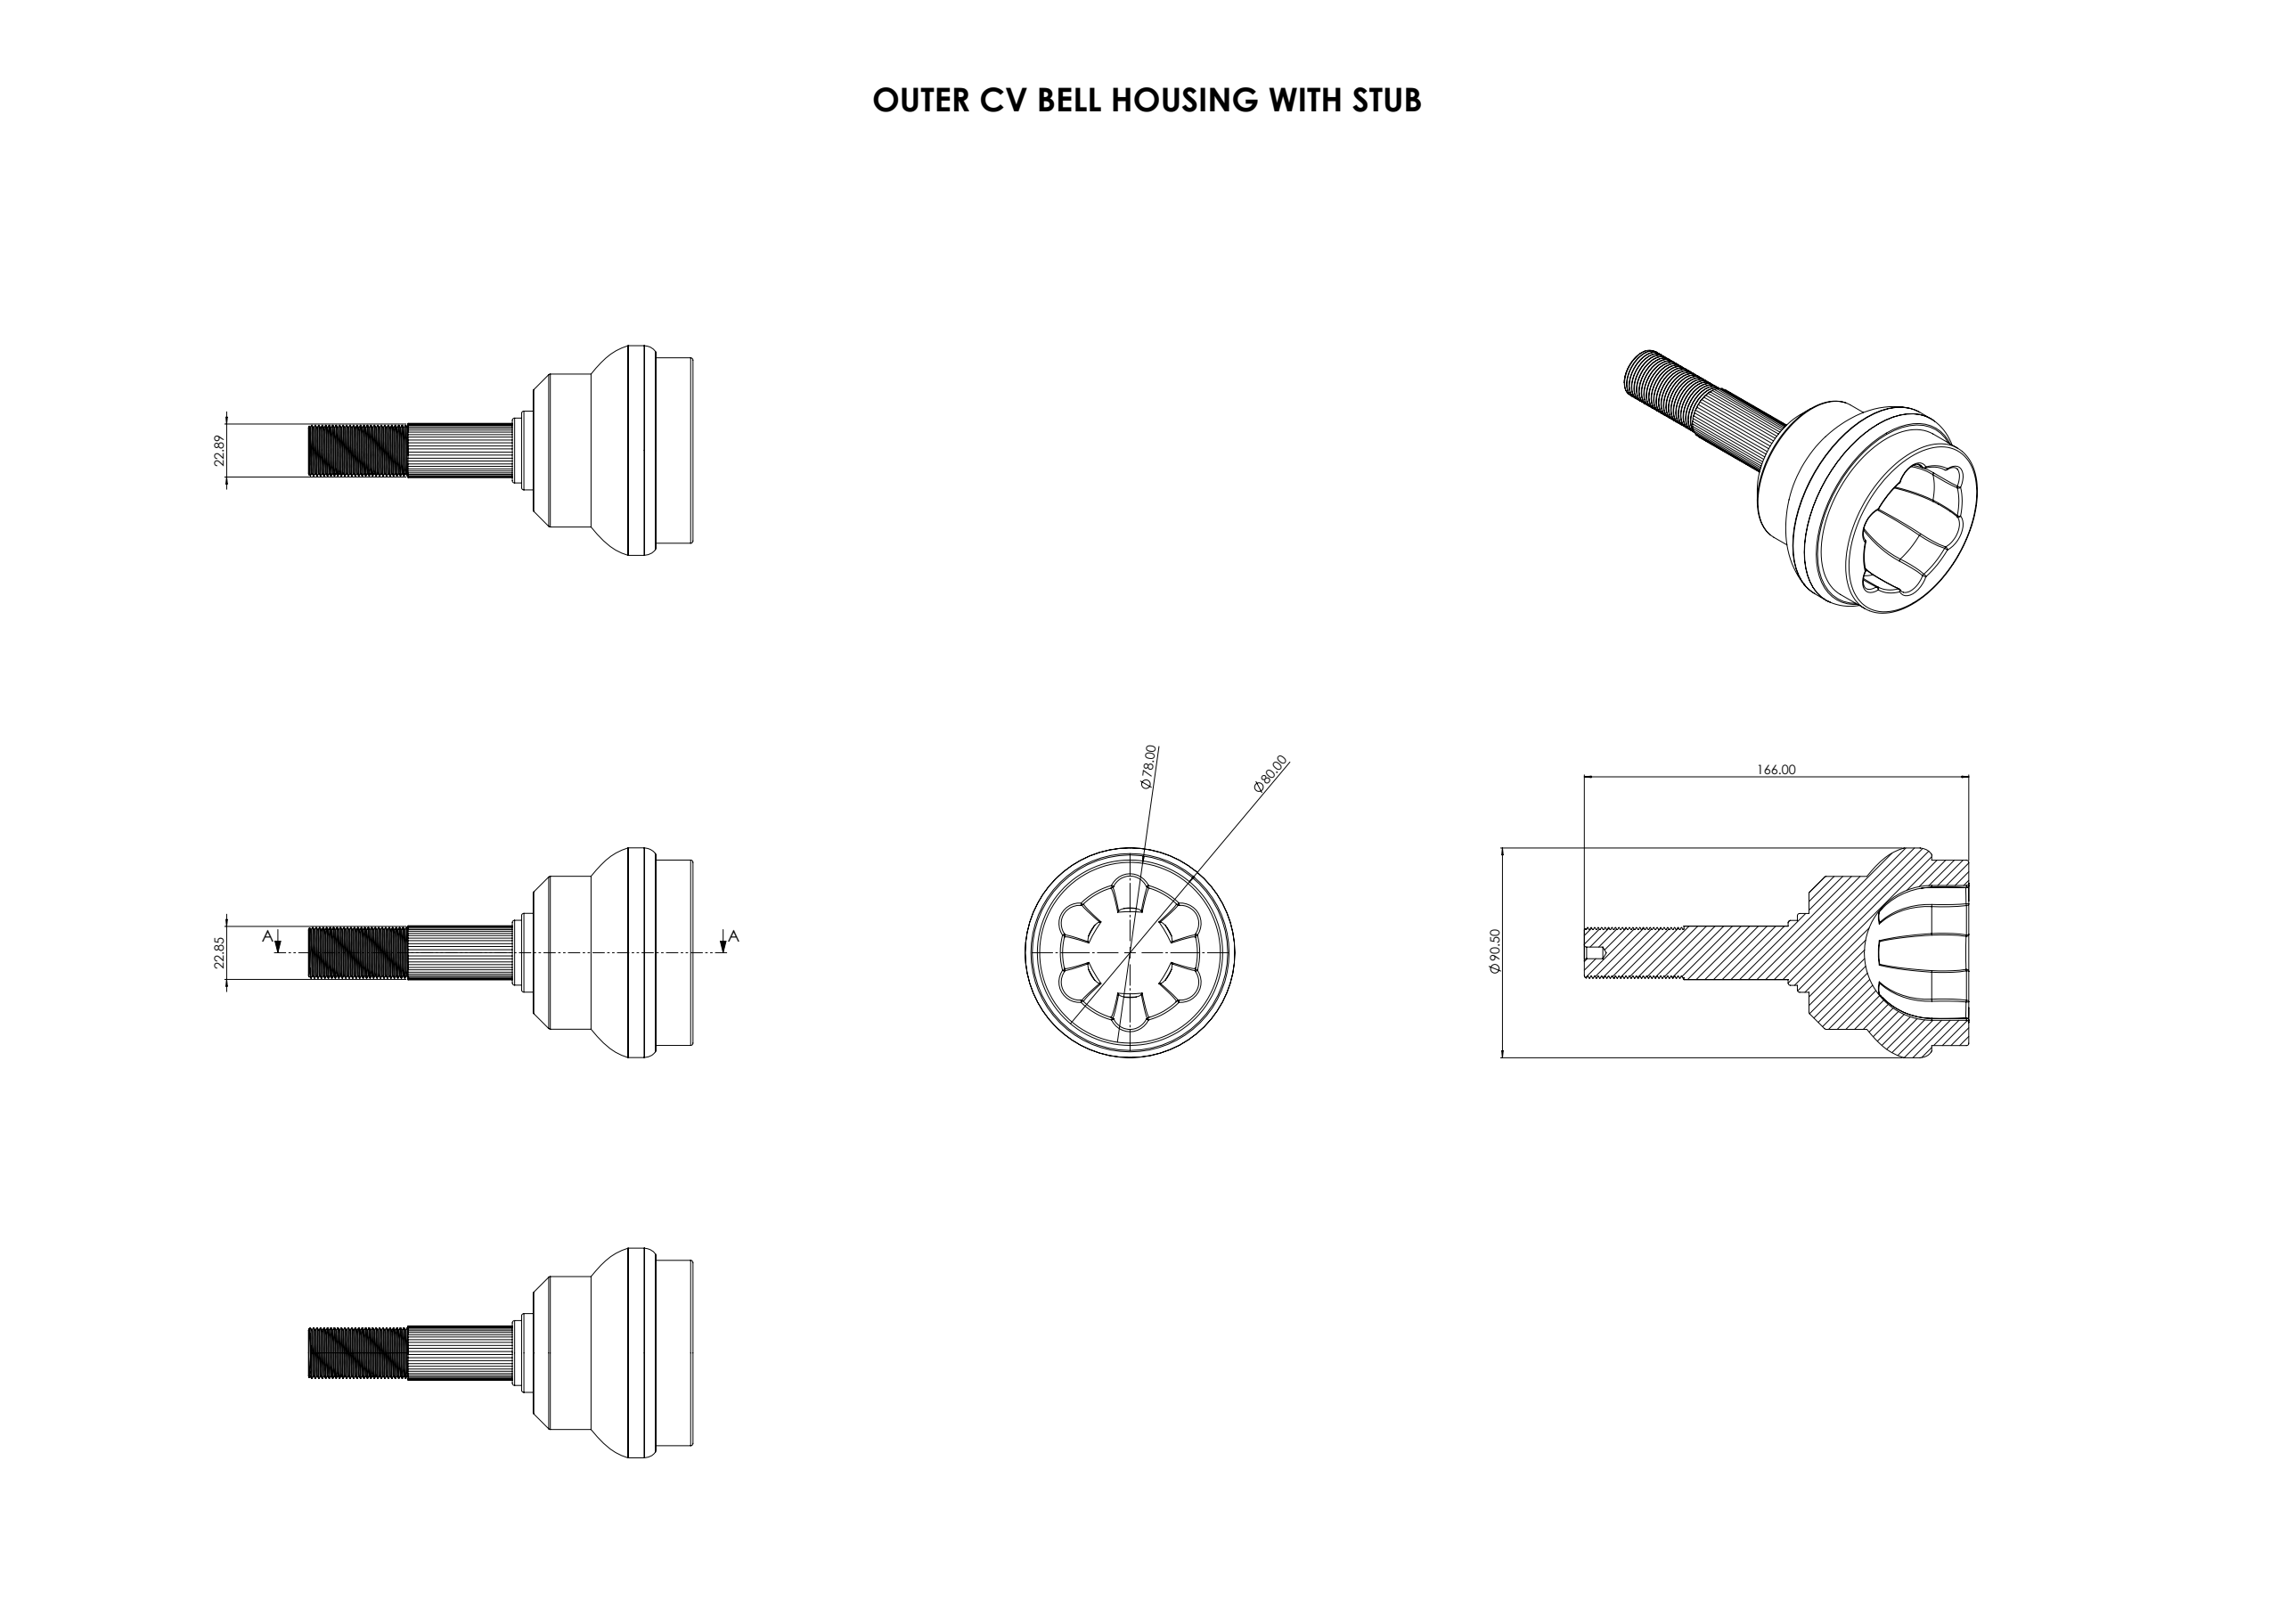
ISO-10303-21;
HEADER;
/* Generated by software containing ST-Developer
 * from STEP Tools, Inc. (www.steptools.com) 
 */

FILE_DESCRIPTION(
/* description */ (''),
/* implementation_level */ '2;1');

FILE_NAME(
/* name */ '01_Outer_CV_Bell_Housing_with_Stub.step',
/* time_stamp */ '2026-10-11T12:57:03-07:00',
/* author */ (''),
/* organization */ (''),
/* preprocessor_version */ 'ST-DEVELOPER v20.2',
/* originating_system */ 'Autodesk Translation Framework v15.15.0.0',
/* authorisation */ '');

FILE_SCHEMA (('AUTOMOTIVE_DESIGN { 1 0 10303 214 3 1 1 }'));
ENDSEC;

DATA;
#10=MECHANICAL_DESIGN_GEOMETRIC_PRESENTATION_REPRESENTATION('',(#256),#90374);
#222=SHAPE_REPRESENTATION_RELATIONSHIP('SRR','None',#90441,#239);
#239=ADVANCED_BREP_SHAPE_REPRESENTATION('',(#273),#90357);
#256=STYLED_ITEM('',(#90666),#273);
#273=MANIFOLD_SOLID_BREP('Body1',#40345);
#290=SPHERICAL_SURFACE('',#40682,1.);
#291=SPHERICAL_SURFACE('',#40693,1.);
#292=SPHERICAL_SURFACE('',#40696,1.);
#293=SPHERICAL_SURFACE('',#40706,1.);
#294=SPHERICAL_SURFACE('',#40722,1.);
#295=SPHERICAL_SURFACE('',#40737,1.);
#296=SPHERICAL_SURFACE('',#40746,1.);
#297=SPHERICAL_SURFACE('',#40754,1.);
#298=SPHERICAL_SURFACE('',#40760,1.);
#299=SPHERICAL_SURFACE('',#40771,1.);
#300=SPHERICAL_SURFACE('',#40778,1.);
#301=SPHERICAL_SURFACE('',#40783,1.);
#574=CONICAL_SURFACE('',#40627,29.5,0.785398163397447);
#575=CONICAL_SURFACE('',#40851,10.6,0.785398163397449);
#576=CONICAL_SURFACE('',#40869,2.5,1.03037682652431);
#781=TOROIDAL_SURFACE('',#40621,32.,1.);
#782=TOROIDAL_SURFACE('',#40631,25.5857864376269,1.);
#783=TOROIDAL_SURFACE('',#40636,16.,1.);
#784=TOROIDAL_SURFACE('',#40644,13.,1.);
#785=TOROIDAL_SURFACE('',#40685,26.4764045897475,8.05);
#786=TOROIDAL_SURFACE('',#40688,30.1,1.);
#787=TOROIDAL_SURFACE('',#40727,30.1,1.);
#788=TOROIDAL_SURFACE('',#40735,26.4764045897475,8.05);
#789=TOROIDAL_SURFACE('',#40740,30.1,1.);
#790=TOROIDAL_SURFACE('',#40748,26.4764045897475,8.05);
#791=TOROIDAL_SURFACE('',#40765,26.4764045897475,8.05);
#792=TOROIDAL_SURFACE('',#40766,30.1,1.);
#793=TOROIDAL_SURFACE('',#40773,26.4764045897475,8.05);
#794=TOROIDAL_SURFACE('',#40781,30.1,1.);
#795=TOROIDAL_SURFACE('',#40788,30.1,1.);
#796=TOROIDAL_SURFACE('',#40792,39.,1.);
#797=TOROIDAL_SURFACE('',#40849,9.925,1.);
#798=TOROIDAL_SURFACE('',#40857,9.78578643762691,1.);
#799=TOROIDAL_SURFACE('',#40863,3.5,1.);
#800=TOROIDAL_SURFACE('',#40899,26.4764045897475,8.05);
#1040=FACE_BOUND('',#4602,.T.);
#1041=FACE_BOUND('',#4612,.T.);
#1042=FACE_BOUND('',#4615,.T.);
#1043=FACE_BOUND('',#4619,.T.);
#1044=FACE_BOUND('',#4649,.T.);
#1045=FACE_BOUND('',#4695,.T.);
#1046=FACE_BOUND('',#4727,.T.);
#1116=PLANE('',#40614);
#1117=PLANE('',#40634);
#1118=PLANE('',#40641);
#1119=PLANE('',#40649);
#1120=PLANE('',#40678);
#1121=PLANE('',#40687);
#1122=PLANE('',#40729);
#1123=PLANE('',#40775);
#1124=PLANE('',#40799);
#1125=PLANE('',#40860);
#1126=PLANE('',#40870);
#1127=PLANE('',#40871);
#1128=PLANE('',#40872);
#1129=PLANE('',#40873);
#1130=PLANE('',#40874);
#1131=PLANE('',#40875);
#1132=PLANE('',#40876);
#1133=PLANE('',#40877);
#1134=PLANE('',#40878);
#1135=PLANE('',#40879);
#1136=PLANE('',#40880);
#1137=PLANE('',#40881);
#1138=PLANE('',#40882);
#1139=PLANE('',#40883);
#1140=PLANE('',#40884);
#1141=PLANE('',#40885);
#1142=PLANE('',#40886);
#1143=PLANE('',#40887);
#1144=PLANE('',#40888);
#1145=PLANE('',#40889);
#1146=PLANE('',#40890);
#1147=PLANE('',#40891);
#1148=PLANE('',#40892);
#1149=PLANE('',#40893);
#1150=PLANE('',#40894);
#1151=PLANE('',#40895);
#1152=PLANE('',#40896);
#1153=PLANE('',#40897);
#1154=PLANE('',#40901);
#1155=PLANE('',#40902);
#1828=(
BOUNDED_CURVE()
B_SPLINE_CURVE(5,(#61045,#61046,#61047,#61048,#61049,#61050,#61051,#61052,
#61053,#61054,#61055,#61056,#61057,#61058,#61059),.UNSPECIFIED.,.F.,.F.)
B_SPLINE_CURVE_WITH_KNOTS((6,1,1,1,1,1,1,1,1,1,6),(0.00785753170805376,
0.1,0.2,0.3,0.4,0.5,0.6,0.7,0.8,0.9,0.941278588050272),.UNSPECIFIED.)
CURVE()
GEOMETRIC_REPRESENTATION_ITEM()
RATIONAL_B_SPLINE_CURVE((1.,1.,1.,1.,1.,1.,1.,1.,1.,1.,1.,1.,1.,1.,1.))
REPRESENTATION_ITEM('')
);
#1829=(
BOUNDED_CURVE()
B_SPLINE_CURVE(5,(#61575,#61576,#61577,#61578,#61579,#61580,#61581,#61582,
#61583,#61584,#61585,#61586,#61587,#61588,#61589,#61590,#61591,#61592,#61593,
#61594),.UNSPECIFIED.,.F.,.F.)
B_SPLINE_CURVE_WITH_KNOTS((6,1,1,1,1,1,1,1,1,1,1,1,1,1,1,6),(0.,0.0666666666666667,
0.133333333333333,0.2,0.266666666666667,0.333333333333333,0.4,0.466666666666667,
0.533333333333333,0.6,0.666666666666667,0.733333333333333,0.8,0.866666666666667,
0.933333333333333,0.992729019266749),.UNSPECIFIED.)
CURVE()
GEOMETRIC_REPRESENTATION_ITEM()
RATIONAL_B_SPLINE_CURVE((1.,1.,1.,1.,1.,1.,1.,1.,1.,1.,1.,1.,1.,1.,1.,1.,
1.,1.,1.,1.))
REPRESENTATION_ITEM('')
);
#1931=(
BOUNDED_SURFACE()
B_SPLINE_SURFACE(5,2,((#60909,#60910,#60911,#60912,#60913,#60914,#60915,
#60916,#60917),(#60918,#60919,#60920,#60921,#60922,#60923,#60924,#60925,
#60926),(#60927,#60928,#60929,#60930,#60931,#60932,#60933,#60934,#60935),
(#60936,#60937,#60938,#60939,#60940,#60941,#60942,#60943,#60944),(#60945,
#60946,#60947,#60948,#60949,#60950,#60951,#60952,#60953),(#60954,#60955,
#60956,#60957,#60958,#60959,#60960,#60961,#60962),(#60963,#60964,#60965,
#60966,#60967,#60968,#60969,#60970,#60971),(#60972,#60973,#60974,#60975,
#60976,#60977,#60978,#60979,#60980),(#60981,#60982,#60983,#60984,#60985,
#60986,#60987,#60988,#60989),(#60990,#60991,#60992,#60993,#60994,#60995,
#60996,#60997,#60998),(#60999,#61000,#61001,#61002,#61003,#61004,#61005,
#61006,#61007),(#61008,#61009,#61010,#61011,#61012,#61013,#61014,#61015,
#61016),(#61017,#61018,#61019,#61020,#61021,#61022,#61023,#61024,#61025),
(#61026,#61027,#61028,#61029,#61030,#61031,#61032,#61033,#61034),(#61035,
#61036,#61037,#61038,#61039,#61040,#61041,#61042,#61043)),.UNSPECIFIED.,
 .F.,.T.,.F.)
B_SPLINE_SURFACE_WITH_KNOTS((6,1,1,1,1,1,1,1,1,1,6),(3,2,2,2,3),(-1.,-0.9,
-0.8,-0.7,-0.6,-0.5,-0.4,-0.3,-0.2,-0.1,0.),(0.,1.5707963267949,3.14159265358979,
4.71238898038469,6.28318530717959),.UNSPECIFIED.)
GEOMETRIC_REPRESENTATION_ITEM()
RATIONAL_B_SPLINE_SURFACE(((1.,0.707106781186548,1.,0.707106781186548,1.,
0.707106781186548,1.,0.707106781186548,1.),(1.,0.707106781186548,1.,0.707106781186548,
1.,0.707106781186548,1.,0.707106781186548,1.),(1.,0.707106781186548,1.,
0.707106781186548,1.,0.707106781186548,1.,0.707106781186548,1.),(1.,0.707106781186548,
1.,0.707106781186548,1.,0.707106781186548,1.,0.707106781186548,1.),(1.,
0.707106781186548,1.,0.707106781186548,1.,0.707106781186548,1.,0.707106781186548,
1.),(1.,0.707106781186548,1.,0.707106781186548,1.,0.707106781186548,1.,
0.707106781186548,1.),(1.,0.707106781186548,1.,0.707106781186548,1.,0.707106781186548,
1.,0.707106781186548,1.),(1.,0.707106781186548,1.,0.707106781186548,1.,
0.707106781186548,1.,0.707106781186548,1.),(1.,0.707106781186548,1.,0.707106781186548,
1.,0.707106781186548,1.,0.707106781186548,1.),(1.,0.707106781186548,1.,
0.707106781186548,1.,0.707106781186548,1.,0.707106781186548,1.),(1.,0.707106781186548,
1.,0.707106781186548,1.,0.707106781186548,1.,0.707106781186548,1.),(1.,
0.707106781186548,1.,0.707106781186548,1.,0.707106781186548,1.,0.707106781186548,
1.),(1.,0.707106781186548,1.,0.707106781186548,1.,0.707106781186548,1.,
0.707106781186548,1.),(1.,0.707106781186548,1.,0.707106781186548,1.,0.707106781186548,
1.,0.707106781186548,1.),(1.,0.707106781186548,1.,0.707106781186548,1.,
0.707106781186548,1.,0.707106781186548,1.)))
REPRESENTATION_ITEM('')
SURFACE()
);
#1932=(
BOUNDED_SURFACE()
B_SPLINE_SURFACE(5,2,((#61394,#61395,#61396,#61397,#61398,#61399,#61400,
#61401,#61402),(#61403,#61404,#61405,#61406,#61407,#61408,#61409,#61410,
#61411),(#61412,#61413,#61414,#61415,#61416,#61417,#61418,#61419,#61420),
(#61421,#61422,#61423,#61424,#61425,#61426,#61427,#61428,#61429),(#61430,
#61431,#61432,#61433,#61434,#61435,#61436,#61437,#61438),(#61439,#61440,
#61441,#61442,#61443,#61444,#61445,#61446,#61447),(#61448,#61449,#61450,
#61451,#61452,#61453,#61454,#61455,#61456),(#61457,#61458,#61459,#61460,
#61461,#61462,#61463,#61464,#61465),(#61466,#61467,#61468,#61469,#61470,
#61471,#61472,#61473,#61474),(#61475,#61476,#61477,#61478,#61479,#61480,
#61481,#61482,#61483),(#61484,#61485,#61486,#61487,#61488,#61489,#61490,
#61491,#61492),(#61493,#61494,#61495,#61496,#61497,#61498,#61499,#61500,
#61501),(#61502,#61503,#61504,#61505,#61506,#61507,#61508,#61509,#61510),
(#61511,#61512,#61513,#61514,#61515,#61516,#61517,#61518,#61519),(#61520,
#61521,#61522,#61523,#61524,#61525,#61526,#61527,#61528),(#61529,#61530,
#61531,#61532,#61533,#61534,#61535,#61536,#61537),(#61538,#61539,#61540,
#61541,#61542,#61543,#61544,#61545,#61546),(#61547,#61548,#61549,#61550,
#61551,#61552,#61553,#61554,#61555),(#61556,#61557,#61558,#61559,#61560,
#61561,#61562,#61563,#61564),(#61565,#61566,#61567,#61568,#61569,#61570,
#61571,#61572,#61573)),.UNSPECIFIED.,.F.,.T.,.F.)
B_SPLINE_SURFACE_WITH_KNOTS((6,1,1,1,1,1,1,1,1,1,1,1,1,1,1,6),(3,2,2,2,
3),(-1.,-0.933333333333333,-0.866666666666667,-0.8,-0.733333333333333,-0.666666666666667,
-0.6,-0.533333333333333,-0.466666666666667,-0.4,-0.333333333333333,-0.266666666666667,
-0.2,-0.133333333333333,-0.0666666666666667,0.),(0.,1.5707963267949,3.14159265358979,
4.71238898038469,6.28318530717959),.UNSPECIFIED.)
GEOMETRIC_REPRESENTATION_ITEM()
RATIONAL_B_SPLINE_SURFACE(((1.,0.707106781186548,1.,0.707106781186548,1.,
0.707106781186548,1.,0.707106781186548,1.),(1.,0.707106781186548,1.,0.707106781186548,
1.,0.707106781186548,1.,0.707106781186548,1.),(1.,0.707106781186548,1.,
0.707106781186548,1.,0.707106781186548,1.,0.707106781186548,1.),(1.,0.707106781186548,
1.,0.707106781186548,1.,0.707106781186548,1.,0.707106781186548,1.),(1.,
0.707106781186548,1.,0.707106781186548,1.,0.707106781186548,1.,0.707106781186548,
1.),(1.,0.707106781186548,1.,0.707106781186548,1.,0.707106781186548,1.,
0.707106781186548,1.),(1.,0.707106781186548,1.,0.707106781186548,1.,0.707106781186548,
1.,0.707106781186548,1.),(1.,0.707106781186548,1.,0.707106781186548,1.,
0.707106781186548,1.,0.707106781186548,1.),(1.,0.707106781186548,1.,0.707106781186548,
1.,0.707106781186548,1.,0.707106781186548,1.),(1.,0.707106781186548,1.,
0.707106781186548,1.,0.707106781186548,1.,0.707106781186548,1.),(1.,0.707106781186548,
1.,0.707106781186548,1.,0.707106781186548,1.,0.707106781186548,1.),(1.,
0.707106781186548,1.,0.707106781186548,1.,0.707106781186548,1.,0.707106781186548,
1.),(1.,0.707106781186548,1.,0.707106781186548,1.,0.707106781186548,1.,
0.707106781186548,1.),(1.,0.707106781186548,1.,0.707106781186548,1.,0.707106781186548,
1.,0.707106781186548,1.),(1.,0.707106781186548,1.,0.707106781186548,1.,
0.707106781186548,1.,0.707106781186548,1.),(1.,0.707106781186548,1.,0.707106781186548,
1.,0.707106781186548,1.,0.707106781186548,1.),(1.,0.707106781186548,1.,
0.707106781186548,1.,0.707106781186548,1.,0.707106781186548,1.),(1.,0.707106781186548,
1.,0.707106781186548,1.,0.707106781186548,1.,0.707106781186548,1.),(1.,
0.707106781186548,1.,0.707106781186548,1.,0.707106781186548,1.,0.707106781186548,
1.),(1.,0.707106781186548,1.,0.707106781186548,1.,0.707106781186548,1.,
0.707106781186548,1.)))
REPRESENTATION_ITEM('')
SURFACE()
);
#1933=(
BOUNDED_SURFACE()
B_SPLINE_SURFACE(2,2,((#62249,#62250,#62251,#62252,#62253,#62254,#62255,
#62256,#62257),(#62258,#62259,#62260,#62261,#62262,#62263,#62264,#62265,
#62266),(#62267,#62268,#62269,#62270,#62271,#62272,#62273,#62274,#62275)),
 .UNSPECIFIED.,.F.,.T.,.F.)
B_SPLINE_SURFACE_WITH_KNOTS((3,3),(3,2,2,2,3),(-1.5707731742648,-2.31493893392376E-5),
(-3.14159265358979,-1.5707963267949,0.,1.5707963267949,3.14159265358979),
 .UNSPECIFIED.)
GEOMETRIC_REPRESENTATION_ITEM()
RATIONAL_B_SPLINE_SURFACE(((1.,0.707106781186548,1.,0.707106781186548,1.,
0.707106781186548,1.,0.707106781186548,1.),(0.707123151197659,0.500011575345865,
0.707123151197659,0.500011575345865,0.707123151197659,0.500011575345865,
0.707123151197659,0.500011575345865,0.707123151197659),(1.,0.707106781186548,
1.,0.707106781186548,1.,0.707106781186548,1.,0.707106781186548,1.)))
REPRESENTATION_ITEM('')
SURFACE()
);
#1938=B_SPLINE_SURFACE_WITH_KNOTS('',3,3,((#60774,#60775,#60776,#60777,
#60778,#60779,#60780,#60781,#60782,#60783,#60784,#60785,#60786,#60787,#60788,
#60789,#60790,#60791,#60792,#60793,#60794,#60795),(#60796,#60797,#60798,
#60799,#60800,#60801,#60802,#60803,#60804,#60805,#60806,#60807,#60808,#60809,
#60810,#60811,#60812,#60813,#60814,#60815,#60816,#60817),(#60818,#60819,
#60820,#60821,#60822,#60823,#60824,#60825,#60826,#60827,#60828,#60829,#60830,
#60831,#60832,#60833,#60834,#60835,#60836,#60837,#60838,#60839),(#60840,
#60841,#60842,#60843,#60844,#60845,#60846,#60847,#60848,#60849,#60850,#60851,
#60852,#60853,#60854,#60855,#60856,#60857,#60858,#60859,#60860,#60861)),
 .UNSPECIFIED.,.F.,.T.,.F.,(4,4),(4,1,1,1,1,1,1,1,1,1,1,1,1,1,1,1,1,1,1,
4),(0.,1.),(1.5707963267949,2.01959527730772,2.46839422782055,2.76759352816244,
3.06679282850432,3.36599212884621,3.66519142918809,3.96439072952998,4.26359002987186,
4.56278933021375,4.86198863055563,5.16118793089752,5.4603872312394,5.75958653158129,
6.05878583192317,6.20838548209412,6.35798513226506,6.95638373294883,7.40518268346166,
7.85398163397448),.UNSPECIFIED.);
#1939=B_SPLINE_SURFACE_WITH_KNOTS('',3,3,((#61124,#61125,#61126,#61127,
#61128,#61129,#61130,#61131,#61132,#61133,#61134,#61135,#61136,#61137,#61138,
#61139,#61140,#61141,#61142,#61143,#61144,#61145,#61146),(#61147,#61148,
#61149,#61150,#61151,#61152,#61153,#61154,#61155,#61156,#61157,#61158,#61159,
#61160,#61161,#61162,#61163,#61164,#61165,#61166,#61167,#61168,#61169),
(#61170,#61171,#61172,#61173,#61174,#61175,#61176,#61177,#61178,#61179,
#61180,#61181,#61182,#61183,#61184,#61185,#61186,#61187,#61188,#61189,#61190,
#61191,#61192),(#61193,#61194,#61195,#61196,#61197,#61198,#61199,#61200,
#61201,#61202,#61203,#61204,#61205,#61206,#61207,#61208,#61209,#61210,#61211,
#61212,#61213,#61214,#61215)),.UNSPECIFIED.,.F.,.T.,.F.,(4,4),(4,1,1,1,
1,1,1,1,1,1,1,1,1,1,1,1,1,1,1,1,4),(0.,1.),(1.5707963267949,2.01959527730772,
2.46839422782055,2.76759352816244,3.06679282850432,3.36599212884621,3.66519142918809,
3.96439072952998,4.26359002987186,4.56278933021375,4.86198863055563,5.16118793089752,
5.4603872312394,5.75958653158129,6.05878583192317,6.20838548209412,6.35798513226506,
6.65718443260694,6.95638373294883,7.40518268346166,7.85398163397448),
 .UNSPECIFIED.);
#1940=B_SPLINE_SURFACE_WITH_KNOTS('',3,3,((#61277,#61278,#61279,#61280,
#61281,#61282,#61283,#61284,#61285,#61286,#61287,#61288,#61289,#61290,#61291,
#61292,#61293,#61294,#61295,#61296,#61297,#61298,#61299),(#61300,#61301,
#61302,#61303,#61304,#61305,#61306,#61307,#61308,#61309,#61310,#61311,#61312,
#61313,#61314,#61315,#61316,#61317,#61318,#61319,#61320,#61321,#61322),
(#61323,#61324,#61325,#61326,#61327,#61328,#61329,#61330,#61331,#61332,
#61333,#61334,#61335,#61336,#61337,#61338,#61339,#61340,#61341,#61342,#61343,
#61344,#61345),(#61346,#61347,#61348,#61349,#61350,#61351,#61352,#61353,
#61354,#61355,#61356,#61357,#61358,#61359,#61360,#61361,#61362,#61363,#61364,
#61365,#61366,#61367,#61368)),.UNSPECIFIED.,.F.,.T.,.F.,(4,4),(4,1,1,1,
1,1,1,1,1,1,1,1,1,1,1,1,1,1,1,1,4),(0.,1.),(1.5707963267949,2.01959527730772,
2.46839422782055,2.76759352816244,3.06679282850432,3.36599212884621,3.66519142918809,
3.96439072952998,4.26359002987186,4.56278933021375,4.86198863055563,5.16118793089752,
5.4603872312394,5.75958653158129,6.05878583192317,6.20838548209412,6.35798513226506,
6.65718443260694,6.95638373294883,7.40518268346166,7.85398163397448),
 .UNSPECIFIED.);
#1941=B_SPLINE_SURFACE_WITH_KNOTS('',3,3,((#61755,#61756,#61757,#61758),
(#61759,#61760,#61761,#61762),(#61763,#61764,#61765,#61766),(#61767,#61768,
#61769,#61770),(#61771,#61772,#61773,#61774)),.UNSPECIFIED.,.F.,.F.,.F.,
(4,1,4),(4,4),(0.,0.571428571428571,1.),(4.17539678580906,5.27137424194997),
 .UNSPECIFIED.);
#1942=B_SPLINE_SURFACE_WITH_KNOTS('',3,3,((#61821,#61822,#61823,#61824),
(#61825,#61826,#61827,#61828),(#61829,#61830,#61831,#61832),(#61833,#61834,
#61835,#61836),(#61837,#61838,#61839,#61840)),.UNSPECIFIED.,.F.,.F.,.F.,
(4,1,4),(4,4),(0.,0.571428571428571,1.),(4.17538600473639,5.27136346380212),
 .UNSPECIFIED.);
#1943=B_SPLINE_SURFACE_WITH_KNOTS('',3,3,((#61885,#61886,#61887,#61888,
#61889),(#61890,#61891,#61892,#61893,#61894),(#61895,#61896,#61897,#61898,
#61899),(#61900,#61901,#61902,#61903,#61904)),.UNSPECIFIED.,.F.,.F.,.F.,
(4,4),(4,1,4),(0.,1.),(8.38443833695044,9.5374231246245,11.0747361748566),
 .UNSPECIFIED.);
#1944=B_SPLINE_SURFACE_WITH_KNOTS('',3,3,((#61923,#61924,#61925,#61926,
#61927,#61928),(#61929,#61930,#61931,#61932,#61933,#61934),(#61935,#61936,
#61937,#61938,#61939,#61940),(#61941,#61942,#61943,#61944,#61945,#61946)),
 .UNSPECIFIED.,.F.,.F.,.F.,(4,4),(4,1,1,4),(0.,1.),(-2.31999627410953E-6,
0.644940971614267,1.07490316602129,1.50486536042832),.UNSPECIFIED.);
#1945=B_SPLINE_SURFACE_WITH_KNOTS('',3,3,((#62010,#62011,#62012,#62013,
#62014,#62015,#62016),(#62017,#62018,#62019,#62020,#62021,#62022,#62023),
(#62024,#62025,#62026,#62027,#62028,#62029,#62030),(#62031,#62032,#62033,
#62034,#62035,#62036,#62037),(#62038,#62039,#62040,#62041,#62042,#62043,
#62044),(#62045,#62046,#62047,#62048,#62049,#62050,#62051)),
 .UNSPECIFIED.,.F.,.F.,.F.,(4,1,1,4),(4,1,1,1,4),(0.,0.285714285714286,
0.571428571428571,1.),(3.95106839817899,4.52186525716006,4.8072636866506,
5.37806054563167,5.94885740461274),.UNSPECIFIED.);
#1946=B_SPLINE_SURFACE_WITH_KNOTS('',3,3,((#62135,#62136,#62137,#62138,
#62139,#62140),(#62141,#62142,#62143,#62144,#62145,#62146),(#62147,#62148,
#62149,#62150,#62151,#62152),(#62153,#62154,#62155,#62156,#62157,#62158)),
 .UNSPECIFIED.,.F.,.F.,.F.,(4,4),(4,1,1,4),(0.,1.),(-2.31999627050912E-6,
0.430022123191898,0.860046566380066,1.50508323116232),.UNSPECIFIED.);
#1947=B_SPLINE_SURFACE_WITH_KNOTS('',3,3,((#62182,#62183,#62184,#62185,
#62186),(#62187,#62188,#62189,#62190,#62191),(#62192,#62193,#62194,#62195,
#62196),(#62197,#62198,#62199,#62200,#62201)),.UNSPECIFIED.,.F.,.F.,.F.,
(4,4),(4,1,4),(0.,1.),(0.,0.644978914561078,1.50495080064252),
 .UNSPECIFIED.);
#1948=B_SPLINE_SURFACE_WITH_KNOTS('',3,3,((#62213,#62214,#62215,#62216,
#62217),(#62218,#62219,#62220,#62221,#62222),(#62223,#62224,#62225,#62226,
#62227),(#62228,#62229,#62230,#62231,#62232)),.UNSPECIFIED.,.F.,.F.,.F.,
(4,4),(4,1,4),(0.,1.),(-2.31999443863861E-6,1.15298346196168,2.69029783790316),
 .UNSPECIFIED.);
#1949=B_SPLINE_SURFACE_WITH_KNOTS('',3,3,((#62392,#62393,#62394,#62395),
(#62396,#62397,#62398,#62399),(#62400,#62401,#62402,#62403),(#62404,#62405,
#62406,#62407),(#62408,#62409,#62410,#62411)),.UNSPECIFIED.,.F.,.F.,.F.,
(4,1,4),(4,4),(0.,0.571428571428571,1.),(4.17539678580906,5.27137424194994),
 .UNSPECIFIED.);
#1950=B_SPLINE_SURFACE_WITH_KNOTS('',3,3,((#62452,#62453,#62454,#62455,
#62456,#62457,#62458),(#62459,#62460,#62461,#62462,#62463,#62464,#62465),
(#62466,#62467,#62468,#62469,#62470,#62471,#62472),(#62473,#62474,#62475,
#62476,#62477,#62478,#62479),(#62480,#62481,#62482,#62483,#62484,#62485,
#62486),(#62487,#62488,#62489,#62490,#62491,#62492,#62493)),
 .UNSPECIFIED.,.F.,.F.,.F.,(4,1,1,4),(4,1,1,1,4),(0.,0.285714285714286,
0.571428571428571,1.),(5.94885740461274,6.5196542639437,6.80505269360918,
7.37584955294014,7.9466464122711),.UNSPECIFIED.);
#1951=B_SPLINE_SURFACE_WITH_KNOTS('',3,3,((#62577,#62578,#62579,#62580,
#62581),(#62582,#62583,#62584,#62585,#62586),(#62587,#62588,#62589,#62590,
#62591),(#62592,#62593,#62594,#62595,#62596)),.UNSPECIFIED.,.F.,.F.,.F.,
(4,4),(4,1,4),(0.,1.),(0.206729096402498,0.851718551084393,1.71170449066025),
 .UNSPECIFIED.);
#1952=B_SPLINE_SURFACE_WITH_KNOTS('',3,3,((#62604,#62605,#62606,#62607,
#62608),(#62609,#62610,#62611,#62612,#62613),(#62614,#62615,#62616,#62617,
#62618),(#62619,#62620,#62621,#62622,#62623)),.UNSPECIFIED.,.F.,.F.,.F.,
(4,4),(4,1,4),(0.,1.),(-2.31999444043195E-6,1.15298346125989,2.69029783626566),
 .UNSPECIFIED.);
#1953=B_SPLINE_SURFACE_WITH_KNOTS('',3,3,((#62634,#62635,#62636,#62637,
#62638),(#62639,#62640,#62641,#62642,#62643),(#62644,#62645,#62646,#62647,
#62648),(#62649,#62650,#62651,#62652,#62653)),.UNSPECIFIED.,.F.,.F.,.F.,
(4,4),(4,1,4),(0.,1.),(8.52932428183543,9.68230906880774,11.2196221181042),
 .UNSPECIFIED.);
#1954=B_SPLINE_SURFACE_WITH_KNOTS('',3,3,((#62666,#62667,#62668,#62669,
#62670),(#62671,#62672,#62673,#62674,#62675),(#62676,#62677,#62678,#62679,
#62680),(#62681,#62682,#62683,#62684,#62685)),.UNSPECIFIED.,.F.,.F.,.F.,
(4,4),(4,1,4),(0.,1.),(-2.31999627648449E-6,0.85992278978735,1.50486662212507),
 .UNSPECIFIED.);
#1955=B_SPLINE_SURFACE_WITH_KNOTS('',3,3,((#63057,#63058,#63059,#63060),
(#63061,#63062,#63063,#63064),(#63065,#63066,#63067,#63068),(#63069,#63070,
#63071,#63072),(#63073,#63074,#63075,#63076)),.UNSPECIFIED.,.F.,.F.,.F.,
(4,1,4),(4,4),(0.,0.571428571428571,1.),(4.17533133480784,5.27130879387958),
 .UNSPECIFIED.);
#1956=B_SPLINE_SURFACE_WITH_KNOTS('',3,3,((#63115,#63116,#63117,#63118,
#63119),(#63120,#63121,#63122,#63123,#63124),(#63125,#63126,#63127,#63128,
#63129),(#63130,#63131,#63132,#63133,#63134)),.UNSPECIFIED.,.F.,.F.,.F.,
(4,4),(4,1,4),(0.,1.),(8.52985716994968,9.68284195691921,11.2201550062119),
 .UNSPECIFIED.);
#1957=B_SPLINE_SURFACE_WITH_KNOTS('',3,3,((#63153,#63154,#63155,#63156,
#63157,#63158),(#63159,#63160,#63161,#63162,#63163,#63164),(#63165,#63166,
#63167,#63168,#63169,#63170),(#63171,#63172,#63173,#63174,#63175,#63176)),
 .UNSPECIFIED.,.F.,.F.,.F.,(4,4),(4,1,1,4),(0.,1.),(0.207327684708445,0.637351476682114,
1.06737526865578,1.71241095661629),.UNSPECIFIED.);
#1958=B_SPLINE_SURFACE_WITH_KNOTS('',3,3,((#63191,#63192,#63193,#63194,
#63195),(#63196,#63197,#63198,#63199,#63200),(#63201,#63202,#63203,#63204,
#63205),(#63206,#63207,#63208,#63209,#63210)),.UNSPECIFIED.,.F.,.F.,.F.,
(4,4),(4,1,4),(0.,1.),(-2.31999443730624E-6,1.15298346125614,2.69029783625691),
 .UNSPECIFIED.);
#1959=B_SPLINE_SURFACE_WITH_KNOTS('',3,3,((#63221,#63222,#63223,#63224,
#63225,#63226),(#63227,#63228,#63229,#63230,#63231,#63232),(#63233,#63234,
#63235,#63236,#63237,#63238),(#63239,#63240,#63241,#63242,#63243,#63244)),
 .UNSPECIFIED.,.F.,.F.,.F.,(4,4),(4,1,1,4),(0.,1.),(0.,0.644950465905299,
1.0749174431755,1.5048844204457),.UNSPECIFIED.);
#1960=B_SPLINE_SURFACE_WITH_KNOTS('',3,3,((#63261,#63262,#63263,#63264,
#63265),(#63266,#63267,#63268,#63269,#63270),(#63271,#63272,#63273,#63274,
#63275),(#63276,#63277,#63278,#63279,#63280)),.UNSPECIFIED.,.F.,.F.,.F.,
(4,4),(4,1,4),(0.,1.),(-2.3199944317628E-6,1.15298346196206,2.69029783790404),
 .UNSPECIFIED.);
#1961=B_SPLINE_SURFACE_WITH_KNOTS('',3,3,((#63297,#63298,#63299,#63300,
#63301,#63302,#63303),(#63304,#63305,#63306,#63307,#63308,#63309,#63310),
(#63311,#63312,#63313,#63314,#63315,#63316,#63317),(#63318,#63319,#63320,
#63321,#63322,#63323,#63324),(#63325,#63326,#63327,#63328,#63329,#63330,
#63331),(#63332,#63333,#63334,#63335,#63336,#63337,#63338)),
 .UNSPECIFIED.,.F.,.F.,.F.,(4,1,1,4),(4,1,1,1,4),(0.,0.285714285714286,
0.571428571428571,1.),(4.94996091805913,5.2353622298247,5.80616485335585,
6.37696747688699,6.94777010041813),.UNSPECIFIED.);
#1962=B_SPLINE_SURFACE_WITH_KNOTS('',3,3,((#63348,#63349,#63350,#63351,
#63352),(#63353,#63354,#63355,#63356,#63357),(#63358,#63359,#63360,#63361,
#63362),(#63363,#63364,#63365,#63366,#63367)),.UNSPECIFIED.,.F.,.F.,.F.,
(4,4),(4,1,4),(0.,1.),(0.,0.85997188017068,1.50495079029869),
 .UNSPECIFIED.);
#1963=B_SPLINE_SURFACE_WITH_KNOTS('',3,3,((#63390,#63391,#63392,#63393,
#63394),(#63395,#63396,#63397,#63398,#63399),(#63400,#63401,#63402,#63403,
#63404),(#63405,#63406,#63407,#63408,#63409)),.UNSPECIFIED.,.F.,.F.,.F.,
(4,4),(4,1,4),(0.,1.),(8.38443833694999,9.92175271289341,11.074738494851),
 .UNSPECIFIED.);
#1964=B_SPLINE_SURFACE_WITH_KNOTS('',3,3,((#63434,#63435,#63436,#63437,
#63438),(#63439,#63440,#63441,#63442,#63443),(#63444,#63445,#63446,#63447,
#63448),(#63449,#63450,#63451,#63452,#63453)),.UNSPECIFIED.,.F.,.F.,.F.,
(4,4),(4,1,4),(0.,1.),(0.,0.644951640555328,1.50488716129577),
 .UNSPECIFIED.);
#1965=B_SPLINE_SURFACE_WITH_KNOTS('',3,3,((#63466,#63467,#63468,#63469,
#63470),(#63471,#63472,#63473,#63474,#63475),(#63476,#63477,#63478,#63479,
#63480),(#63481,#63482,#63483,#63484,#63485)),.UNSPECIFIED.,.F.,.F.,.F.,
(4,4),(4,1,4),(0.,1.),(-2.31999443914823E-6,1.15298346196168,2.69029783790317),
 .UNSPECIFIED.);
#1966=B_SPLINE_SURFACE_WITH_KNOTS('',3,3,((#63504,#63505,#63506,#63507,
#63508,#63509,#63510),(#63511,#63512,#63513,#63514,#63515,#63516,#63517),
(#63518,#63519,#63520,#63521,#63522,#63523,#63524),(#63525,#63526,#63527,
#63528,#63529,#63530,#63531),(#63532,#63533,#63534,#63535,#63536,#63537,
#63538),(#63539,#63540,#63541,#63542,#63543,#63544,#63545)),
 .UNSPECIFIED.,.F.,.F.,.F.,(4,1,1,4),(4,1,1,1,4),(0.,0.285714285714286,
0.571428571428571,1.),(4.94996091806794,5.52076354159657,6.09156616512519,
6.37696747688951,6.94777010041813),.UNSPECIFIED.);
#1967=B_SPLINE_SURFACE_WITH_KNOTS('',3,3,((#63550,#63551,#63552,#63553),
(#63554,#63555,#63556,#63557),(#63558,#63559,#63560,#63561),(#63562,#63563,
#63564,#63565),(#63566,#63567,#63568,#63569)),.UNSPECIFIED.,.F.,.F.,.F.,
(4,1,4),(4,4),(0.,0.571428571428571,1.),(4.17531192673851,5.2712893858124),
 .UNSPECIFIED.);
#1968=B_SPLINE_SURFACE_WITH_KNOTS('',3,3,((#63608,#63609,#63610,#63611,
#63612),(#63613,#63614,#63615,#63616,#63617),(#63618,#63619,#63620,#63621,
#63622),(#63623,#63624,#63625,#63626,#63627)),.UNSPECIFIED.,.F.,.F.,.F.,
(4,4),(4,1,4),(0.,1.),(8.38443833695038,9.53742312462444,11.0747361748565),
 .UNSPECIFIED.);
#1969=B_SPLINE_SURFACE_WITH_KNOTS('',3,3,((#63640,#63641,#63642,#63643,
#63644,#63645),(#63646,#63647,#63648,#63649,#63650,#63651),(#63652,#63653,
#63654,#63655,#63656,#63657),(#63658,#63659,#63660,#63661,#63662,#63663)),
 .UNSPECIFIED.,.F.,.F.,.F.,(4,4),(4,1,1,4),(0.,1.),(-2.3199962741138E-6,
0.644939523401962,1.07490075233412,1.50486198126628),.UNSPECIFIED.);
#1970=B_SPLINE_SURFACE_WITH_KNOTS('',3,3,((#63708,#63709,#63710,#63711,
#63712,#63713),(#63714,#63715,#63716,#63717,#63718,#63719),(#63720,#63721,
#63722,#63723,#63724,#63725),(#63726,#63727,#63728,#63729,#63730,#63731)),
 .UNSPECIFIED.,.F.,.F.,.F.,(4,4),(4,1,1,4),(0.,1.),(0.,0.429964410955918,
0.859928821911836,1.50487543834571),.UNSPECIFIED.);
#1971=B_SPLINE_SURFACE_WITH_KNOTS('',3,3,((#63741,#63742,#63743,#63744,
#63745),(#63746,#63747,#63748,#63749,#63750),(#63751,#63752,#63753,#63754,
#63755),(#63756,#63757,#63758,#63759,#63760)),.UNSPECIFIED.,.F.,.F.,.F.,
(4,4),(4,1,4),(0.,1.),(-2.31999443732384E-6,1.15298346196168,2.69029783790317),
 .UNSPECIFIED.);
#1972=B_SPLINE_SURFACE_WITH_KNOTS('',3,3,((#63764,#63765,#63766,#63767,
#63768,#63769,#63770),(#63771,#63772,#63773,#63774,#63775,#63776,#63777),
(#63778,#63779,#63780,#63781,#63782,#63783,#63784),(#63785,#63786,#63787,
#63788,#63789,#63790,#63791),(#63792,#63793,#63794,#63795,#63796,#63797,
#63798),(#63799,#63800,#63801,#63802,#63803,#63804,#63805)),
 .UNSPECIFIED.,.F.,.F.,.F.,(4,1,1,4),(4,1,1,1,4),(0.,0.285714285714286,
0.571428571428571,1.),(4.94996091805957,5.23536222982578,5.80616485335821,
6.37696747689064,6.94777010042307),.UNSPECIFIED.);
#1973=B_SPLINE_SURFACE_WITH_KNOTS('',3,3,((#63808,#63809,#63810,#63811,
#63812,#63813,#63814),(#63815,#63816,#63817,#63818,#63819,#63820,#63821),
(#63822,#63823,#63824,#63825,#63826,#63827,#63828),(#63829,#63830,#63831,
#63832,#63833,#63834,#63835),(#63836,#63837,#63838,#63839,#63840,#63841,
#63842),(#63843,#63844,#63845,#63846,#63847,#63848,#63849)),
 .UNSPECIFIED.,.F.,.F.,.F.,(4,1,1,4),(4,1,1,1,4),(0.,0.285714285714286,
0.571428571428571,1.),(4.94996091806794,5.23536222983225,5.80616485336088,
6.3769674768895,6.94777010041813),.UNSPECIFIED.);
#1974=B_SPLINE_SURFACE_WITH_KNOTS('',3,3,((#63860,#63861,#63862,#63863,
#63864),(#63865,#63866,#63867,#63868,#63869),(#63870,#63871,#63872,#63873,
#63874),(#63875,#63876,#63877,#63878,#63879)),.UNSPECIFIED.,.F.,.F.,.F.,
(4,4),(4,1,4),(0.,1.),(0.206737365090144,0.851711715694741,1.71167751650087),
 .UNSPECIFIED.);
#1975=B_SPLINE_SURFACE_WITH_KNOTS('',3,3,((#63895,#63896,#63897,#63898),
(#63899,#63900,#63901,#63902),(#63903,#63904,#63905,#63906),(#63907,#63908,
#63909,#63910),(#63911,#63912,#63913,#63914)),.UNSPECIFIED.,.F.,.F.,.F.,
(4,1,4),(4,4),(0.,0.571428571428571,1.),(4.17431363002051,5.27029108627002),
 .UNSPECIFIED.);
#1976=B_SPLINE_SURFACE_WITH_KNOTS('',3,3,((#63948,#63949,#63950,#63951,
#63952),(#63953,#63954,#63955,#63956,#63957),(#63958,#63959,#63960,#63961,
#63962),(#63963,#63964,#63965,#63966,#63967)),.UNSPECIFIED.,.F.,.F.,.F.,
(4,4),(4,1,4),(0.,1.),(-2.31999444274574E-6,1.15298346125989,2.69029783626567),
 .UNSPECIFIED.);
#1977=B_SPLINE_SURFACE_WITH_KNOTS('',3,3,((#64687,#64688,#64689,#64690,
#64691,#64692,#64693,#64694,#64695,#64696,#64697,#64698,#64699,#64700,#64701,
#64702,#64703,#64704,#64705,#64706,#64707,#64708,#64709,#64710,#64711,#64712,
#64713,#64714,#64715,#64716,#64717,#64718,#64719,#64720,#64721,#64722,#64723,
#64724,#64725,#64726,#64727,#64728,#64729,#64730,#64731,#64732,#64733,#64734,
#64735,#64736,#64737,#64738,#64739,#64740,#64741,#64742,#64743,#64744,#64745,
#64746,#64747,#64748,#64749,#64750,#64751,#64752,#64753,#64754,#64755,#64756,
#64757,#64758,#64759,#64760,#64761,#64762,#64763,#64764,#64765,#64766,#64767,
#64768,#64769,#64770,#64771,#64772,#64773,#64774,#64775,#64776,#64777,#64778,
#64779,#64780,#64781,#64782,#64783,#64784,#64785,#64786,#64787,#64788,#64789,
#64790,#64791,#64792,#64793,#64794,#64795,#64796,#64797,#64798,#64799,#64800,
#64801,#64802,#64803,#64804,#64805,#64806,#64807,#64808,#64809,#64810,#64811,
#64812,#64813,#64814,#64815,#64816,#64817,#64818,#64819,#64820,#64821,#64822,
#64823,#64824,#64825,#64826,#64827,#64828,#64829,#64830,#64831,#64832,#64833,
#64834,#64835,#64836,#64837,#64838,#64839,#64840,#64841,#64842,#64843,#64844,
#64845,#64846,#64847,#64848,#64849,#64850,#64851,#64852,#64853,#64854,#64855,
#64856,#64857,#64858,#64859,#64860,#64861,#64862,#64863,#64864,#64865,#64866,
#64867,#64868,#64869,#64870,#64871,#64872,#64873,#64874,#64875,#64876,#64877,
#64878,#64879,#64880,#64881,#64882,#64883,#64884,#64885,#64886,#64887,#64888,
#64889,#64890,#64891,#64892,#64893,#64894,#64895,#64896,#64897,#64898,#64899,
#64900,#64901,#64902,#64903,#64904,#64905,#64906,#64907,#64908,#64909,#64910,
#64911,#64912,#64913,#64914,#64915,#64916,#64917,#64918,#64919,#64920,#64921,
#64922,#64923,#64924,#64925,#64926,#64927,#64928,#64929,#64930,#64931,#64932,
#64933,#64934,#64935,#64936,#64937,#64938,#64939,#64940,#64941,#64942,#64943,
#64944,#64945,#64946,#64947,#64948,#64949,#64950,#64951,#64952,#64953,#64954,
#64955,#64956,#64957,#64958,#64959,#64960,#64961,#64962,#64963,#64964,#64965,
#64966,#64967,#64968,#64969,#64970,#64971,#64972,#64973,#64974,#64975,#64976,
#64977,#64978,#64979,#64980,#64981,#64982,#64983,#64984,#64985,#64986,#64987,
#64988,#64989,#64990,#64991,#64992,#64993,#64994,#64995,#64996,#64997,#64998,
#64999,#65000,#65001,#65002,#65003,#65004,#65005,#65006,#65007,#65008,#65009,
#65010,#65011,#65012,#65013,#65014,#65015,#65016,#65017,#65018,#65019,#65020,
#65021,#65022,#65023,#65024,#65025,#65026,#65027,#65028,#65029,#65030,#65031,
#65032,#65033,#65034,#65035,#65036,#65037,#65038,#65039,#65040,#65041,#65042,
#65043,#65044,#65045,#65046,#65047,#65048,#65049),(#65050,#65051,#65052,
#65053,#65054,#65055,#65056,#65057,#65058,#65059,#65060,#65061,#65062,#65063,
#65064,#65065,#65066,#65067,#65068,#65069,#65070,#65071,#65072,#65073,#65074,
#65075,#65076,#65077,#65078,#65079,#65080,#65081,#65082,#65083,#65084,#65085,
#65086,#65087,#65088,#65089,#65090,#65091,#65092,#65093,#65094,#65095,#65096,
#65097,#65098,#65099,#65100,#65101,#65102,#65103,#65104,#65105,#65106,#65107,
#65108,#65109,#65110,#65111,#65112,#65113,#65114,#65115,#65116,#65117,#65118,
#65119,#65120,#65121,#65122,#65123,#65124,#65125,#65126,#65127,#65128,#65129,
#65130,#65131,#65132,#65133,#65134,#65135,#65136,#65137,#65138,#65139,#65140,
#65141,#65142,#65143,#65144,#65145,#65146,#65147,#65148,#65149,#65150,#65151,
#65152,#65153,#65154,#65155,#65156,#65157,#65158,#65159,#65160,#65161,#65162,
#65163,#65164,#65165,#65166,#65167,#65168,#65169,#65170,#65171,#65172,#65173,
#65174,#65175,#65176,#65177,#65178,#65179,#65180,#65181,#65182,#65183,#65184,
#65185,#65186,#65187,#65188,#65189,#65190,#65191,#65192,#65193,#65194,#65195,
#65196,#65197,#65198,#65199,#65200,#65201,#65202,#65203,#65204,#65205,#65206,
#65207,#65208,#65209,#65210,#65211,#65212,#65213,#65214,#65215,#65216,#65217,
#65218,#65219,#65220,#65221,#65222,#65223,#65224,#65225,#65226,#65227,#65228,
#65229,#65230,#65231,#65232,#65233,#65234,#65235,#65236,#65237,#65238,#65239,
#65240,#65241,#65242,#65243,#65244,#65245,#65246,#65247,#65248,#65249,#65250,
#65251,#65252,#65253,#65254,#65255,#65256,#65257,#65258,#65259,#65260,#65261,
#65262,#65263,#65264,#65265,#65266,#65267,#65268,#65269,#65270,#65271,#65272,
#65273,#65274,#65275,#65276,#65277,#65278,#65279,#65280,#65281,#65282,#65283,
#65284,#65285,#65286,#65287,#65288,#65289,#65290,#65291,#65292,#65293,#65294,
#65295,#65296,#65297,#65298,#65299,#65300,#65301,#65302,#65303,#65304,#65305,
#65306,#65307,#65308,#65309,#65310,#65311,#65312,#65313,#65314,#65315,#65316,
#65317,#65318,#65319,#65320,#65321,#65322,#65323,#65324,#65325,#65326,#65327,
#65328,#65329,#65330,#65331,#65332,#65333,#65334,#65335,#65336,#65337,#65338,
#65339,#65340,#65341,#65342,#65343,#65344,#65345,#65346,#65347,#65348,#65349,
#65350,#65351,#65352,#65353,#65354,#65355,#65356,#65357,#65358,#65359,#65360,
#65361,#65362,#65363,#65364,#65365,#65366,#65367,#65368,#65369,#65370,#65371,
#65372,#65373,#65374,#65375,#65376,#65377,#65378,#65379,#65380,#65381,#65382,
#65383,#65384,#65385,#65386,#65387,#65388,#65389,#65390,#65391,#65392,#65393,
#65394,#65395,#65396,#65397,#65398,#65399,#65400,#65401,#65402,#65403,#65404,
#65405,#65406,#65407,#65408,#65409,#65410,#65411,#65412),(#65413,#65414,
#65415,#65416,#65417,#65418,#65419,#65420,#65421,#65422,#65423,#65424,#65425,
#65426,#65427,#65428,#65429,#65430,#65431,#65432,#65433,#65434,#65435,#65436,
#65437,#65438,#65439,#65440,#65441,#65442,#65443,#65444,#65445,#65446,#65447,
#65448,#65449,#65450,#65451,#65452,#65453,#65454,#65455,#65456,#65457,#65458,
#65459,#65460,#65461,#65462,#65463,#65464,#65465,#65466,#65467,#65468,#65469,
#65470,#65471,#65472,#65473,#65474,#65475,#65476,#65477,#65478,#65479,#65480,
#65481,#65482,#65483,#65484,#65485,#65486,#65487,#65488,#65489,#65490,#65491,
#65492,#65493,#65494,#65495,#65496,#65497,#65498,#65499,#65500,#65501,#65502,
#65503,#65504,#65505,#65506,#65507,#65508,#65509,#65510,#65511,#65512,#65513,
#65514,#65515,#65516,#65517,#65518,#65519,#65520,#65521,#65522,#65523,#65524,
#65525,#65526,#65527,#65528,#65529,#65530,#65531,#65532,#65533,#65534,#65535,
#65536,#65537,#65538,#65539,#65540,#65541,#65542,#65543,#65544,#65545,#65546,
#65547,#65548,#65549,#65550,#65551,#65552,#65553,#65554,#65555,#65556,#65557,
#65558,#65559,#65560,#65561,#65562,#65563,#65564,#65565,#65566,#65567,#65568,
#65569,#65570,#65571,#65572,#65573,#65574,#65575,#65576,#65577,#65578,#65579,
#65580,#65581,#65582,#65583,#65584,#65585,#65586,#65587,#65588,#65589,#65590,
#65591,#65592,#65593,#65594,#65595,#65596,#65597,#65598,#65599,#65600,#65601,
#65602,#65603,#65604,#65605,#65606,#65607,#65608,#65609,#65610,#65611,#65612,
#65613,#65614,#65615,#65616,#65617,#65618,#65619,#65620,#65621,#65622,#65623,
#65624,#65625,#65626,#65627,#65628,#65629,#65630,#65631,#65632,#65633,#65634,
#65635,#65636,#65637,#65638,#65639,#65640,#65641,#65642,#65643,#65644,#65645,
#65646,#65647,#65648,#65649,#65650,#65651,#65652,#65653,#65654,#65655,#65656,
#65657,#65658,#65659,#65660,#65661,#65662,#65663,#65664,#65665,#65666,#65667,
#65668,#65669,#65670,#65671,#65672,#65673,#65674,#65675,#65676,#65677,#65678,
#65679,#65680,#65681,#65682,#65683,#65684,#65685,#65686,#65687,#65688,#65689,
#65690,#65691,#65692,#65693,#65694,#65695,#65696,#65697,#65698,#65699,#65700,
#65701,#65702,#65703,#65704,#65705,#65706,#65707,#65708,#65709,#65710,#65711,
#65712,#65713,#65714,#65715,#65716,#65717,#65718,#65719,#65720,#65721,#65722,
#65723,#65724,#65725,#65726,#65727,#65728,#65729,#65730,#65731,#65732,#65733,
#65734,#65735,#65736,#65737,#65738,#65739,#65740,#65741,#65742,#65743,#65744,
#65745,#65746,#65747,#65748,#65749,#65750,#65751,#65752,#65753,#65754,#65755,
#65756,#65757,#65758,#65759,#65760,#65761,#65762,#65763,#65764,#65765,#65766,
#65767,#65768,#65769,#65770,#65771,#65772,#65773,#65774,#65775),(#65776,
#65777,#65778,#65779,#65780,#65781,#65782,#65783,#65784,#65785,#65786,#65787,
#65788,#65789,#65790,#65791,#65792,#65793,#65794,#65795,#65796,#65797,#65798,
#65799,#65800,#65801,#65802,#65803,#65804,#65805,#65806,#65807,#65808,#65809,
#65810,#65811,#65812,#65813,#65814,#65815,#65816,#65817,#65818,#65819,#65820,
#65821,#65822,#65823,#65824,#65825,#65826,#65827,#65828,#65829,#65830,#65831,
#65832,#65833,#65834,#65835,#65836,#65837,#65838,#65839,#65840,#65841,#65842,
#65843,#65844,#65845,#65846,#65847,#65848,#65849,#65850,#65851,#65852,#65853,
#65854,#65855,#65856,#65857,#65858,#65859,#65860,#65861,#65862,#65863,#65864,
#65865,#65866,#65867,#65868,#65869,#65870,#65871,#65872,#65873,#65874,#65875,
#65876,#65877,#65878,#65879,#65880,#65881,#65882,#65883,#65884,#65885,#65886,
#65887,#65888,#65889,#65890,#65891,#65892,#65893,#65894,#65895,#65896,#65897,
#65898,#65899,#65900,#65901,#65902,#65903,#65904,#65905,#65906,#65907,#65908,
#65909,#65910,#65911,#65912,#65913,#65914,#65915,#65916,#65917,#65918,#65919,
#65920,#65921,#65922,#65923,#65924,#65925,#65926,#65927,#65928,#65929,#65930,
#65931,#65932,#65933,#65934,#65935,#65936,#65937,#65938,#65939,#65940,#65941,
#65942,#65943,#65944,#65945,#65946,#65947,#65948,#65949,#65950,#65951,#65952,
#65953,#65954,#65955,#65956,#65957,#65958,#65959,#65960,#65961,#65962,#65963,
#65964,#65965,#65966,#65967,#65968,#65969,#65970,#65971,#65972,#65973,#65974,
#65975,#65976,#65977,#65978,#65979,#65980,#65981,#65982,#65983,#65984,#65985,
#65986,#65987,#65988,#65989,#65990,#65991,#65992,#65993,#65994,#65995,#65996,
#65997,#65998,#65999,#66000,#66001,#66002,#66003,#66004,#66005,#66006,#66007,
#66008,#66009,#66010,#66011,#66012,#66013,#66014,#66015,#66016,#66017,#66018,
#66019,#66020,#66021,#66022,#66023,#66024,#66025,#66026,#66027,#66028,#66029,
#66030,#66031,#66032,#66033,#66034,#66035,#66036,#66037,#66038,#66039,#66040,
#66041,#66042,#66043,#66044,#66045,#66046,#66047,#66048,#66049,#66050,#66051,
#66052,#66053,#66054,#66055,#66056,#66057,#66058,#66059,#66060,#66061,#66062,
#66063,#66064,#66065,#66066,#66067,#66068,#66069,#66070,#66071,#66072,#66073,
#66074,#66075,#66076,#66077,#66078,#66079,#66080,#66081,#66082,#66083,#66084,
#66085,#66086,#66087,#66088,#66089,#66090,#66091,#66092,#66093,#66094,#66095,
#66096,#66097,#66098,#66099,#66100,#66101,#66102,#66103,#66104,#66105,#66106,
#66107,#66108,#66109,#66110,#66111,#66112,#66113,#66114,#66115,#66116,#66117,
#66118,#66119,#66120,#66121,#66122,#66123,#66124,#66125,#66126,#66127,#66128,
#66129,#66130,#66131,#66132,#66133,#66134,#66135,#66136,#66137,#66138)),
 .UNSPECIFIED.,.F.,.F.,.F.,(4,4),(4,1,1,1,1,1,1,1,1,1,1,1,1,1,1,1,1,1,1,
1,1,1,1,1,1,1,1,1,1,1,1,1,1,1,1,1,1,1,1,1,1,1,1,1,1,1,1,1,1,1,1,1,1,1,1,
1,1,1,1,1,1,1,1,1,1,1,1,1,1,1,1,1,1,1,1,1,1,1,1,1,1,1,1,1,1,1,1,1,1,1,1,
1,1,1,1,1,1,1,1,1,1,1,1,1,1,1,1,1,1,1,1,1,1,1,1,1,1,1,1,1,1,1,1,1,1,1,1,
1,1,1,1,1,1,1,1,1,1,1,1,1,1,1,1,1,1,1,1,1,1,1,1,1,1,1,1,1,1,1,1,1,1,1,1,
1,1,1,1,1,1,1,1,1,1,1,1,1,1,1,1,1,1,1,1,1,1,1,1,1,1,1,1,1,1,1,1,1,1,1,1,
1,1,1,1,1,1,1,1,1,1,1,1,1,1,1,1,1,1,1,1,1,1,1,1,1,1,1,1,1,1,1,1,1,1,1,1,
1,1,1,1,1,1,1,1,1,1,1,1,1,1,1,1,1,1,1,1,1,1,1,1,1,1,1,1,1,1,1,1,1,1,1,1,
1,1,1,1,1,1,1,1,1,1,1,1,1,1,1,1,1,1,1,1,1,1,1,1,1,1,1,1,1,1,1,1,1,1,1,1,
1,1,1,1,1,1,1,1,1,1,1,1,1,1,1,1,1,1,1,1,1,1,1,1,1,1,1,1,1,1,1,1,1,1,1,1,
1,1,1,1,1,1,1,1,1,1,1,1,1,1,1,1,1,4),(0.,0.0989006089183968),(8.30375037697097,
8.80139974796424,9.29904911895752,9.79669848995079,10.2943478609441,10.7919972319373,
11.2896466029306,11.7872959739239,12.2849453449171,12.7825947159104,13.2802440869037,
13.777893457897,14.2755428288902,14.7731921998835,15.2708415708768,15.7684909418701,
16.2661403128633,16.7637896838566,17.2614390548499,17.7590884258431,18.2567377968364,
18.7543871678297,19.252036538823,19.7496859098162,20.2473352808095,20.7449846518028,
21.242634022796,21.7402833937893,22.2379327647826,22.7355821357759,23.2332315067691,
23.7308808777624,24.2285302487557,24.726179619749,25.2238289907422,25.7214783617355,
26.2191277327288,26.716777103722,27.2144264747153,27.7120758457086,28.2097252167019,
28.7073745876951,29.2050239586884,29.7026733296817,30.2003227006749,30.6979720716682,
31.1956214426615,31.6932708136548,32.190920184648,32.6885695556413,33.1862189266346,
33.6838682976279,34.1815176686211,34.6791670396144,35.1768164106077,35.6744657816009,
36.1721151525942,36.6697645235875,37.1674138945808,37.665063265574,38.1627126365673,
38.6603620075606,39.1580113785539,39.6556607495471,40.1533101205404,40.6509594915337,
41.1486088625269,41.6462582335202,42.1439076045135,42.6415569755068,43.1392063465,
43.6368557174933,44.1345050884866,44.6321544594798,45.1298038304731,45.6274532014664,
46.1251025724597,46.6227519434529,47.1204013144462,47.6180506854395,48.1157000564327,
48.613349427426,49.1109987984193,49.6086481694126,50.1062975404058,50.6039469113991,
51.1015962823924,51.5992456533857,52.0968950243789,52.5945443953722,53.0921937663655,
53.5898431373587,54.087492508352,54.5851418793453,55.0827912503386,55.5804406213318,
56.0780899923251,56.5757393633184,57.0733887343116,57.5710381053049,58.0686874762982,
58.5663368472915,59.0639862182847,59.561635589278,60.0592849602713,60.5569343312646,
61.0545837022578,61.5522330732511,62.0498824442444,62.5475318152376,63.0451811862309,
63.5428305572242,64.0404799282175,64.5381292992107,65.035778670204,65.5334280411973,
66.0310774121906,66.5287267831838,67.0263761541771,67.5240255251704,68.0216748961636,
68.5193242671569,69.0169736381502,69.5146230091434,70.0122723801367,70.50992175113,
71.0075711221233,71.5052204931165,72.0028698641098,72.5005192351031,72.9981686060964,
73.4958179770896,73.9934673480829,74.4911167190762,74.9887660900694,75.4864154610627,
75.984064832056,76.4817142030493,76.9793635740425,77.4770129450358,77.9746623160291,
78.4723116870224,78.9699610580156,79.4676104290089,79.9652598000022,80.4629091709954,
80.9605585419887,81.458207912982,81.9558572839753,82.4535066549685,82.9511560259618,
83.4488053969551,83.9464547679483,84.4441041389416,84.9417535099349,85.4394028809282,
85.9370522519214,86.4347016229147,86.932350993908,87.4300003649012,87.9276497358945,
88.4252991068878,88.9229484778811,89.4205978488743,89.9182472198676,90.4158965908609,
90.9135459618542,91.4111953328474,91.9088447038407,92.406494074834,92.9041434458272,
93.4017928168205,93.8994421878138,94.3970915588071,94.8947409298003,95.3923903007936,
95.8900396717869,96.3876890427802,96.8853384137734,97.3829877847667,97.88063715576,
98.3782865267532,98.8759358977465,99.3735852687398,99.8712346397331,100.368884010726,
100.86653338172,101.364182752713,101.861832123706,102.359481494699,102.857130865693,
103.354780236686,103.852429607679,104.350078978673,104.847728349666,105.345377720659,
105.843027091652,106.340676462646,106.838325833639,107.335975204632,107.833624575625,
108.331273946619,108.828923317612,109.326572688605,109.824222059598,110.321871430592,
110.819520801585,111.317170172578,111.814819543572,112.312468914565,112.810118285558,
113.307767656551,113.805417027545,114.303066398538,114.800715769531,115.298365140524,
115.796014511518,116.293663882511,116.791313253504,117.288962624498,117.786611995491,
118.284261366484,118.781910737477,119.279560108471,119.777209479464,120.274858850457,
120.77250822145,121.270157592444,121.767806963437,122.26545633443,122.763105705424,
123.260755076417,123.75840444741,124.256053818403,124.753703189397,125.25135256039,
125.749001931383,126.246651302376,126.74430067337,127.241950044363,127.739599415356,
128.23724878635,128.734898157343,129.232547528336,129.730196899329,130.227846270323,
130.725495641316,131.223145012309,131.720794383302,132.218443754296,132.716093125289,
133.213742496282,133.711391867276,134.209041238269,134.706690609262,135.204339980255,
135.701989351249,136.199638722242,136.697288093235,137.194937464228,137.692586835222,
138.190236206215,138.687885577208,139.185534948202,139.683184319195,140.180833690188,
140.678483061181,141.176132432175,141.673781803168,142.171431174161,142.669080545154,
143.166729916148,143.664379287141,144.162028658134,144.659678029128,145.157327400121,
145.654976771114,146.152626142107,146.650275513101,147.147924884094,147.645574255087,
148.14322362608,148.640872997074,149.138522368067,149.63617173906,150.133821110054,
150.631470481047,151.12911985204,151.626769223033,152.124418594027,152.62206796502,
153.119717336013,153.617366707006,154.115016078,154.612665448993,155.110314819986,
155.60796419098,156.105613561973,156.603262932966,157.100912303959,157.598561674953,
158.096211045946,158.593860416939,159.091509787932,159.589159158926,160.086808529919,
160.584457900912,161.082107271906,161.579756642899,162.077406013892,162.575055384885,
163.072704755879,163.570354126872,164.068003497865,164.565652868858,165.063302239852,
165.560951610845,166.058600981838,166.556250352832,167.053899723825,167.551549094818,
168.049198465811,168.546847836805,169.044497207798,169.542146578791,170.039795949784,
170.537445320778,171.035094691771,171.532744062764,172.030393433758,172.528042804751,
173.025692175744,173.523341546737,174.020990917731,174.518640288724,175.016289659717,
175.51393903071,176.011588401704,176.509237772697,177.00688714369,177.504536514684,
178.002185885677,178.49983525667,178.997484627663,179.495133998657,179.99278336965,
180.490432740643,180.988082111636,181.48573148263,181.983380853623,182.481030224616,
182.97867959561,183.476328966603,183.973978337596,184.471627708589,184.969277079583,
185.466926450576,185.964575821569,186.462225192562,186.959874563556,187.457523934549),
 .UNSPECIFIED.);
#1978=B_SPLINE_SURFACE_WITH_KNOTS('',3,3,((#66276,#66277,#66278,#66279,
#66280,#66281,#66282),(#66283,#66284,#66285,#66286,#66287,#66288,#66289),
(#66290,#66291,#66292,#66293,#66294,#66295,#66296),(#66297,#66298,#66299,
#66300,#66301,#66302,#66303),(#66304,#66305,#66306,#66307,#66308,#66309,
#66310)),.UNSPECIFIED.,.F.,.F.,.F.,(4,1,4),(4,1,1,1,4),(0.,0.5,1.),(-4.31133033879964,
-4.03625205560856,-3.48609548922641,-2.93593892284426,-2.38578235646211),
 .UNSPECIFIED.);
#1979=B_SPLINE_SURFACE_WITH_KNOTS('',3,3,((#66511,#66512,#66513,#66514,
#66515,#66516,#66517,#66518,#66519,#66520,#66521,#66522,#66523,#66524,#66525,
#66526,#66527,#66528,#66529,#66530,#66531,#66532,#66533,#66534,#66535,#66536,
#66537,#66538,#66539,#66540,#66541,#66542,#66543,#66544,#66545,#66546,#66547,
#66548,#66549,#66550,#66551,#66552,#66553,#66554,#66555,#66556,#66557,#66558,
#66559,#66560,#66561,#66562,#66563,#66564,#66565,#66566,#66567,#66568,#66569,
#66570,#66571,#66572,#66573,#66574,#66575,#66576,#66577,#66578,#66579,#66580,
#66581,#66582,#66583,#66584,#66585,#66586,#66587,#66588,#66589,#66590,#66591,
#66592,#66593,#66594,#66595,#66596,#66597,#66598,#66599,#66600,#66601,#66602,
#66603,#66604,#66605,#66606,#66607,#66608,#66609,#66610,#66611,#66612,#66613,
#66614,#66615,#66616,#66617,#66618,#66619,#66620,#66621,#66622,#66623,#66624,
#66625,#66626,#66627,#66628,#66629,#66630,#66631,#66632,#66633,#66634,#66635,
#66636,#66637,#66638,#66639,#66640,#66641,#66642,#66643,#66644,#66645,#66646,
#66647,#66648,#66649,#66650,#66651,#66652,#66653,#66654,#66655,#66656,#66657,
#66658,#66659,#66660,#66661,#66662,#66663,#66664,#66665,#66666,#66667,#66668,
#66669,#66670,#66671,#66672,#66673,#66674,#66675,#66676,#66677,#66678,#66679,
#66680,#66681,#66682,#66683,#66684,#66685,#66686,#66687,#66688,#66689,#66690,
#66691,#66692,#66693,#66694,#66695,#66696,#66697,#66698,#66699,#66700,#66701,
#66702,#66703,#66704,#66705,#66706,#66707,#66708,#66709,#66710,#66711,#66712,
#66713,#66714,#66715,#66716,#66717,#66718,#66719,#66720,#66721,#66722,#66723,
#66724,#66725,#66726,#66727,#66728,#66729,#66730,#66731,#66732,#66733,#66734,
#66735,#66736,#66737,#66738,#66739,#66740,#66741,#66742,#66743,#66744,#66745,
#66746,#66747,#66748,#66749,#66750,#66751,#66752,#66753,#66754,#66755,#66756,
#66757,#66758,#66759,#66760,#66761,#66762,#66763,#66764,#66765,#66766,#66767,
#66768,#66769,#66770,#66771,#66772,#66773,#66774,#66775,#66776,#66777,#66778,
#66779,#66780,#66781,#66782,#66783,#66784,#66785,#66786,#66787,#66788,#66789,
#66790,#66791,#66792,#66793,#66794,#66795,#66796,#66797,#66798,#66799,#66800,
#66801,#66802,#66803,#66804,#66805,#66806,#66807,#66808,#66809,#66810,#66811,
#66812,#66813,#66814,#66815,#66816,#66817,#66818,#66819,#66820,#66821,#66822,
#66823,#66824,#66825,#66826,#66827,#66828,#66829,#66830,#66831,#66832,#66833,
#66834,#66835,#66836,#66837,#66838,#66839,#66840,#66841,#66842,#66843,#66844,
#66845,#66846,#66847,#66848,#66849,#66850,#66851,#66852,#66853,#66854,#66855,
#66856,#66857,#66858,#66859,#66860,#66861,#66862,#66863,#66864,#66865,#66866,
#66867,#66868,#66869,#66870,#66871,#66872,#66873,#66874,#66875,#66876,#66877),
(#66878,#66879,#66880,#66881,#66882,#66883,#66884,#66885,#66886,#66887,
#66888,#66889,#66890,#66891,#66892,#66893,#66894,#66895,#66896,#66897,#66898,
#66899,#66900,#66901,#66902,#66903,#66904,#66905,#66906,#66907,#66908,#66909,
#66910,#66911,#66912,#66913,#66914,#66915,#66916,#66917,#66918,#66919,#66920,
#66921,#66922,#66923,#66924,#66925,#66926,#66927,#66928,#66929,#66930,#66931,
#66932,#66933,#66934,#66935,#66936,#66937,#66938,#66939,#66940,#66941,#66942,
#66943,#66944,#66945,#66946,#66947,#66948,#66949,#66950,#66951,#66952,#66953,
#66954,#66955,#66956,#66957,#66958,#66959,#66960,#66961,#66962,#66963,#66964,
#66965,#66966,#66967,#66968,#66969,#66970,#66971,#66972,#66973,#66974,#66975,
#66976,#66977,#66978,#66979,#66980,#66981,#66982,#66983,#66984,#66985,#66986,
#66987,#66988,#66989,#66990,#66991,#66992,#66993,#66994,#66995,#66996,#66997,
#66998,#66999,#67000,#67001,#67002,#67003,#67004,#67005,#67006,#67007,#67008,
#67009,#67010,#67011,#67012,#67013,#67014,#67015,#67016,#67017,#67018,#67019,
#67020,#67021,#67022,#67023,#67024,#67025,#67026,#67027,#67028,#67029,#67030,
#67031,#67032,#67033,#67034,#67035,#67036,#67037,#67038,#67039,#67040,#67041,
#67042,#67043,#67044,#67045,#67046,#67047,#67048,#67049,#67050,#67051,#67052,
#67053,#67054,#67055,#67056,#67057,#67058,#67059,#67060,#67061,#67062,#67063,
#67064,#67065,#67066,#67067,#67068,#67069,#67070,#67071,#67072,#67073,#67074,
#67075,#67076,#67077,#67078,#67079,#67080,#67081,#67082,#67083,#67084,#67085,
#67086,#67087,#67088,#67089,#67090,#67091,#67092,#67093,#67094,#67095,#67096,
#67097,#67098,#67099,#67100,#67101,#67102,#67103,#67104,#67105,#67106,#67107,
#67108,#67109,#67110,#67111,#67112,#67113,#67114,#67115,#67116,#67117,#67118,
#67119,#67120,#67121,#67122,#67123,#67124,#67125,#67126,#67127,#67128,#67129,
#67130,#67131,#67132,#67133,#67134,#67135,#67136,#67137,#67138,#67139,#67140,
#67141,#67142,#67143,#67144,#67145,#67146,#67147,#67148,#67149,#67150,#67151,
#67152,#67153,#67154,#67155,#67156,#67157,#67158,#67159,#67160,#67161,#67162,
#67163,#67164,#67165,#67166,#67167,#67168,#67169,#67170,#67171,#67172,#67173,
#67174,#67175,#67176,#67177,#67178,#67179,#67180,#67181,#67182,#67183,#67184,
#67185,#67186,#67187,#67188,#67189,#67190,#67191,#67192,#67193,#67194,#67195,
#67196,#67197,#67198,#67199,#67200,#67201,#67202,#67203,#67204,#67205,#67206,
#67207,#67208,#67209,#67210,#67211,#67212,#67213,#67214,#67215,#67216,#67217,
#67218,#67219,#67220,#67221,#67222,#67223,#67224,#67225,#67226,#67227,#67228,
#67229,#67230,#67231,#67232,#67233,#67234,#67235,#67236,#67237,#67238,#67239,
#67240,#67241,#67242,#67243,#67244),(#67245,#67246,#67247,#67248,#67249,
#67250,#67251,#67252,#67253,#67254,#67255,#67256,#67257,#67258,#67259,#67260,
#67261,#67262,#67263,#67264,#67265,#67266,#67267,#67268,#67269,#67270,#67271,
#67272,#67273,#67274,#67275,#67276,#67277,#67278,#67279,#67280,#67281,#67282,
#67283,#67284,#67285,#67286,#67287,#67288,#67289,#67290,#67291,#67292,#67293,
#67294,#67295,#67296,#67297,#67298,#67299,#67300,#67301,#67302,#67303,#67304,
#67305,#67306,#67307,#67308,#67309,#67310,#67311,#67312,#67313,#67314,#67315,
#67316,#67317,#67318,#67319,#67320,#67321,#67322,#67323,#67324,#67325,#67326,
#67327,#67328,#67329,#67330,#67331,#67332,#67333,#67334,#67335,#67336,#67337,
#67338,#67339,#67340,#67341,#67342,#67343,#67344,#67345,#67346,#67347,#67348,
#67349,#67350,#67351,#67352,#67353,#67354,#67355,#67356,#67357,#67358,#67359,
#67360,#67361,#67362,#67363,#67364,#67365,#67366,#67367,#67368,#67369,#67370,
#67371,#67372,#67373,#67374,#67375,#67376,#67377,#67378,#67379,#67380,#67381,
#67382,#67383,#67384,#67385,#67386,#67387,#67388,#67389,#67390,#67391,#67392,
#67393,#67394,#67395,#67396,#67397,#67398,#67399,#67400,#67401,#67402,#67403,
#67404,#67405,#67406,#67407,#67408,#67409,#67410,#67411,#67412,#67413,#67414,
#67415,#67416,#67417,#67418,#67419,#67420,#67421,#67422,#67423,#67424,#67425,
#67426,#67427,#67428,#67429,#67430,#67431,#67432,#67433,#67434,#67435,#67436,
#67437,#67438,#67439,#67440,#67441,#67442,#67443,#67444,#67445,#67446,#67447,
#67448,#67449,#67450,#67451,#67452,#67453,#67454,#67455,#67456,#67457,#67458,
#67459,#67460,#67461,#67462,#67463,#67464,#67465,#67466,#67467,#67468,#67469,
#67470,#67471,#67472,#67473,#67474,#67475,#67476,#67477,#67478,#67479,#67480,
#67481,#67482,#67483,#67484,#67485,#67486,#67487,#67488,#67489,#67490,#67491,
#67492,#67493,#67494,#67495,#67496,#67497,#67498,#67499,#67500,#67501,#67502,
#67503,#67504,#67505,#67506,#67507,#67508,#67509,#67510,#67511,#67512,#67513,
#67514,#67515,#67516,#67517,#67518,#67519,#67520,#67521,#67522,#67523,#67524,
#67525,#67526,#67527,#67528,#67529,#67530,#67531,#67532,#67533,#67534,#67535,
#67536,#67537,#67538,#67539,#67540,#67541,#67542,#67543,#67544,#67545,#67546,
#67547,#67548,#67549,#67550,#67551,#67552,#67553,#67554,#67555,#67556,#67557,
#67558,#67559,#67560,#67561,#67562,#67563,#67564,#67565,#67566,#67567,#67568,
#67569,#67570,#67571,#67572,#67573,#67574,#67575,#67576,#67577,#67578,#67579,
#67580,#67581,#67582,#67583,#67584,#67585,#67586,#67587,#67588,#67589,#67590,
#67591,#67592,#67593,#67594,#67595,#67596,#67597,#67598,#67599,#67600,#67601,
#67602,#67603,#67604,#67605,#67606,#67607,#67608,#67609,#67610,#67611),
(#67612,#67613,#67614,#67615,#67616,#67617,#67618,#67619,#67620,#67621,
#67622,#67623,#67624,#67625,#67626,#67627,#67628,#67629,#67630,#67631,#67632,
#67633,#67634,#67635,#67636,#67637,#67638,#67639,#67640,#67641,#67642,#67643,
#67644,#67645,#67646,#67647,#67648,#67649,#67650,#67651,#67652,#67653,#67654,
#67655,#67656,#67657,#67658,#67659,#67660,#67661,#67662,#67663,#67664,#67665,
#67666,#67667,#67668,#67669,#67670,#67671,#67672,#67673,#67674,#67675,#67676,
#67677,#67678,#67679,#67680,#67681,#67682,#67683,#67684,#67685,#67686,#67687,
#67688,#67689,#67690,#67691,#67692,#67693,#67694,#67695,#67696,#67697,#67698,
#67699,#67700,#67701,#67702,#67703,#67704,#67705,#67706,#67707,#67708,#67709,
#67710,#67711,#67712,#67713,#67714,#67715,#67716,#67717,#67718,#67719,#67720,
#67721,#67722,#67723,#67724,#67725,#67726,#67727,#67728,#67729,#67730,#67731,
#67732,#67733,#67734,#67735,#67736,#67737,#67738,#67739,#67740,#67741,#67742,
#67743,#67744,#67745,#67746,#67747,#67748,#67749,#67750,#67751,#67752,#67753,
#67754,#67755,#67756,#67757,#67758,#67759,#67760,#67761,#67762,#67763,#67764,
#67765,#67766,#67767,#67768,#67769,#67770,#67771,#67772,#67773,#67774,#67775,
#67776,#67777,#67778,#67779,#67780,#67781,#67782,#67783,#67784,#67785,#67786,
#67787,#67788,#67789,#67790,#67791,#67792,#67793,#67794,#67795,#67796,#67797,
#67798,#67799,#67800,#67801,#67802,#67803,#67804,#67805,#67806,#67807,#67808,
#67809,#67810,#67811,#67812,#67813,#67814,#67815,#67816,#67817,#67818,#67819,
#67820,#67821,#67822,#67823,#67824,#67825,#67826,#67827,#67828,#67829,#67830,
#67831,#67832,#67833,#67834,#67835,#67836,#67837,#67838,#67839,#67840,#67841,
#67842,#67843,#67844,#67845,#67846,#67847,#67848,#67849,#67850,#67851,#67852,
#67853,#67854,#67855,#67856,#67857,#67858,#67859,#67860,#67861,#67862,#67863,
#67864,#67865,#67866,#67867,#67868,#67869,#67870,#67871,#67872,#67873,#67874,
#67875,#67876,#67877,#67878,#67879,#67880,#67881,#67882,#67883,#67884,#67885,
#67886,#67887,#67888,#67889,#67890,#67891,#67892,#67893,#67894,#67895,#67896,
#67897,#67898,#67899,#67900,#67901,#67902,#67903,#67904,#67905,#67906,#67907,
#67908,#67909,#67910,#67911,#67912,#67913,#67914,#67915,#67916,#67917,#67918,
#67919,#67920,#67921,#67922,#67923,#67924,#67925,#67926,#67927,#67928,#67929,
#67930,#67931,#67932,#67933,#67934,#67935,#67936,#67937,#67938,#67939,#67940,
#67941,#67942,#67943,#67944,#67945,#67946,#67947,#67948,#67949,#67950,#67951,
#67952,#67953,#67954,#67955,#67956,#67957,#67958,#67959,#67960,#67961,#67962,
#67963,#67964,#67965,#67966,#67967,#67968,#67969,#67970,#67971,#67972,#67973,
#67974,#67975,#67976,#67977,#67978)),.UNSPECIFIED.,.F.,.F.,.F.,(4,4),(4,
1,1,1,1,1,1,1,1,1,1,1,1,1,1,1,1,1,1,1,1,1,1,1,1,1,1,1,1,1,1,1,1,1,1,1,1,
1,1,1,1,1,1,1,1,1,1,1,1,1,1,1,1,1,1,1,1,1,1,1,1,1,1,1,1,1,1,1,1,1,1,1,1,
1,1,1,1,1,1,1,1,1,1,1,1,1,1,1,1,1,1,1,1,1,1,1,1,1,1,1,1,1,1,1,1,1,1,1,1,
1,1,1,1,1,1,1,1,1,1,1,1,1,1,1,1,1,1,1,1,1,1,1,1,1,1,1,1,1,1,1,1,1,1,1,1,
1,1,1,1,1,1,1,1,1,1,1,1,1,1,1,1,1,1,1,1,1,1,1,1,1,1,1,1,1,1,1,1,1,1,1,1,
1,1,1,1,1,1,1,1,1,1,1,1,1,1,1,1,1,1,1,1,1,1,1,1,1,1,1,1,1,1,1,1,1,1,1,1,
1,1,1,1,1,1,1,1,1,1,1,1,1,1,1,1,1,1,1,1,1,1,1,1,1,1,1,1,1,1,1,1,1,1,1,1,
1,1,1,1,1,1,1,1,1,1,1,1,1,1,1,1,1,1,1,1,1,1,1,1,1,1,1,1,1,1,1,1,1,1,1,1,
1,1,1,1,1,1,1,1,1,1,1,1,1,1,1,1,1,1,1,1,1,1,1,1,1,1,1,1,1,1,1,1,1,1,1,1,
1,1,1,1,1,1,1,1,1,1,1,1,1,1,1,1,1,1,1,1,1,1,1,1,1,1,1,1,1,1,1,1,1,1,1,1,
1,1,1,4),(-2.53587172121443E-8,0.0989001011122836),(9.22778945151176,9.72652408304394,
10.2252587145761,10.7239933461083,11.2227279776405,11.7214626091727,12.2201972407048,
12.718931872237,13.2176665037692,13.7164011353014,14.2151357668335,14.7138703983657,
15.2126050298979,15.7113396614301,16.2100742929623,16.7088089244944,17.2075435560266,
17.7062781875588,18.205012819091,18.7037474506231,19.2024820821553,19.7012167136875,
20.1999513452197,20.6986859767519,21.197420608284,21.6961552398162,22.1948898713484,
22.6936245028806,23.1923591344127,23.6910937659449,24.1898283974771,24.6885630290093,
25.1872976605415,25.6860322920736,26.1847669236058,26.683501555138,27.1822361866702,
27.6809708182023,28.1797054497345,28.6784400812667,29.1771747127989,29.6759093443311,
30.1746439758632,30.6733786073954,31.1721132389276,31.6708478704598,32.1695825019919,
32.6683171335241,33.1670517650563,33.6657863965885,34.1645210281207,34.6632556596528,
35.161990291185,35.6607249227172,36.1594595542494,36.6581941857815,37.1569288173137,
37.6556634488459,38.1543980803781,38.6531327119103,39.1518673434424,39.6506019749746,
40.1493366065068,40.648071238039,41.1468058695711,41.6455405011033,42.1442751326355,
42.6430097641677,43.1417443956999,43.640479027232,44.1392136587642,44.6379482902964,
45.1366829218286,45.6354175533607,46.1341521848929,46.6328868164251,47.1316214479573,
47.6303560794895,48.1290907110216,48.6278253425538,49.126559974086,49.6252946056182,
50.1240292371503,50.6227638686825,51.1214985002147,51.6202331317469,52.1189677632791,
52.6177023948112,53.1164370263434,53.6151716578756,54.1139062894078,54.6126409209399,
55.1113755524721,55.6101101840043,56.1088448155365,56.6075794470687,57.1063140786008,
57.605048710133,58.1037833416652,58.6025179731974,59.1012526047295,59.5999872362617,
60.0987218677939,60.5974564993261,61.0961911308583,61.5949257623904,62.0936603939226,
62.5923950254548,63.091129656987,63.5898642885191,64.0885989200513,64.5873335515835,
65.0860681831157,65.5848028146479,66.08353744618,66.5822720777122,67.0810067092444,
67.5797413407766,68.0784759723088,68.5772106038409,69.0759452353731,69.5746798669053,
70.0734144984375,70.5721491299696,71.0708837615018,71.569618393034,72.0683530245662,
72.5670876560984,73.0658222876305,73.5645569191627,74.0632915506949,74.5620261822271,
75.0607608137592,75.5594954452914,76.0582300768236,76.5569647083558,77.055699339888,
77.5544339714201,78.0531686029523,78.5519032344845,79.0506378660167,79.5493724975488,
80.048107129081,80.5468417606132,81.0455763921454,81.5443110236776,82.0430456552097,
82.5417802867419,83.0405149182741,83.5392495498063,84.0379841813384,84.5367188128706,
85.0354534444028,85.534188075935,86.0329227074672,86.5316573389993,87.0303919705315,
87.5291266020637,88.0278612335959,88.526595865128,89.0253304966602,89.5240651281924,
90.0227997597246,90.5215343912568,91.0202690227889,91.5190036543211,92.0177382858533,
92.5164729173855,93.0152075489176,93.5139421804498,94.012676811982,94.5114114435142,
95.0101460750464,95.5088807065785,96.0076153381107,96.5063499696429,97.0050846011751,
97.5038192327072,98.0025538642394,98.5012884957716,99.0000231273038,99.4987577588359,
99.9974923903681,100.4962270219,100.994961653432,101.493696284965,101.992430916497,
102.491165548029,102.989900179561,103.488634811093,103.987369442626,104.486104074158,
104.98483870569,105.483573337222,105.982307968754,106.481042600286,106.979777231819,
107.478511863351,107.977246494883,108.475981126415,108.974715757947,109.47345038948,
109.972185021012,110.470919652544,110.969654284076,111.468388915608,111.96712354714,
112.465858178673,112.964592810205,113.463327441737,113.962062073269,114.460796704801,
114.959531336333,115.458265967866,115.957000599398,116.45573523093,116.954469862462,
117.453204493994,117.951939125527,118.450673757059,118.949408388591,119.448143020123,
119.946877651655,120.445612283187,120.94434691472,121.443081546252,121.941816177784,
122.440550809316,122.939285440848,123.43802007238,123.936754703913,124.435489335445,
124.934223966977,125.432958598509,125.931693230041,126.430427861574,126.929162493106,
127.427897124638,127.92663175617,128.425366387702,128.924101019234,129.422835650767,
129.921570282299,130.420304913831,130.919039545363,131.417774176895,131.916508808428,
132.41524343996,132.913978071492,133.412712703024,133.911447334556,134.410181966088,
134.908916597621,135.407651229153,135.906385860685,136.405120492217,136.903855123749,
137.402589755281,137.901324386814,138.400059018346,138.898793649878,139.39752828141,
139.896262912942,140.394997544475,140.893732176007,141.392466807539,141.891201439071,
142.389936070603,142.888670702135,143.387405333668,143.8861399652,144.384874596732,
144.883609228264,145.382343859796,145.881078491329,146.379813122861,146.878547754393,
147.377282385925,147.876017017457,148.374751648989,148.873486280522,149.372220912054,
149.870955543586,150.369690175118,150.86842480665,151.367159438182,151.865894069715,
152.364628701247,152.863363332779,153.362097964311,153.860832595843,154.359567227376,
154.858301858908,155.35703649044,155.855771121972,156.354505753504,156.853240385036,
157.351975016569,157.850709648101,158.349444279633,158.848178911165,159.346913542697,
159.845648174229,160.344382805762,160.843117437294,161.341852068826,161.840586700358,
162.33932133189,162.838055963423,163.336790594955,163.835525226487,164.334259858019,
164.832994489551,165.331729121083,165.830463752616,166.329198384148,166.82793301568,
167.326667647212,167.825402278744,168.324136910276,168.822871541809,169.321606173341,
169.820340804873,170.319075436405,170.817810067937,171.31654469947,171.815279331002,
172.314013962534,172.812748594066,173.311483225598,173.81021785713,174.308952488663,
174.807687120195,175.306421751727,175.805156383259,176.303891014791,176.802625646324,
177.301360277856,177.800094909388,178.29882954092,178.797564172452,179.296298803984,
179.795033435517,180.293768067049,180.792502698581,181.291237330113,181.789971961645,
182.288706593177,182.78744122471,183.286175856242,183.784910487774,184.283645119306,
184.782379750838,185.281114382371,185.779849013903,186.278583645435,186.777318276967,
187.276052908499,187.774787540031,188.273522171564,188.772256803096,189.270991434628,
189.76972606616,190.268460697692,190.767195329225),.UNSPECIFIED.);
#2145=FACE_OUTER_BOUND('',#4542,.T.);
#2146=FACE_OUTER_BOUND('',#4543,.T.);
#2147=FACE_OUTER_BOUND('',#4544,.T.);
#2148=FACE_OUTER_BOUND('',#4545,.T.);
#2149=FACE_OUTER_BOUND('',#4546,.T.);
#2150=FACE_OUTER_BOUND('',#4547,.T.);
#2151=FACE_OUTER_BOUND('',#4548,.T.);
#2152=FACE_OUTER_BOUND('',#4549,.T.);
#2153=FACE_OUTER_BOUND('',#4550,.T.);
#2154=FACE_OUTER_BOUND('',#4551,.T.);
#2155=FACE_OUTER_BOUND('',#4552,.T.);
#2156=FACE_OUTER_BOUND('',#4553,.T.);
#2157=FACE_OUTER_BOUND('',#4554,.T.);
#2158=FACE_OUTER_BOUND('',#4555,.T.);
#2159=FACE_OUTER_BOUND('',#4556,.T.);
#2160=FACE_OUTER_BOUND('',#4557,.T.);
#2161=FACE_OUTER_BOUND('',#4558,.T.);
#2162=FACE_OUTER_BOUND('',#4559,.T.);
#2163=FACE_OUTER_BOUND('',#4560,.T.);
#2164=FACE_OUTER_BOUND('',#4561,.T.);
#2165=FACE_OUTER_BOUND('',#4562,.T.);
#2166=FACE_OUTER_BOUND('',#4563,.T.);
#2167=FACE_OUTER_BOUND('',#4564,.T.);
#2168=FACE_OUTER_BOUND('',#4565,.T.);
#2169=FACE_OUTER_BOUND('',#4566,.T.);
#2170=FACE_OUTER_BOUND('',#4567,.T.);
#2171=FACE_OUTER_BOUND('',#4568,.T.);
#2172=FACE_OUTER_BOUND('',#4569,.T.);
#2173=FACE_OUTER_BOUND('',#4570,.T.);
#2174=FACE_OUTER_BOUND('',#4571,.T.);
#2175=FACE_OUTER_BOUND('',#4572,.T.);
#2176=FACE_OUTER_BOUND('',#4573,.T.);
#2177=FACE_OUTER_BOUND('',#4574,.T.);
#2178=FACE_OUTER_BOUND('',#4575,.T.);
#2179=FACE_OUTER_BOUND('',#4576,.T.);
#2180=FACE_OUTER_BOUND('',#4577,.T.);
#2181=FACE_OUTER_BOUND('',#4578,.T.);
#2182=FACE_OUTER_BOUND('',#4579,.T.);
#2183=FACE_OUTER_BOUND('',#4580,.T.);
#2184=FACE_OUTER_BOUND('',#4581,.T.);
#2185=FACE_OUTER_BOUND('',#4582,.T.);
#2186=FACE_OUTER_BOUND('',#4583,.T.);
#2187=FACE_OUTER_BOUND('',#4584,.T.);
#2188=FACE_OUTER_BOUND('',#4585,.T.);
#2189=FACE_OUTER_BOUND('',#4586,.T.);
#2190=FACE_OUTER_BOUND('',#4587,.T.);
#2191=FACE_OUTER_BOUND('',#4588,.T.);
#2192=FACE_OUTER_BOUND('',#4589,.T.);
#2193=FACE_OUTER_BOUND('',#4590,.T.);
#2194=FACE_OUTER_BOUND('',#4591,.T.);
#2195=FACE_OUTER_BOUND('',#4592,.T.);
#2196=FACE_OUTER_BOUND('',#4593,.T.);
#2197=FACE_OUTER_BOUND('',#4594,.T.);
#2198=FACE_OUTER_BOUND('',#4595,.T.);
#2199=FACE_OUTER_BOUND('',#4596,.T.);
#2200=FACE_OUTER_BOUND('',#4597,.T.);
#2201=FACE_OUTER_BOUND('',#4598,.T.);
#2202=FACE_OUTER_BOUND('',#4599,.T.);
#2203=FACE_OUTER_BOUND('',#4600,.T.);
#2204=FACE_OUTER_BOUND('',#4601,.T.);
#2205=FACE_OUTER_BOUND('',#4603,.T.);
#2206=FACE_OUTER_BOUND('',#4604,.T.);
#2207=FACE_OUTER_BOUND('',#4605,.T.);
#2208=FACE_OUTER_BOUND('',#4606,.T.);
#2209=FACE_OUTER_BOUND('',#4607,.T.);
#2210=FACE_OUTER_BOUND('',#4608,.T.);
#2211=FACE_OUTER_BOUND('',#4609,.T.);
#2212=FACE_OUTER_BOUND('',#4610,.T.);
#2213=FACE_OUTER_BOUND('',#4611,.T.);
#2214=FACE_OUTER_BOUND('',#4613,.T.);
#2215=FACE_OUTER_BOUND('',#4614,.T.);
#2216=FACE_OUTER_BOUND('',#4616,.T.);
#2217=FACE_OUTER_BOUND('',#4617,.T.);
#2218=FACE_OUTER_BOUND('',#4618,.T.);
#2219=FACE_OUTER_BOUND('',#4620,.T.);
#2220=FACE_OUTER_BOUND('',#4621,.T.);
#2221=FACE_OUTER_BOUND('',#4622,.T.);
#2222=FACE_OUTER_BOUND('',#4623,.T.);
#2223=FACE_OUTER_BOUND('',#4624,.T.);
#2224=FACE_OUTER_BOUND('',#4625,.T.);
#2225=FACE_OUTER_BOUND('',#4626,.T.);
#2226=FACE_OUTER_BOUND('',#4627,.T.);
#2227=FACE_OUTER_BOUND('',#4628,.T.);
#2228=FACE_OUTER_BOUND('',#4629,.T.);
#2229=FACE_OUTER_BOUND('',#4630,.T.);
#2230=FACE_OUTER_BOUND('',#4631,.T.);
#2231=FACE_OUTER_BOUND('',#4632,.T.);
#2232=FACE_OUTER_BOUND('',#4633,.T.);
#2233=FACE_OUTER_BOUND('',#4634,.T.);
#2234=FACE_OUTER_BOUND('',#4635,.T.);
#2235=FACE_OUTER_BOUND('',#4636,.T.);
#2236=FACE_OUTER_BOUND('',#4637,.T.);
#2237=FACE_OUTER_BOUND('',#4638,.T.);
#2238=FACE_OUTER_BOUND('',#4639,.T.);
#2239=FACE_OUTER_BOUND('',#4640,.T.);
#2240=FACE_OUTER_BOUND('',#4641,.T.);
#2241=FACE_OUTER_BOUND('',#4642,.T.);
#2242=FACE_OUTER_BOUND('',#4643,.T.);
#2243=FACE_OUTER_BOUND('',#4644,.T.);
#2244=FACE_OUTER_BOUND('',#4645,.T.);
#2245=FACE_OUTER_BOUND('',#4646,.T.);
#2246=FACE_OUTER_BOUND('',#4647,.T.);
#2247=FACE_OUTER_BOUND('',#4648,.T.);
#2248=FACE_OUTER_BOUND('',#4650,.T.);
#2249=FACE_OUTER_BOUND('',#4651,.T.);
#2250=FACE_OUTER_BOUND('',#4652,.T.);
#2251=FACE_OUTER_BOUND('',#4653,.T.);
#2252=FACE_OUTER_BOUND('',#4654,.T.);
#2253=FACE_OUTER_BOUND('',#4655,.T.);
#2254=FACE_OUTER_BOUND('',#4656,.T.);
#2255=FACE_OUTER_BOUND('',#4657,.T.);
#2256=FACE_OUTER_BOUND('',#4658,.T.);
#2257=FACE_OUTER_BOUND('',#4659,.T.);
#2258=FACE_OUTER_BOUND('',#4660,.T.);
#2259=FACE_OUTER_BOUND('',#4661,.T.);
#2260=FACE_OUTER_BOUND('',#4662,.T.);
#2261=FACE_OUTER_BOUND('',#4663,.T.);
#2262=FACE_OUTER_BOUND('',#4664,.T.);
#2263=FACE_OUTER_BOUND('',#4665,.T.);
#2264=FACE_OUTER_BOUND('',#4666,.T.);
#2265=FACE_OUTER_BOUND('',#4667,.T.);
#2266=FACE_OUTER_BOUND('',#4668,.T.);
#2267=FACE_OUTER_BOUND('',#4669,.T.);
#2268=FACE_OUTER_BOUND('',#4670,.T.);
#2269=FACE_OUTER_BOUND('',#4671,.T.);
#2270=FACE_OUTER_BOUND('',#4672,.T.);
#2271=FACE_OUTER_BOUND('',#4673,.T.);
#2272=FACE_OUTER_BOUND('',#4674,.T.);
#2273=FACE_OUTER_BOUND('',#4675,.T.);
#2274=FACE_OUTER_BOUND('',#4676,.T.);
#2275=FACE_OUTER_BOUND('',#4677,.T.);
#2276=FACE_OUTER_BOUND('',#4678,.T.);
#2277=FACE_OUTER_BOUND('',#4679,.T.);
#2278=FACE_OUTER_BOUND('',#4680,.T.);
#2279=FACE_OUTER_BOUND('',#4681,.T.);
#2280=FACE_OUTER_BOUND('',#4682,.T.);
#2281=FACE_OUTER_BOUND('',#4683,.T.);
#2282=FACE_OUTER_BOUND('',#4684,.T.);
#2283=FACE_OUTER_BOUND('',#4685,.T.);
#2284=FACE_OUTER_BOUND('',#4686,.T.);
#2285=FACE_OUTER_BOUND('',#4687,.T.);
#2286=FACE_OUTER_BOUND('',#4688,.T.);
#2287=FACE_OUTER_BOUND('',#4689,.T.);
#2288=FACE_OUTER_BOUND('',#4690,.T.);
#2289=FACE_OUTER_BOUND('',#4691,.T.);
#2290=FACE_OUTER_BOUND('',#4692,.T.);
#2291=FACE_OUTER_BOUND('',#4693,.T.);
#2292=FACE_OUTER_BOUND('',#4694,.T.);
#2293=FACE_OUTER_BOUND('',#4696,.T.);
#2294=FACE_OUTER_BOUND('',#4697,.T.);
#2295=FACE_OUTER_BOUND('',#4698,.T.);
#2296=FACE_OUTER_BOUND('',#4699,.T.);
#2297=FACE_OUTER_BOUND('',#4700,.T.);
#2298=FACE_OUTER_BOUND('',#4701,.T.);
#2299=FACE_OUTER_BOUND('',#4702,.T.);
#2300=FACE_OUTER_BOUND('',#4703,.T.);
#2301=FACE_OUTER_BOUND('',#4704,.T.);
#2302=FACE_OUTER_BOUND('',#4705,.T.);
#2303=FACE_OUTER_BOUND('',#4706,.T.);
#2304=FACE_OUTER_BOUND('',#4707,.T.);
#2305=FACE_OUTER_BOUND('',#4708,.T.);
#2306=FACE_OUTER_BOUND('',#4709,.T.);
#2307=FACE_OUTER_BOUND('',#4710,.T.);
#2308=FACE_OUTER_BOUND('',#4711,.T.);
#2309=FACE_OUTER_BOUND('',#4712,.T.);
#2310=FACE_OUTER_BOUND('',#4713,.T.);
#2311=FACE_OUTER_BOUND('',#4714,.T.);
#2312=FACE_OUTER_BOUND('',#4715,.T.);
#2313=FACE_OUTER_BOUND('',#4716,.T.);
#2314=FACE_OUTER_BOUND('',#4717,.T.);
#2315=FACE_OUTER_BOUND('',#4718,.T.);
#2316=FACE_OUTER_BOUND('',#4719,.T.);
#2317=FACE_OUTER_BOUND('',#4720,.T.);
#2318=FACE_OUTER_BOUND('',#4721,.T.);
#2319=FACE_OUTER_BOUND('',#4722,.T.);
#2320=FACE_OUTER_BOUND('',#4723,.T.);
#2321=FACE_OUTER_BOUND('',#4724,.T.);
#2322=FACE_OUTER_BOUND('',#4725,.T.);
#2323=FACE_OUTER_BOUND('',#4726,.T.);
#2324=FACE_OUTER_BOUND('',#4728,.T.);
#2325=FACE_OUTER_BOUND('',#4729,.T.);
#2326=FACE_OUTER_BOUND('',#4730,.T.);
#2327=FACE_OUTER_BOUND('',#4731,.T.);
#2328=FACE_OUTER_BOUND('',#4732,.T.);
#2329=FACE_OUTER_BOUND('',#4733,.T.);
#2330=FACE_OUTER_BOUND('',#4734,.T.);
#2331=FACE_OUTER_BOUND('',#4735,.T.);
#2332=FACE_OUTER_BOUND('',#4736,.T.);
#2333=FACE_OUTER_BOUND('',#4737,.T.);
#2334=FACE_OUTER_BOUND('',#4738,.T.);
#2335=FACE_OUTER_BOUND('',#4739,.T.);
#2336=FACE_OUTER_BOUND('',#4740,.T.);
#2337=FACE_OUTER_BOUND('',#4741,.T.);
#2338=FACE_OUTER_BOUND('',#4742,.T.);
#2339=FACE_OUTER_BOUND('',#4743,.T.);
#2340=FACE_OUTER_BOUND('',#4744,.T.);
#2341=FACE_OUTER_BOUND('',#4745,.T.);
#2342=FACE_OUTER_BOUND('',#4746,.T.);
#2343=FACE_OUTER_BOUND('',#4747,.T.);
#2344=FACE_OUTER_BOUND('',#4748,.T.);
#2345=FACE_OUTER_BOUND('',#4749,.T.);
#2346=FACE_OUTER_BOUND('',#4750,.T.);
#2347=FACE_OUTER_BOUND('',#4751,.T.);
#2348=FACE_OUTER_BOUND('',#4752,.T.);
#2349=FACE_OUTER_BOUND('',#4753,.T.);
#2350=FACE_OUTER_BOUND('',#4754,.T.);
#2351=FACE_OUTER_BOUND('',#4755,.T.);
#2352=FACE_OUTER_BOUND('',#4756,.T.);
#2353=FACE_OUTER_BOUND('',#4757,.T.);
#2354=FACE_OUTER_BOUND('',#4758,.T.);
#2355=FACE_OUTER_BOUND('',#4759,.T.);
#2356=FACE_OUTER_BOUND('',#4760,.T.);
#2357=FACE_OUTER_BOUND('',#4761,.T.);
#2358=FACE_OUTER_BOUND('',#4762,.T.);
#2359=FACE_OUTER_BOUND('',#4763,.T.);
#2360=FACE_OUTER_BOUND('',#4764,.T.);
#2361=FACE_OUTER_BOUND('',#4765,.T.);
#2362=FACE_OUTER_BOUND('',#4766,.T.);
#4542=EDGE_LOOP('',(#25125,#25126,#25127));
#4543=EDGE_LOOP('',(#25128,#25129,#25130,#25131,#25132));
#4544=EDGE_LOOP('',(#25133,#25134,#25135,#25136));
#4545=EDGE_LOOP('',(#25137,#25138,#25139,#25140));
#4546=EDGE_LOOP('',(#25141,#25142,#25143,#25144));
#4547=EDGE_LOOP('',(#25145,#25146,#25147,#25148));
#4548=EDGE_LOOP('',(#25149,#25150,#25151,#25152));
#4549=EDGE_LOOP('',(#25153,#25154,#25155,#25156));
#4550=EDGE_LOOP('',(#25157,#25158,#25159,#25160));
#4551=EDGE_LOOP('',(#25161,#25162,#25163,#25164));
#4552=EDGE_LOOP('',(#25165,#25166,#25167,#25168));
#4553=EDGE_LOOP('',(#25169,#25170,#25171,#25172));
#4554=EDGE_LOOP('',(#25173,#25174,#25175,#25176));
#4555=EDGE_LOOP('',(#25177,#25178,#25179,#25180));
#4556=EDGE_LOOP('',(#25181,#25182,#25183,#25184));
#4557=EDGE_LOOP('',(#25185,#25186,#25187,#25188));
#4558=EDGE_LOOP('',(#25189,#25190,#25191,#25192));
#4559=EDGE_LOOP('',(#25193,#25194,#25195,#25196));
#4560=EDGE_LOOP('',(#25197,#25198,#25199,#25200));
#4561=EDGE_LOOP('',(#25201,#25202,#25203,#25204));
#4562=EDGE_LOOP('',(#25205,#25206,#25207,#25208));
#4563=EDGE_LOOP('',(#25209,#25210,#25211,#25212));
#4564=EDGE_LOOP('',(#25213,#25214,#25215,#25216));
#4565=EDGE_LOOP('',(#25217,#25218,#25219,#25220));
#4566=EDGE_LOOP('',(#25221,#25222,#25223,#25224));
#4567=EDGE_LOOP('',(#25225,#25226,#25227,#25228));
#4568=EDGE_LOOP('',(#25229,#25230,#25231,#25232));
#4569=EDGE_LOOP('',(#25233,#25234,#25235,#25236));
#4570=EDGE_LOOP('',(#25237,#25238,#25239,#25240,#25241));
#4571=EDGE_LOOP('',(#25242,#25243,#25244,#25245));
#4572=EDGE_LOOP('',(#25246,#25247,#25248,#25249));
#4573=EDGE_LOOP('',(#25250,#25251,#25252,#25253));
#4574=EDGE_LOOP('',(#25254,#25255,#25256,#25257));
#4575=EDGE_LOOP('',(#25258,#25259,#25260,#25261));
#4576=EDGE_LOOP('',(#25262,#25263,#25264,#25265));
#4577=EDGE_LOOP('',(#25266,#25267,#25268,#25269));
#4578=EDGE_LOOP('',(#25270,#25271,#25272,#25273));
#4579=EDGE_LOOP('',(#25274,#25275,#25276,#25277));
#4580=EDGE_LOOP('',(#25278,#25279,#25280,#25281));
#4581=EDGE_LOOP('',(#25282,#25283,#25284,#25285));
#4582=EDGE_LOOP('',(#25286,#25287,#25288,#25289));
#4583=EDGE_LOOP('',(#25290,#25291,#25292,#25293));
#4584=EDGE_LOOP('',(#25294,#25295,#25296,#25297));
#4585=EDGE_LOOP('',(#25298,#25299,#25300,#25301));
#4586=EDGE_LOOP('',(#25302,#25303,#25304,#25305));
#4587=EDGE_LOOP('',(#25306,#25307,#25308,#25309));
#4588=EDGE_LOOP('',(#25310,#25311,#25312,#25313));
#4589=EDGE_LOOP('',(#25314,#25315,#25316,#25317));
#4590=EDGE_LOOP('',(#25318,#25319,#25320,#25321));
#4591=EDGE_LOOP('',(#25322,#25323,#25324,#25325));
#4592=EDGE_LOOP('',(#25326,#25327,#25328,#25329));
#4593=EDGE_LOOP('',(#25330,#25331,#25332,#25333));
#4594=EDGE_LOOP('',(#25334,#25335,#25336,#25337));
#4595=EDGE_LOOP('',(#25338,#25339,#25340,#25341));
#4596=EDGE_LOOP('',(#25342,#25343,#25344,#25345));
#4597=EDGE_LOOP('',(#25346,#25347,#25348,#25349));
#4598=EDGE_LOOP('',(#25350,#25351,#25352,#25353));
#4599=EDGE_LOOP('',(#25354,#25355,#25356,#25357));
#4600=EDGE_LOOP('',(#25358,#25359,#25360,#25361));
#4601=EDGE_LOOP('',(#25362));
#4602=EDGE_LOOP('',(#25363));
#4603=EDGE_LOOP('',(#25364,#25365,#25366,#25367,#25368));
#4604=EDGE_LOOP('',(#25369,#25370,#25371,#25372,#25373,#25374));
#4605=EDGE_LOOP('',(#25375,#25376,#25377,#25378,#25379));
#4606=EDGE_LOOP('',(#25380,#25381,#25382,#25383,#25384));
#4607=EDGE_LOOP('',(#25385,#25386,#25387,#25388,#25389,#25390));
#4608=EDGE_LOOP('',(#25391,#25392,#25393,#25394,#25395,#25396));
#4609=EDGE_LOOP('',(#25397,#25398,#25399,#25400,#25401,#25402));
#4610=EDGE_LOOP('',(#25403,#25404,#25405,#25406,#25407));
#4611=EDGE_LOOP('',(#25408));
#4612=EDGE_LOOP('',(#25409));
#4613=EDGE_LOOP('',(#25410,#25411,#25412,#25413,#25414));
#4614=EDGE_LOOP('',(#25415));
#4615=EDGE_LOOP('',(#25416));
#4616=EDGE_LOOP('',(#25417,#25418,#25419,#25420,#25421));
#4617=EDGE_LOOP('',(#25422,#25423,#25424,#25425,#25426));
#4618=EDGE_LOOP('',(#25427));
#4619=EDGE_LOOP('',(#25428,#25429,#25430,#25431,#25432,#25433,#25434,#25435,
#25436,#25437,#25438,#25439,#25440,#25441,#25442,#25443,#25444,#25445,#25446,
#25447,#25448,#25449,#25450,#25451,#25452,#25453,#25454,#25455,#25456,#25457,
#25458,#25459,#25460,#25461,#25462,#25463,#25464,#25465,#25466,#25467,#25468,
#25469,#25470,#25471,#25472,#25473,#25474,#25475,#25476,#25477,#25478,#25479,
#25480,#25481));
#4620=EDGE_LOOP('',(#25482,#25483,#25484,#25485,#25486));
#4621=EDGE_LOOP('',(#25487,#25488,#25489,#25490,#25491,#25492));
#4622=EDGE_LOOP('',(#25493,#25494));
#4623=EDGE_LOOP('',(#25495,#25496,#25497,#25498,#25499,#25500));
#4624=EDGE_LOOP('',(#25501,#25502,#25503,#25504,#25505));
#4625=EDGE_LOOP('',(#25506,#25507,#25508,#25509));
#4626=EDGE_LOOP('',(#25510,#25511,#25512));
#4627=EDGE_LOOP('',(#25513,#25514,#25515,#25516,#25517,#25518,#25519,#25520,
#25521,#25522));
#4628=EDGE_LOOP('',(#25523,#25524));
#4629=EDGE_LOOP('',(#25525,#25526,#25527,#25528));
#4630=EDGE_LOOP('',(#25529,#25530,#25531));
#4631=EDGE_LOOP('',(#25532,#25533,#25534));
#4632=EDGE_LOOP('',(#25535,#25536,#25537,#25538));
#4633=EDGE_LOOP('',(#25539,#25540,#25541,#25542));
#4634=EDGE_LOOP('',(#25543,#25544,#25545,#25546));
#4635=EDGE_LOOP('',(#25547,#25548,#25549,#25550,#25551));
#4636=EDGE_LOOP('',(#25552,#25553,#25554,#25555,#25556,#25557));
#4637=EDGE_LOOP('',(#25558,#25559,#25560,#25561,#25562,#25563));
#4638=EDGE_LOOP('',(#25564,#25565,#25566,#25567,#25568,#25569,#25570,#25571,
#25572,#25573,#25574,#25575,#25576,#25577,#25578,#25579,#25580,#25581,#25582,
#25583,#25584,#25585,#25586,#25587,#25588,#25589,#25590,#25591,#25592,#25593,
#25594,#25595,#25596));
#4639=EDGE_LOOP('',(#25597,#25598,#25599,#25600,#25601,#25602));
#4640=EDGE_LOOP('',(#25603,#25604,#25605,#25606));
#4641=EDGE_LOOP('',(#25607,#25608,#25609,#25610));
#4642=EDGE_LOOP('',(#25611,#25612,#25613,#25614,#25615));
#4643=EDGE_LOOP('',(#25616,#25617,#25618,#25619,#25620));
#4644=EDGE_LOOP('',(#25621,#25622,#25623,#25624,#25625));
#4645=EDGE_LOOP('',(#25626,#25627,#25628,#25629,#25630,#25631));
#4646=EDGE_LOOP('',(#25632,#25633,#25634,#25635,#25636));
#4647=EDGE_LOOP('',(#25637,#25638,#25639,#25640));
#4648=EDGE_LOOP('',(#25641));
#4649=EDGE_LOOP('',(#25642,#25643,#25644,#25645,#25646,#25647,#25648,#25649,
#25650,#25651,#25652,#25653));
#4650=EDGE_LOOP('',(#25654,#25655,#25656,#25657,#25658,#25659,#25660,#25661,
#25662,#25663));
#4651=EDGE_LOOP('',(#25664,#25665,#25666,#25667,#25668,#25669));
#4652=EDGE_LOOP('',(#25670,#25671,#25672,#25673,#25674));
#4653=EDGE_LOOP('',(#25675,#25676,#25677));
#4654=EDGE_LOOP('',(#25678,#25679,#25680,#25681));
#4655=EDGE_LOOP('',(#25682,#25683,#25684,#25685));
#4656=EDGE_LOOP('',(#25686,#25687,#25688,#25689,#25690,#25691));
#4657=EDGE_LOOP('',(#25692,#25693,#25694,#25695));
#4658=EDGE_LOOP('',(#25696,#25697,#25698,#25699));
#4659=EDGE_LOOP('',(#25700,#25701,#25702));
#4660=EDGE_LOOP('',(#25703,#25704,#25705,#25706,#25707,#25708,#25709,#25710,
#25711,#25712));
#4661=EDGE_LOOP('',(#25713,#25714,#25715,#25716));
#4662=EDGE_LOOP('',(#25717,#25718,#25719,#25720,#25721));
#4663=EDGE_LOOP('',(#25722,#25723,#25724,#25725,#25726,#25727));
#4664=EDGE_LOOP('',(#25728,#25729,#25730,#25731,#25732,#25733));
#4665=EDGE_LOOP('',(#25734,#25735,#25736,#25737));
#4666=EDGE_LOOP('',(#25738,#25739,#25740));
#4667=EDGE_LOOP('',(#25741,#25742,#25743,#25744));
#4668=EDGE_LOOP('',(#25745,#25746,#25747,#25748,#25749,#25750));
#4669=EDGE_LOOP('',(#25751,#25752,#25753,#25754,#25755,#25756,#25757,#25758,
#25759,#25760));
#4670=EDGE_LOOP('',(#25761,#25762,#25763,#25764));
#4671=EDGE_LOOP('',(#25765,#25766,#25767,#25768));
#4672=EDGE_LOOP('',(#25769,#25770,#25771,#25772,#25773,#25774));
#4673=EDGE_LOOP('',(#25775,#25776,#25777,#25778,#25779));
#4674=EDGE_LOOP('',(#25780,#25781,#25782,#25783));
#4675=EDGE_LOOP('',(#25784,#25785,#25786));
#4676=EDGE_LOOP('',(#25787,#25788,#25789,#25790,#25791,#25792,#25793,#25794,
#25795,#25796));
#4677=EDGE_LOOP('',(#25797,#25798));
#4678=EDGE_LOOP('',(#25799,#25800,#25801,#25802));
#4679=EDGE_LOOP('',(#25803,#25804,#25805,#25806,#25807,#25808));
#4680=EDGE_LOOP('',(#25809,#25810,#25811));
#4681=EDGE_LOOP('',(#25812,#25813,#25814,#25815));
#4682=EDGE_LOOP('',(#25816,#25817,#25818,#25819));
#4683=EDGE_LOOP('',(#25820,#25821,#25822,#25823));
#4684=EDGE_LOOP('',(#25824,#25825,#25826,#25827,#25828,#25829));
#4685=EDGE_LOOP('',(#25830,#25831,#25832,#25833));
#4686=EDGE_LOOP('',(#25834,#25835,#25836,#25837));
#4687=EDGE_LOOP('',(#25838,#25839,#25840,#25841));
#4688=EDGE_LOOP('',(#25842,#25843,#25844,#25845,#25846));
#4689=EDGE_LOOP('',(#25847,#25848,#25849,#25850,#25851));
#4690=EDGE_LOOP('',(#25852,#25853,#25854,#25855,#25856));
#4691=EDGE_LOOP('',(#25857,#25858,#25859,#25860,#25861,#25862,#25863));
#4692=EDGE_LOOP('',(#25864,#25865,#25866,#25867,#25868));
#4693=EDGE_LOOP('',(#25869,#25870,#25871,#25872));
#4694=EDGE_LOOP('',(#25873,#25874,#25875,#25876,#25877,#25878,#25879,#25880,
#25881,#25882,#25883,#25884,#25885,#25886,#25887,#25888,#25889,#25890,#25891,
#25892,#25893,#25894,#25895,#25896,#25897,#25898,#25899,#25900,#25901,#25902,
#25903,#25904,#25905,#25906,#25907,#25908,#25909,#25910,#25911,#25912,#25913,
#25914,#25915,#25916,#25917,#25918,#25919,#25920,#25921,#25922,#25923,#25924,
#25925,#25926));
#4695=EDGE_LOOP('',(#25927,#25928,#25929,#25930,#25931));
#4696=EDGE_LOOP('',(#25932,#25933,#25934,#25935));
#4697=EDGE_LOOP('',(#25936,#25937,#25938,#25939));
#4698=EDGE_LOOP('',(#25940,#25941,#25942,#25943));
#4699=EDGE_LOOP('',(#25944,#25945,#25946,#25947));
#4700=EDGE_LOOP('',(#25948,#25949,#25950,#25951));
#4701=EDGE_LOOP('',(#25952,#25953,#25954,#25955));
#4702=EDGE_LOOP('',(#25956,#25957,#25958,#25959));
#4703=EDGE_LOOP('',(#25960,#25961,#25962,#25963));
#4704=EDGE_LOOP('',(#25964,#25965,#25966,#25967));
#4705=EDGE_LOOP('',(#25968,#25969,#25970,#25971));
#4706=EDGE_LOOP('',(#25972,#25973,#25974,#25975));
#4707=EDGE_LOOP('',(#25976,#25977,#25978,#25979));
#4708=EDGE_LOOP('',(#25980,#25981,#25982,#25983));
#4709=EDGE_LOOP('',(#25984,#25985,#25986,#25987));
#4710=EDGE_LOOP('',(#25988,#25989,#25990,#25991));
#4711=EDGE_LOOP('',(#25992,#25993,#25994,#25995));
#4712=EDGE_LOOP('',(#25996,#25997,#25998,#25999));
#4713=EDGE_LOOP('',(#26000,#26001,#26002,#26003));
#4714=EDGE_LOOP('',(#26004,#26005,#26006,#26007));
#4715=EDGE_LOOP('',(#26008,#26009,#26010,#26011));
#4716=EDGE_LOOP('',(#26012,#26013,#26014,#26015));
#4717=EDGE_LOOP('',(#26016,#26017,#26018,#26019));
#4718=EDGE_LOOP('',(#26020,#26021,#26022,#26023,#26024,#26025));
#4719=EDGE_LOOP('',(#26026,#26027,#26028,#26029,#26030,#26031,#26032,#26033,
#26034,#26035,#26036,#26037,#26038,#26039,#26040,#26041,#26042,#26043,#26044,
#26045,#26046,#26047,#26048,#26049,#26050,#26051,#26052,#26053,#26054,#26055,
#26056,#26057,#26058,#26059,#26060,#26061,#26062,#26063,#26064,#26065,#26066,
#26067,#26068,#26069,#26070,#26071,#26072,#26073,#26074,#26075,#26076,#26077,
#26078,#26079,#26080,#26081,#26082,#26083,#26084,#26085,#26086));
#4720=EDGE_LOOP('',(#26087,#26088,#26089,#26090,#26091,#26092));
#4721=EDGE_LOOP('',(#26093,#26094,#26095,#26096,#26097));
#4722=EDGE_LOOP('',(#26098,#26099,#26100,#26101));
#4723=EDGE_LOOP('',(#26102,#26103,#26104,#26105));
#4724=EDGE_LOOP('',(#26106,#26107,#26108,#26109));
#4725=EDGE_LOOP('',(#26110,#26111,#26112,#26113,#26114,#26115,#26116));
#4726=EDGE_LOOP('',(#26117));
#4727=EDGE_LOOP('',(#26118));
#4728=EDGE_LOOP('',(#26119,#26120,#26121,#26122));
#4729=EDGE_LOOP('',(#26123,#26124,#26125,#26126));
#4730=EDGE_LOOP('',(#26127,#26128,#26129,#26130));
#4731=EDGE_LOOP('',(#26131,#26132,#26133,#26134,#26135));
#4732=EDGE_LOOP('',(#26136,#26137,#26138,#26139,#26140,#26141,#26142,#26143,
#26144,#26145,#26146,#26147,#26148,#26149,#26150,#26151,#26152,#26153,#26154,
#26155,#26156,#26157,#26158,#26159,#26160,#26161,#26162,#26163,#26164,#26165,
#26166,#26167,#26168,#26169,#26170,#26171,#26172,#26173,#26174,#26175,#26176,
#26177,#26178,#26179,#26180,#26181,#26182,#26183,#26184,#26185,#26186,#26187,
#26188,#26189,#26190,#26191,#26192,#26193,#26194,#26195,#26196,#26197,#26198,
#26199));
#4733=EDGE_LOOP('',(#26200,#26201,#26202));
#4734=EDGE_LOOP('',(#26203,#26204,#26205,#26206));
#4735=EDGE_LOOP('',(#26207,#26208,#26209,#26210));
#4736=EDGE_LOOP('',(#26211,#26212,#26213,#26214));
#4737=EDGE_LOOP('',(#26215,#26216,#26217,#26218));
#4738=EDGE_LOOP('',(#26219,#26220,#26221,#26222));
#4739=EDGE_LOOP('',(#26223,#26224,#26225,#26226));
#4740=EDGE_LOOP('',(#26227,#26228,#26229,#26230));
#4741=EDGE_LOOP('',(#26231,#26232,#26233,#26234));
#4742=EDGE_LOOP('',(#26235,#26236,#26237,#26238));
#4743=EDGE_LOOP('',(#26239,#26240,#26241,#26242));
#4744=EDGE_LOOP('',(#26243,#26244,#26245,#26246));
#4745=EDGE_LOOP('',(#26247,#26248,#26249,#26250));
#4746=EDGE_LOOP('',(#26251,#26252,#26253,#26254));
#4747=EDGE_LOOP('',(#26255,#26256,#26257,#26258));
#4748=EDGE_LOOP('',(#26259,#26260,#26261,#26262));
#4749=EDGE_LOOP('',(#26263,#26264,#26265,#26266));
#4750=EDGE_LOOP('',(#26267,#26268,#26269,#26270));
#4751=EDGE_LOOP('',(#26271,#26272,#26273,#26274));
#4752=EDGE_LOOP('',(#26275,#26276,#26277,#26278));
#4753=EDGE_LOOP('',(#26279,#26280,#26281,#26282));
#4754=EDGE_LOOP('',(#26283,#26284,#26285,#26286));
#4755=EDGE_LOOP('',(#26287,#26288,#26289,#26290));
#4756=EDGE_LOOP('',(#26291,#26292,#26293,#26294));
#4757=EDGE_LOOP('',(#26295,#26296,#26297,#26298));
#4758=EDGE_LOOP('',(#26299,#26300,#26301,#26302));
#4759=EDGE_LOOP('',(#26303,#26304,#26305,#26306));
#4760=EDGE_LOOP('',(#26307,#26308,#26309,#26310));
#4761=EDGE_LOOP('',(#26311,#26312));
#4762=EDGE_LOOP('',(#26313,#26314,#26315,#26316,#26317,#26318,#26319,#26320,
#26321));
#4763=EDGE_LOOP('',(#26322,#26323,#26324,#26325));
#4764=EDGE_LOOP('',(#26326,#26327));
#4765=EDGE_LOOP('',(#26328,#26329));
#4766=EDGE_LOOP('',(#26330,#26331,#26332));
#7015=CIRCLE('',#40553,10.925);
#7016=CIRCLE('',#40555,10.925);
#7017=CIRCLE('',#40583,10.925);
#7018=CIRCLE('',#40585,10.0685);
#7019=CIRCLE('',#40613,1.00000000000003);
#7020=CIRCLE('',#40615,40.);
#7021=CIRCLE('',#40616,0.999999999999991);
#7022=CIRCLE('',#40618,0.999999999999996);
#7023=CIRCLE('',#40619,33.);
#7024=CIRCLE('',#40620,33.);
#7025=CIRCLE('',#40622,33.);
#7026=CIRCLE('',#40623,33.);
#7027=CIRCLE('',#40624,1.);
#7028=CIRCLE('',#40625,32.7071067811865);
#7029=CIRCLE('',#40626,32.7071067811865);
#7030=CIRCLE('',#40628,26.2928932188134);
#7031=CIRCLE('',#40629,26.2928932188134);
#7032=CIRCLE('',#40632,1.);
#7033=CIRCLE('',#40633,25.5857864376269);
#7034=CIRCLE('',#40635,17.);
#7035=CIRCLE('',#40637,17.);
#7036=CIRCLE('',#40638,17.);
#7037=CIRCLE('',#40639,1.);
#7038=CIRCLE('',#40640,16.);
#7039=CIRCLE('',#40642,14.);
#7040=CIRCLE('',#40645,14.);
#7041=CIRCLE('',#40646,14.);
#7042=CIRCLE('',#40647,1.);
#7043=CIRCLE('',#40648,13.);
#7044=CIRCLE('',#40650,0.999999999999999);
#7045=CIRCLE('',#40651,1.);
#7046=CIRCLE('',#40652,1.);
#7047=CIRCLE('',#40653,0.999999999999999);
#7048=CIRCLE('',#40654,0.999999999999999);
#7049=CIRCLE('',#40655,1.);
#7050=CIRCLE('',#40656,1.);
#7051=CIRCLE('',#40657,1.);
#7052=CIRCLE('',#40658,1.);
#7053=CIRCLE('',#40659,1.);
#7054=CIRCLE('',#40660,1.);
#7055=CIRCLE('',#40661,0.999999999999999);
#7056=CIRCLE('',#40662,1.);
#7057=CIRCLE('',#40663,1.);
#7058=CIRCLE('',#40664,1.);
#7059=CIRCLE('',#40665,1.);
#7060=CIRCLE('',#40666,0.999999999999999);
#7061=CIRCLE('',#40667,1.);
#7062=CIRCLE('',#40668,1.);
#7063=CIRCLE('',#40669,1.);
#7064=CIRCLE('',#40670,1.);
#7065=CIRCLE('',#40671,1.);
#7066=CIRCLE('',#40672,1.);
#7067=CIRCLE('',#40673,1.);
#7068=CIRCLE('',#40674,0.999999999999999);
#7069=CIRCLE('',#40675,1.);
#7070=CIRCLE('',#40676,0.999999999999999);
#7071=CIRCLE('',#40679,8.05);
#7072=CIRCLE('',#40680,0.999999999999997);
#7073=CIRCLE('',#40681,1.);
#7074=CIRCLE('',#40683,0.999999999999999);
#7075=CIRCLE('',#40684,1.);
#7076=CIRCLE('',#40686,8.05);
#7077=CIRCLE('',#40689,1.00000000000001);
#7078=CIRCLE('',#40690,29.1);
#7079=CIRCLE('',#40691,1.);
#7080=CIRCLE('',#40692,30.1);
#7081=CIRCLE('',#40694,0.999999999999998);
#7082=CIRCLE('',#40695,0.999999999999997);
#7083=CIRCLE('',#40697,0.999999999999995);
#7084=CIRCLE('',#40698,0.999999999999999);
#7085=CIRCLE('',#40699,0.999999999999997);
#7086=CIRCLE('',#40700,1.);
#7087=CIRCLE('',#40702,29.1);
#7088=CIRCLE('',#40703,0.999999999999999);
#7089=CIRCLE('',#40704,1.);
#7090=CIRCLE('',#40705,1.);
#7091=CIRCLE('',#40707,1.);
#7092=CIRCLE('',#40708,1.);
#7093=CIRCLE('',#40709,1.00000000000001);
#7094=CIRCLE('',#40710,29.1006737620246);
#7095=CIRCLE('',#40711,29.1);
#7096=CIRCLE('',#40712,29.1);
#7097=CIRCLE('',#40713,29.1);
#7098=CIRCLE('',#40714,29.1);
#7099=CIRCLE('',#40715,29.1);
#7100=CIRCLE('',#40716,29.1);
#7101=CIRCLE('',#40717,1.00000000000001);
#7102=CIRCLE('',#40718,0.999999999999995);
#7103=CIRCLE('',#40719,1.);
#7104=CIRCLE('',#40720,1.);
#7105=CIRCLE('',#40721,1.);
#7106=CIRCLE('',#40723,1.);
#7107=CIRCLE('',#40724,1.00000000000001);
#7108=CIRCLE('',#40726,29.1);
#7109=CIRCLE('',#40728,30.1);
#7110=CIRCLE('',#40730,39.);
#7111=CIRCLE('',#40731,30.1);
#7112=CIRCLE('',#40732,30.1);
#7113=CIRCLE('',#40733,30.1);
#7114=CIRCLE('',#40734,30.1);
#7115=CIRCLE('',#40736,8.05);
#7116=CIRCLE('',#40738,1.);
#7117=CIRCLE('',#40739,1.);
#7118=CIRCLE('',#40741,29.1);
#7119=CIRCLE('',#40742,0.999999999999999);
#7120=CIRCLE('',#40743,1.);
#7121=CIRCLE('',#40744,1.);
#7122=CIRCLE('',#40745,1.);
#7123=CIRCLE('',#40747,1.);
#7124=CIRCLE('',#40749,8.05);
#7125=CIRCLE('',#40750,1.);
#7126=CIRCLE('',#40751,1.);
#7127=CIRCLE('',#40752,1.);
#7128=CIRCLE('',#40753,1.);
#7129=CIRCLE('',#40755,0.999999999999996);
#7130=CIRCLE('',#40756,1.);
#7131=CIRCLE('',#40757,1.00000000000001);
#7132=CIRCLE('',#40759,29.1);
#7133=CIRCLE('',#40761,0.999999999999996);
#7134=CIRCLE('',#40762,1.);
#7135=CIRCLE('',#40763,0.999999999999996);
#7136=CIRCLE('',#40764,0.999999999999999);
#7137=CIRCLE('',#40767,29.1);
#7138=CIRCLE('',#40768,1.);
#7139=CIRCLE('',#40769,1.);
#7140=CIRCLE('',#40770,0.999999999999997);
#7141=CIRCLE('',#40772,0.999999999999996);
#7142=CIRCLE('',#40774,8.05);
#7143=CIRCLE('',#40776,1.);
#7144=CIRCLE('',#40777,0.999999999999997);
#7145=CIRCLE('',#40779,1.);
#7146=CIRCLE('',#40780,1.);
#7147=CIRCLE('',#40782,29.1);
#7148=CIRCLE('',#40784,0.999999999999997);
#7149=CIRCLE('',#40785,0.999999999999999);
#7150=CIRCLE('',#40786,1.00000000000001);
#7151=CIRCLE('',#40787,0.999999999999999);
#7152=CIRCLE('',#40791,1.);
#7153=CIRCLE('',#40793,1.);
#7154=CIRCLE('',#40794,40.);
#7155=CIRCLE('',#40795,40.);
#7156=CIRCLE('',#40798,0.999999999999999);
#7157=CIRCLE('',#40800,0.999999999999999);
#7158=CIRCLE('',#40801,1.);
#7159=CIRCLE('',#40802,0.999999999999999);
#7160=CIRCLE('',#40803,1.);
#7161=CIRCLE('',#40804,1.);
#7162=CIRCLE('',#40805,1.);
#7163=CIRCLE('',#40806,1.);
#7164=CIRCLE('',#40807,1.);
#7165=CIRCLE('',#40808,1.);
#7166=CIRCLE('',#40809,1.);
#7167=CIRCLE('',#40810,0.999999999999999);
#7168=CIRCLE('',#40811,1.);
#7169=CIRCLE('',#40812,1.);
#7170=CIRCLE('',#40813,1.);
#7171=CIRCLE('',#40814,1.);
#7172=CIRCLE('',#40815,0.999999999999999);
#7173=CIRCLE('',#40816,1.);
#7174=CIRCLE('',#40817,1.);
#7175=CIRCLE('',#40818,1.);
#7176=CIRCLE('',#40819,1.);
#7177=CIRCLE('',#40820,1.);
#7178=CIRCLE('',#40821,1.);
#7179=CIRCLE('',#40822,0.999999999999999);
#7180=CIRCLE('',#40823,0.999999999999999);
#7181=CIRCLE('',#40824,1.);
#7182=CIRCLE('',#40825,1.);
#7183=CIRCLE('',#40826,10.925);
#7184=CIRCLE('',#40850,10.6321067811865);
#7185=CIRCLE('',#40852,10.4928932188135);
#7186=CIRCLE('',#40853,10.4928932188135);
#7187=CIRCLE('',#40858,1.);
#7188=CIRCLE('',#40859,9.78578643762691);
#7189=CIRCLE('',#40861,3.5);
#7190=CIRCLE('',#40864,2.5);
#7191=CIRCLE('',#40865,1.);
#7192=CIRCLE('',#40867,2.5);
#7193=CIRCLE('',#40898,8.05);
#9424=B_SPLINE_CURVE_WITH_KNOTS('',3,(#57289,#57290,#57291,#57292),
 .UNSPECIFIED.,.F.,.F.,(4,4),(-4.09323272002468,-3.80641258671356),
 .UNSPECIFIED.);
#9425=B_SPLINE_CURVE_WITH_KNOTS('',3,(#57298,#57299,#57300,#57301,#57302,
#57303,#57304,#57305,#57306,#57307,#57308,#57309,#57310,#57311,#57312,#57313,
#57314,#57315,#57316,#57317,#57318,#57319,#57320,#57321,#57322,#57323,#57324,
#57325,#57326,#57327,#57328,#57329,#57330,#57331,#57332,#57333,#57334,#57335,
#57336,#57337,#57338,#57339,#57340),.UNSPECIFIED.,.F.,.F.,(4,3,3,3,3,3,
3,3,3,3,3,3,3,3,4),(-10.3764180272043,-10.0814246918918,-9.58269006035967,
-9.08395542882749,-8.58522079729531,-8.08648616576313,-7.58775153423096,
-7.08901690269878,-6.5902822711666,-6.09154763963442,-5.59281300810224,
-5.09407837657007,-4.59534374503789,-4.09660911350571,-4.09323272002468),
 .UNSPECIFIED.);
#9426=B_SPLINE_CURVE_WITH_KNOTS('',3,(#57343,#57344,#57345,#57346,#57347,
#57348,#57349,#57350,#57351,#57352,#57353,#57354,#57355,#57356,#57357,#57358,
#57359,#57360,#57361,#57362,#57363,#57364,#57365,#57366,#57367,#57368,#57369,
#57370,#57371,#57372,#57373,#57374,#57375,#57376,#57377,#57378,#57379),
 .UNSPECIFIED.,.F.,.F.,(4,3,3,3,3,3,3,3,3,3,3,3,4),(1.7350537127581,1.98928870769521,
2.48693807868848,2.98458744968175,3.48223682067503,3.9798861916683,4.47753556266157,
4.97518493365484,5.47283430464811,5.97048367564139,6.46813304663466,6.96578241762793,
7.40290411470023),.UNSPECIFIED.);
#9427=B_SPLINE_CURVE_WITH_KNOTS('',3,(#57384,#57385,#57386,#57387,#57388,
#57389,#57390,#57391,#57392,#57393,#57394,#57395,#57396,#57397,#57398,#57399,
#57400,#57401,#57402,#57403,#57404,#57405,#57406,#57407,#57408,#57409,#57410,
#57411,#57412,#57413,#57414,#57415,#57416,#57417,#57418,#57419,#57420,#57421,
#57422,#57423,#57424,#57425,#57426),.UNSPECIFIED.,.F.,.F.,(4,3,3,3,3,3,
3,3,3,3,3,3,3,3,4),(-16.6596033343838,-16.5649749018102,-16.066240270278,
-15.5675056387458,-15.0687710072136,-14.5700363756814,-14.0713017441493,
-13.5725671126171,-13.0738324810849,-12.5750978495527,-12.0763632180206,
-11.5776285864884,-11.0788939549562,-10.580159323424,-10.3764180272043),
 .UNSPECIFIED.);
#9428=B_SPLINE_CURVE_WITH_KNOTS('',3,(#57427,#57428,#57429,#57430,#57431,
#57432,#57433,#57434,#57435,#57436,#57437,#57438,#57439,#57440,#57441,#57442,
#57443,#57444,#57445,#57446,#57447,#57448,#57449,#57450,#57451,#57452,#57453,
#57454,#57455,#57456,#57457,#57458,#57459,#57460,#57461,#57462,#57463,#57464,
#57465,#57466,#57467,#57468,#57469),.UNSPECIFIED.,.F.,.F.,(4,3,3,3,3,3,
3,3,3,3,3,3,3,3,4),(7.40290411470023,7.4634317886212,7.96108115961447,8.45873053060775,
8.95637990160102,9.45402927259429,9.95167864358756,10.4493280145808,10.9469773855741,
11.4446267565674,11.9422761275606,12.4399254985539,12.9375748695472,13.4352242405405,
13.6860894218798),.UNSPECIFIED.);
#9429=B_SPLINE_CURVE_WITH_KNOTS('',3,(#57474,#57475,#57476,#57477,#57478,
#57479,#57480,#57481,#57482,#57483,#57484,#57485,#57486,#57487,#57488,#57489,
#57490,#57491,#57492,#57493,#57494,#57495,#57496,#57497,#57498,#57499,#57500,
#57501,#57502,#57503,#57504,#57505,#57506,#57507,#57508,#57509,#57510,#57511,
#57512,#57513),.UNSPECIFIED.,.F.,.F.,(4,3,3,3,3,3,3,3,3,3,3,3,3,4),(-22.9427886415634,
-22.5497904801963,-22.0510558486641,-21.5523212171319,-21.0535865855998,
-20.5548519540676,-20.0561173225354,-19.5573826910032,-19.058648059471,
-18.5599134279389,-18.0611787964067,-17.5624441648745,-17.0637095333423,
-16.6596033343838),.UNSPECIFIED.);
#9430=B_SPLINE_CURVE_WITH_KNOTS('',3,(#57514,#57515,#57516,#57517,#57518,
#57519,#57520,#57521,#57522,#57523,#57524,#57525,#57526,#57527,#57528,#57529,
#57530,#57531,#57532,#57533,#57534,#57535,#57536,#57537,#57538,#57539,#57540,
#57541,#57542,#57543,#57544,#57545,#57546,#57547,#57548,#57549,#57550,#57551,
#57552,#57553,#57554,#57555,#57556),.UNSPECIFIED.,.F.,.F.,(4,3,3,3,3,3,
3,3,3,3,3,3,3,3,4),(13.6860894218798,13.9328736115337,14.430522982527,14.9281723535203,
15.4258217245135,15.9234710955068,16.4211204665001,16.9187698374934,17.4164192084866,
17.9140685794799,18.4117179504732,18.9093673214664,19.4070166924597,19.904666063453,
19.9692747290594),.UNSPECIFIED.);
#9431=B_SPLINE_CURVE_WITH_KNOTS('',3,(#57561,#57562,#57563,#57564,#57565,
#57566,#57567,#57568,#57569,#57570,#57571,#57572,#57573,#57574,#57575,#57576,
#57577,#57578,#57579,#57580,#57581,#57582,#57583,#57584,#57585,#57586,#57587,
#57588,#57589,#57590,#57591,#57592,#57593,#57594,#57595,#57596,#57597,#57598,
#57599,#57600,#57601,#57602,#57603),.UNSPECIFIED.,.F.,.F.,(4,3,3,3,3,3,
3,3,3,3,3,3,3,3,4),(-29.225973948743,-29.0333406901146,-28.5346060585824,
-28.0358714270502,-27.5371367955181,-27.0384021639859,-26.5396675324537,
-26.0409329009215,-25.5421982693894,-25.0434636378572,-24.544729006325,
-24.0459943747928,-23.5472597432606,-23.0485251117285,-22.9427886415634),
 .UNSPECIFIED.);
#9432=B_SPLINE_CURVE_WITH_KNOTS('',3,(#57604,#57605,#57606,#57607,#57608,
#57609,#57610,#57611,#57612,#57613,#57614,#57615,#57616,#57617,#57618,#57619,
#57620,#57621,#57622,#57623,#57624,#57625,#57626,#57627,#57628,#57629,#57630,
#57631,#57632,#57633,#57634,#57635,#57636,#57637,#57638,#57639,#57640,#57641,
#57642,#57643),.UNSPECIFIED.,.F.,.F.,(4,3,3,3,3,3,3,3,3,3,3,3,3,4),(19.9692747290594,
20.4023154344463,20.8999648054395,21.3976141764328,21.8952635474261,22.3929129184194,
22.8905622894126,23.3882116604059,23.8858610313992,24.3835104023924,24.8811597733857,
25.378809144379,25.8764585153723,26.252460036239),.UNSPECIFIED.);
#9433=B_SPLINE_CURVE_WITH_KNOTS('',3,(#57648,#57649,#57650,#57651,#57652,
#57653,#57654,#57655,#57656,#57657,#57658,#57659,#57660,#57661,#57662,#57663,
#57664,#57665,#57666,#57667,#57668,#57669,#57670,#57671,#57672,#57673,#57674,
#57675,#57676,#57677,#57678,#57679,#57680,#57681,#57682,#57683,#57684,#57685,
#57686,#57687),.UNSPECIFIED.,.F.,.F.,(4,3,3,3,3,3,3,3,3,3,3,3,3,4),(-35.5091592559226,
-35.0181562685007,-34.5194216369686,-34.0206870054364,-33.5219523739042,
-33.023217742372,-32.5244831108399,-32.0257484793077,-31.5270138477755,
-31.0282792162433,-30.5295445847111,-30.030809953179,-29.5320753216468,
-29.225973948743),.UNSPECIFIED.);
#9434=B_SPLINE_CURVE_WITH_KNOTS('',3,(#57688,#57689,#57690,#57691,#57692,
#57693,#57694,#57695,#57696,#57697,#57698,#57699,#57700,#57701,#57702,#57703,
#57704,#57705,#57706,#57707,#57708,#57709,#57710,#57711,#57712,#57713,#57714,
#57715,#57716,#57717,#57718,#57719,#57720,#57721,#57722,#57723,#57724,#57725,
#57726,#57727,#57728,#57729,#57730),.UNSPECIFIED.,.F.,.F.,(4,3,3,3,3,3,
3,3,3,3,3,3,3,3,4),(26.252460036239,26.3741078863655,26.8717572573588,27.3694066283521,
27.8670559993454,28.3647053703386,28.8623547413319,29.3600041123252,29.8576534833185,
30.3553028543117,30.852952225305,31.3506015962983,31.8482509672916,32.3459003382848,
32.5356453434186),.UNSPECIFIED.);
#9435=B_SPLINE_CURVE_WITH_KNOTS('',3,(#57735,#57736,#57737,#57738,#57739,
#57740,#57741,#57742,#57743,#57744,#57745,#57746,#57747,#57748,#57749,#57750,
#57751,#57752,#57753,#57754,#57755,#57756,#57757,#57758,#57759,#57760,#57761,
#57762,#57763,#57764,#57765,#57766,#57767,#57768,#57769,#57770,#57771,#57772,
#57773,#57774,#57775,#57776,#57777),.UNSPECIFIED.,.F.,.F.,(4,3,3,3,3,3,
3,3,3,3,3,3,3,3,4),(-41.7923445631022,-41.501706478419,-41.0029718468869,
-40.5042372153547,-40.0055025838225,-39.5067679522903,-39.0080333207582,
-38.509298689226,-38.0105640576938,-37.5118294261616,-37.0130947946294,
-36.5143601630973,-36.0156255315651,-35.5168909000329,-35.5091592559226),
 .UNSPECIFIED.);
#9436=B_SPLINE_CURVE_WITH_KNOTS('',3,(#57778,#57779,#57780,#57781,#57782,
#57783,#57784,#57785,#57786,#57787,#57788,#57789,#57790,#57791,#57792,#57793,
#57794,#57795,#57796,#57797,#57798,#57799,#57800,#57801,#57802,#57803,#57804,
#57805,#57806,#57807,#57808,#57809,#57810,#57811,#57812,#57813,#57814,#57815,
#57816,#57817,#57818,#57819,#57820),.UNSPECIFIED.,.F.,.F.,(4,3,3,3,3,3,
3,3,3,3,3,3,3,3,4),(32.5356453434186,32.8435497092781,33.3411990802714,
33.8388484512646,34.3364978222579,34.8341471932512,35.3317965642444,35.8294459352377,
36.327095306231,36.8247446772243,37.3223940482175,37.8200434192108,38.3176927902041,
38.8153421611973,38.8188306505982),.UNSPECIFIED.);
#9437=B_SPLINE_CURVE_WITH_KNOTS('',3,(#57825,#57826,#57827,#57828,#57829,
#57830,#57831,#57832,#57833,#57834,#57835,#57836,#57837,#57838,#57839,#57840,
#57841,#57842,#57843,#57844,#57845,#57846,#57847,#57848,#57849,#57850,#57851,
#57852,#57853,#57854,#57855,#57856,#57857,#57858,#57859,#57860,#57861,#57862,
#57863,#57864,#57865,#57866,#57867),.UNSPECIFIED.,.F.,.F.,(4,3,3,3,3,3,
3,3,3,3,3,3,3,3,4),(-48.0755298702818,-47.9852566883374,-47.4865220568052,
-46.987787425273,-46.4890527937408,-45.9903181622087,-45.4915835306765,
-44.9928488991443,-44.4941142676121,-43.9953796360799,-43.4966450045478,
-42.9979103730156,-42.4991757414834,-42.0004411099512,-41.7923445631022),
 .UNSPECIFIED.);
#9438=B_SPLINE_CURVE_WITH_KNOTS('',3,(#57868,#57869,#57870,#57871,#57872,
#57873,#57874,#57875,#57876,#57877,#57878,#57879,#57880,#57881,#57882,#57883,
#57884,#57885,#57886,#57887,#57888,#57889,#57890,#57891,#57892,#57893,#57894,
#57895,#57896,#57897,#57898,#57899,#57900,#57901,#57902,#57903,#57904,#57905,
#57906,#57907),.UNSPECIFIED.,.F.,.F.,(4,3,3,3,3,3,3,3,3,3,3,3,3,4),(38.8188306505982,
39.3129915321906,39.8106409031839,40.3082902741771,40.8059396451704,41.3035890161637,
41.801238387157,42.2988877581502,42.7965371291435,43.2941865001368,43.7918358711301,
44.2894852421233,44.7871346131166,45.1020159577778),.UNSPECIFIED.);
#9439=B_SPLINE_CURVE_WITH_KNOTS('',3,(#57912,#57913,#57914,#57915,#57916,
#57917,#57918,#57919,#57920,#57921,#57922,#57923,#57924,#57925,#57926,#57927,
#57928,#57929,#57930,#57931,#57932,#57933,#57934,#57935,#57936,#57937,#57938,
#57939,#57940,#57941,#57942,#57943,#57944,#57945,#57946,#57947,#57948,#57949,
#57950,#57951),.UNSPECIFIED.,.F.,.F.,(4,3,3,3,3,3,3,3,3,3,3,3,3,4),(-54.3587151774614,
-53.9700722667235,-53.4713376351913,-52.9726030036591,-52.473868372127,
-51.9751337405948,-51.4763991090626,-50.9776644775304,-50.4789298459983,
-49.9801952144661,-49.4814605829339,-48.9827259514017,-48.4839913198695,
-48.0755298702818),.UNSPECIFIED.);
#9440=B_SPLINE_CURVE_WITH_KNOTS('',3,(#57952,#57953,#57954,#57955,#57956,
#57957,#57958,#57959,#57960,#57961,#57962,#57963,#57964,#57965,#57966,#57967,
#57968,#57969,#57970,#57971,#57972,#57973,#57974,#57975,#57976,#57977,#57978,
#57979,#57980,#57981,#57982,#57983,#57984,#57985,#57986,#57987,#57988,#57989,
#57990,#57991,#57992,#57993,#57994),.UNSPECIFIED.,.F.,.F.,(4,3,3,3,3,3,
3,3,3,3,3,3,3,3,4),(45.1020159577778,45.2847839841099,45.7824333551032,
46.2800827260964,46.7777320970897,47.275381468083,47.7730308390762,48.2706802100695,
48.7683295810628,49.2659789520561,49.7636283230493,50.2612776940426,50.7589270650359,
51.2565764360291,51.3852012649574),.UNSPECIFIED.);
#9441=B_SPLINE_CURVE_WITH_KNOTS('',3,(#57999,#58000,#58001,#58002,#58003,
#58004,#58005,#58006,#58007,#58008,#58009,#58010,#58011,#58012,#58013,#58014,
#58015,#58016,#58017,#58018,#58019,#58020,#58021,#58022,#58023,#58024,#58025,
#58026,#58027,#58028,#58029,#58030,#58031,#58032,#58033,#58034,#58035,#58036,
#58037,#58038,#58039,#58040,#58041),.UNSPECIFIED.,.F.,.F.,(4,3,3,3,3,3,
3,3,3,3,3,3,3,3,4),(-60.641900484641,-60.4536224766418,-59.9548878451096,
-59.4561532135775,-58.9574185820453,-58.4586839505131,-57.9599493189809,
-57.4612146874487,-56.9624800559166,-56.4637454243844,-55.9650107928522,
-55.46627616132,-54.9675415297879,-54.4688068982557,-54.3587151774614),
 .UNSPECIFIED.);
#9442=B_SPLINE_CURVE_WITH_KNOTS('',3,(#58042,#58043,#58044,#58045,#58046,
#58047,#58048,#58049,#58050,#58051,#58052,#58053,#58054,#58055,#58056,#58057,
#58058,#58059,#58060,#58061,#58062,#58063,#58064,#58065,#58066,#58067,#58068,
#58069,#58070,#58071,#58072,#58073,#58074,#58075,#58076,#58077,#58078,#58079,
#58080,#58081),.UNSPECIFIED.,.F.,.F.,(4,3,3,3,3,3,3,3,3,3,3,3,3,4),(51.3852012649574,
51.7542258070224,52.2518751780157,52.749524549009,53.2471739200022,53.7448232909955,
54.2424726619888,54.7401220329821,55.2377714039753,55.7354207749686,56.2330701459619,
56.7307195169552,57.2283688879484,57.6683865721369),.UNSPECIFIED.);
#9443=B_SPLINE_CURVE_WITH_KNOTS('',3,(#58086,#58087,#58088,#58089,#58090,
#58091,#58092,#58093,#58094,#58095,#58096,#58097,#58098,#58099,#58100,#58101,
#58102,#58103,#58104,#58105,#58106,#58107,#58108,#58109,#58110,#58111,#58112,
#58113,#58114,#58115,#58116,#58117,#58118,#58119,#58120,#58121,#58122,#58123,
#58124,#58125),.UNSPECIFIED.,.F.,.F.,(4,3,3,3,3,3,3,3,3,3,3,3,3,4),(-66.9250857918206,
-66.4384380550279,-65.9397034234958,-65.4409687919636,-64.9422341604314,
-64.4434995288992,-63.9447648973671,-63.4460302658349,-62.9472956343027,
-62.4485610027705,-61.9498263712383,-61.4510917397062,-60.952357108174,
-60.641900484641),.UNSPECIFIED.);
#9444=B_SPLINE_CURVE_WITH_KNOTS('',3,(#58126,#58127,#58128,#58129,#58130,
#58131,#58132,#58133,#58134,#58135,#58136,#58137,#58138,#58139,#58140,#58141,
#58142,#58143,#58144,#58145,#58146,#58147,#58148,#58149,#58150,#58151,#58152,
#58153,#58154,#58155,#58156,#58157,#58158,#58159,#58160,#58161,#58162,#58163,
#58164,#58165,#58166,#58167,#58168),.UNSPECIFIED.,.F.,.F.,(4,3,3,3,3,3,
3,3,3,3,3,3,3,3,4),(57.6683865721369,57.7260182589417,58.223667629935,58.7213170009282,
59.2189663719215,59.7166157429148,60.214265113908,60.7119144849013,61.2095638558946,
61.7072132268879,62.2048625978811,62.7025119688744,63.2001613398677,63.6978107108609,
63.9515718793165),.UNSPECIFIED.);
#9445=B_SPLINE_CURVE_WITH_KNOTS('',3,(#58173,#58174,#58175,#58176,#58177,
#58178,#58179,#58180,#58181,#58182,#58183,#58184,#58185,#58186,#58187,#58188,
#58189,#58190,#58191,#58192,#58193,#58194,#58195,#58196,#58197,#58198,#58199,
#58200,#58201,#58202,#58203,#58204,#58205,#58206,#58207,#58208,#58209,#58210,
#58211,#58212,#58213,#58214,#58215),.UNSPECIFIED.,.F.,.F.,(4,3,3,3,3,3,
3,3,3,3,3,3,3,3,4),(-73.2082710990002,-72.9219882649462,-72.4232536334141,
-71.9245190018819,-71.4257843703497,-70.9270497388175,-70.4283151072854,
-69.9295804757532,-69.430845844221,-68.9321112126888,-68.4333765811567,
-67.9346419496245,-67.4359073180923,-66.9371726865601,-66.9250857918206),
 .UNSPECIFIED.);
#9446=B_SPLINE_CURVE_WITH_KNOTS('',3,(#58216,#58217,#58218,#58219,#58220,
#58221,#58222,#58223,#58224,#58225,#58226,#58227,#58228,#58229,#58230,#58231,
#58232,#58233,#58234,#58235,#58236,#58237,#58238,#58239,#58240,#58241,#58242,
#58243,#58244,#58245,#58246,#58247,#58248,#58249,#58250,#58251,#58252,#58253,
#58254,#58255,#58256,#58257,#58258),.UNSPECIFIED.,.F.,.F.,(4,3,3,3,3,3,
3,3,3,3,3,3,3,3,4),(63.9515718793165,64.1954600818542,64.6931094528475,
65.1907588238408,65.688408194834,66.1860575658273,66.6837069368206,67.1813563078139,
67.6790056788071,68.1766550498004,68.6743044207937,69.1719537917869,69.6696031627802,
70.1672525337735,70.2347571864961),.UNSPECIFIED.);
#9447=B_SPLINE_CURVE_WITH_KNOTS('',3,(#58263,#58264,#58265,#58266,#58267,
#58268,#58269,#58270,#58271,#58272,#58273,#58274,#58275,#58276,#58277,#58278,
#58279,#58280,#58281,#58282,#58283,#58284,#58285,#58286,#58287,#58288,#58289,
#58290,#58291,#58292,#58293,#58294,#58295,#58296,#58297,#58298,#58299,#58300,
#58301,#58302,#58303,#58304,#58305),.UNSPECIFIED.,.F.,.F.,(4,3,3,3,3,3,
3,3,3,3,3,3,3,3,4),(-79.4914564061798,-79.4055384748646,-78.9068038433324,
-78.4080692118002,-77.9093345802681,-77.4105999487359,-76.9118653172037,
-76.4131306856715,-75.9143960541393,-75.4156614226072,-74.916926791075,
-74.4181921595428,-73.9194575280106,-73.4207228964784,-73.2082710990002),
 .UNSPECIFIED.);
#9448=B_SPLINE_CURVE_WITH_KNOTS('',3,(#58306,#58307,#58308,#58309,#58310,
#58311,#58312,#58313,#58314,#58315,#58316,#58317,#58318,#58319,#58320,#58321,
#58322,#58323,#58324,#58325,#58326,#58327,#58328,#58329,#58330,#58331,#58332,
#58333,#58334,#58335,#58336,#58337,#58338,#58339,#58340,#58341,#58342,#58343,
#58344,#58345),.UNSPECIFIED.,.F.,.F.,(4,3,3,3,3,3,3,3,3,3,3,3,3,4),(70.2347571864961,
70.6649019047668,71.16255127576,71.6602006467533,72.1578500177466,72.6554993887399,
73.1531487597331,73.6507981307264,74.1484475017197,74.6460968727129,75.1437462437062,
75.6413956146995,76.1390449856927,76.5179424936757),.UNSPECIFIED.);
#9449=B_SPLINE_CURVE_WITH_KNOTS('',3,(#58350,#58351,#58352,#58353,#58354,
#58355,#58356,#58357,#58358,#58359,#58360,#58361,#58362,#58363,#58364,#58365,
#58366,#58367,#58368,#58369,#58370,#58371,#58372,#58373,#58374,#58375,#58376,
#58377,#58378,#58379,#58380,#58381,#58382,#58383,#58384,#58385,#58386,#58387,
#58388,#58389),.UNSPECIFIED.,.F.,.F.,(4,3,3,3,3,3,3,3,3,3,3,3,3,4),(-85.7746417133593,
-85.3903540532507,-84.8916194217185,-84.3928847901863,-83.8941501586542,
-83.395415527122,-82.8966808955898,-82.3979462640577,-81.8992116325255,
-81.4004770009933,-80.9017423694611,-80.4030077379289,-79.9042731063968,
-79.4914564061798),.UNSPECIFIED.);
#9450=B_SPLINE_CURVE_WITH_KNOTS('',3,(#58390,#58391,#58392,#58393,#58394,
#58395,#58396,#58397,#58398,#58399,#58400,#58401,#58402,#58403,#58404,#58405,
#58406,#58407,#58408,#58409,#58410,#58411,#58412,#58413,#58414,#58415,#58416,
#58417,#58418,#58419,#58420,#58421,#58422,#58423,#58424,#58425,#58426,#58427,
#58428,#58429,#58430,#58431,#58432),.UNSPECIFIED.,.F.,.F.,(4,3,3,3,3,3,
3,3,3,3,3,3,3,3,4),(76.5179424936757,76.636694356686,77.1343437276793,77.6319930986726,
78.1296424696659,78.6272918406591,79.1249412116524,79.6225905826457,80.1202399536389,
80.6178893246322,81.1155386956255,81.6131880666188,82.110837437612,82.6084868086053,
82.8011278008553),.UNSPECIFIED.);
#9451=B_SPLINE_CURVE_WITH_KNOTS('',3,(#58437,#58438,#58439,#58440,#58441,
#58442,#58443,#58444,#58445,#58446,#58447,#58448,#58449,#58450,#58451,#58452,
#58453,#58454,#58455,#58456,#58457,#58458,#58459,#58460,#58461,#58462,#58463,
#58464,#58465,#58466,#58467,#58468,#58469,#58470,#58471,#58472,#58473,#58474,
#58475,#58476,#58477,#58478,#58479),.UNSPECIFIED.,.F.,.F.,(4,3,3,3,3,3,
3,3,3,3,3,3,3,3,4),(-92.057827020539,-91.873904263169,-91.3751696316368,
-90.8764350001046,-90.3777003685725,-89.8789657370403,-89.3802311055081,
-88.881496473976,-88.3827618424438,-87.8840272109116,-87.3852925793794,
-86.8865579478472,-86.387823316315,-85.8890886847829,-85.7746417133593),
 .UNSPECIFIED.);
#9452=B_SPLINE_CURVE_WITH_KNOTS('',3,(#58480,#58481,#58482,#58483,#58484,
#58485,#58486,#58487,#58488,#58489,#58490,#58491,#58492,#58493,#58494,#58495,
#58496,#58497,#58498,#58499,#58500,#58501,#58502,#58503,#58504,#58505,#58506,
#58507,#58508,#58509,#58510,#58511,#58512,#58513,#58514,#58515,#58516,#58517,
#58518,#58519,#58520,#58521,#58522),.UNSPECIFIED.,.F.,.F.,(4,3,3,3,3,3,
3,3,3,3,3,3,3,3,4),(82.8011278008553,83.1061361795986,83.6037855505919,
84.1014349215851,84.5990842925784,85.0967336635717,85.5943830345649,86.0920324055582,
86.5896817765515,87.0873311475448,87.584980518538,88.0826298895313,88.5802792605246,
89.0779286315178,89.0843131080349),.UNSPECIFIED.);
#9453=B_SPLINE_CURVE_WITH_KNOTS('',3,(#58527,#58528,#58529,#58530,#58531,
#58532,#58533,#58534,#58535,#58536,#58537,#58538,#58539,#58540,#58541,#58542,
#58543,#58544,#58545,#58546,#58547,#58548,#58549,#58550,#58551,#58552,#58553,
#58554,#58555,#58556,#58557,#58558,#58559,#58560,#58561,#58562,#58563,#58564,
#58565,#58566),.UNSPECIFIED.,.F.,.F.,(4,3,3,3,3,3,3,3,3,3,3,3,3,4),(-98.3410123277185,
-97.8587198415551,-97.359985210023,-96.8612505784908,-96.3625159469586,
-95.8637813154264,-95.3650466838943,-94.8663120523621,-94.3675774208299,
-93.8688427892977,-93.3701081577655,-92.8713735262334,-92.3726388947012,
-92.057827020539),.UNSPECIFIED.);
#9454=B_SPLINE_CURVE_WITH_KNOTS('',3,(#58567,#58568,#58569,#58570,#58571,
#58572,#58573,#58574,#58575,#58576,#58577,#58578,#58579,#58580,#58581,#58582,
#58583,#58584,#58585,#58586,#58587,#58588,#58589,#58590,#58591,#58592,#58593,
#58594,#58595,#58596,#58597,#58598,#58599,#58600,#58601,#58602,#58603,#58604,
#58605,#58606),.UNSPECIFIED.,.F.,.F.,(4,3,3,3,3,3,3,3,3,3,3,3,3,4),(89.0843131080349,
89.5755780025111,90.0732273735044,90.5708767444977,91.0685261154909,91.5661754864842,
92.0638248574775,92.5614742284707,93.059123599464,93.5567729704573,94.0544223414506,
94.5520717124438,95.0497210834371,95.3674984152145),.UNSPECIFIED.);
#9455=B_SPLINE_CURVE_WITH_KNOTS('',3,(#58611,#58612,#58613,#58614,#58615,
#58616,#58617,#58618,#58619,#58620,#58621,#58622,#58623,#58624,#58625,#58626,
#58627,#58628,#58629,#58630,#58631,#58632,#58633,#58634,#58635,#58636,#58637,
#58638,#58639,#58640,#58641,#58642,#58643,#58644,#58645,#58646,#58647,#58648,
#58649,#58650,#58651,#58652,#58653),.UNSPECIFIED.,.F.,.F.,(4,3,3,3,3,3,
3,3,3,3,3,3,3,3,4),(-104.624197634898,-104.342270051473,-103.843535419941,
-103.344800788409,-102.846066156877,-102.347331525345,-101.848596893813,
-101.34986226228,-100.851127630748,-100.352392999216,-99.8536583676838,
-99.3549237361517,-98.8561891046195,-98.3574544730873,-98.3410123277185),
 .UNSPECIFIED.);
#9456=B_SPLINE_CURVE_WITH_KNOTS('',3,(#58654,#58655,#58656,#58657,#58658,
#58659,#58660,#58661,#58662,#58663,#58664,#58665,#58666,#58667,#58668,#58669,
#58670,#58671,#58672,#58673,#58674,#58675,#58676,#58677,#58678,#58679,#58680,
#58681,#58682,#58683,#58684,#58685,#58686,#58687,#58688,#58689,#58690,#58691,
#58692,#58693,#58694,#58695,#58696),.UNSPECIFIED.,.F.,.F.,(4,3,3,3,3,3,
3,3,3,3,3,3,3,3,4),(95.3674984152145,95.5473704544304,96.0450198254237,
96.5426691964169,97.0403185674102,97.5379679384035,98.0356173093967,98.53326668039,
99.0309160513833,99.5285654223766,100.02621479337,100.523864164363,101.021513535356,
101.51916290635,101.650683722394),.UNSPECIFIED.);
#9457=B_SPLINE_CURVE_WITH_KNOTS('',3,(#58701,#58702,#58703,#58704,#58705,
#58706,#58707,#58708,#58709,#58710,#58711,#58712,#58713,#58714,#58715,#58716,
#58717,#58718,#58719,#58720,#58721,#58722,#58723,#58724,#58725,#58726,#58727,
#58728,#58729,#58730,#58731,#58732,#58733,#58734,#58735,#58736,#58737,#58738,
#58739,#58740,#58741,#58742,#58743),.UNSPECIFIED.,.F.,.F.,(4,3,3,3,3,3,
3,3,3,3,3,3,3,3,4),(-110.907382942078,-110.825820261392,-110.32708562986,
-109.828350998327,-109.329616366795,-108.830881735263,-108.332147103731,
-107.833412472199,-107.334677840667,-106.835943209134,-106.337208577602,
-105.83847394607,-105.339739314538,-104.841004683006,-104.624197634898),
 .UNSPECIFIED.);
#9458=B_SPLINE_CURVE_WITH_KNOTS('',3,(#58744,#58745,#58746,#58747,#58748,
#58749,#58750,#58751,#58752,#58753,#58754,#58755,#58756,#58757,#58758,#58759,
#58760,#58761,#58762,#58763,#58764,#58765,#58766,#58767,#58768,#58769,#58770,
#58771,#58772,#58773,#58774,#58775,#58776,#58777,#58778,#58779,#58780,#58781,
#58782,#58783),.UNSPECIFIED.,.F.,.F.,(4,3,3,3,3,3,3,3,3,3,3,3,3,4),(101.650683722394,
102.016812277343,102.514461648336,103.012111019329,103.509760390323,104.007409761316,
104.505059132309,105.002708503303,105.500357874296,105.998007245289,106.495656616282,
106.993305987276,107.490955358269,107.933869029574),.UNSPECIFIED.);
#9459=B_SPLINE_CURVE_WITH_KNOTS('',3,(#58788,#58789,#58790,#58791,#58792,
#58793,#58794,#58795,#58796,#58797,#58798,#58799,#58800,#58801,#58802,#58803,
#58804,#58805,#58806,#58807,#58808,#58809,#58810,#58811,#58812,#58813,#58814,
#58815,#58816,#58817,#58818,#58819,#58820,#58821,#58822,#58823,#58824,#58825,
#58826,#58827),.UNSPECIFIED.,.F.,.F.,(4,3,3,3,3,3,3,3,3,3,3,3,3,4),(-117.190568249257,
-116.810635839778,-116.311901208246,-115.813166576714,-115.314431945181,
-114.815697313649,-114.316962682117,-113.818228050585,-113.319493419053,
-112.82075878752,-112.322024155988,-111.823289524456,-111.324554892924,
-110.907382942078),.UNSPECIFIED.);
#9460=B_SPLINE_CURVE_WITH_KNOTS('',3,(#58828,#58829,#58830,#58831,#58832,
#58833,#58834,#58835,#58836,#58837,#58838,#58839,#58840,#58841,#58842,#58843,
#58844,#58845,#58846,#58847,#58848,#58849,#58850,#58851,#58852,#58853,#58854,
#58855,#58856,#58857,#58858,#58859,#58860,#58861,#58862,#58863,#58864,#58865,
#58866,#58867,#58868,#58869,#58870),.UNSPECIFIED.,.F.,.F.,(4,3,3,3,3,3,
3,3,3,3,3,3,3,3,4),(107.933869029574,107.988604729262,108.486254100255,
108.983903471249,109.481552842242,109.979202213235,110.476851584229,110.974500955222,
111.472150326215,111.969799697208,112.467449068202,112.965098439195,113.462747810188,
113.960397181181,114.217054336753),.UNSPECIFIED.);
#9461=B_SPLINE_CURVE_WITH_KNOTS('',3,(#58875,#58876,#58877,#58878,#58879,
#58880,#58881,#58882,#58883,#58884,#58885,#58886,#58887,#58888,#58889,#58890,
#58891,#58892,#58893,#58894,#58895,#58896,#58897,#58898,#58899,#58900,#58901,
#58902,#58903,#58904,#58905,#58906,#58907,#58908,#58909,#58910,#58911,#58912,
#58913,#58914,#58915,#58916,#58917),.UNSPECIFIED.,.F.,.F.,(4,3,3,3,3,3,
3,3,3,3,3,3,3,3,4),(-123.473753556437,-123.294186049696,-122.795451418164,
-122.296716786632,-121.7979821551,-121.299247523568,-120.800512892035,-120.301778260503,
-119.803043628971,-119.304308997439,-118.805574365907,-118.306839734374,
-117.808105102842,-117.30937047131,-117.190568249257),.UNSPECIFIED.);
#9462=B_SPLINE_CURVE_WITH_KNOTS('',3,(#58918,#58919,#58920,#58921,#58922,
#58923,#58924,#58925,#58926,#58927,#58928,#58929,#58930,#58931,#58932,#58933,
#58934,#58935,#58936,#58937,#58938,#58939,#58940,#58941,#58942,#58943,#58944,
#58945,#58946,#58947,#58948,#58949,#58950,#58951,#58952,#58953,#58954,#58955,
#58956,#58957,#58958,#58959,#58960),.UNSPECIFIED.,.F.,.F.,(4,3,3,3,3,3,
3,3,3,3,3,3,3,3,4),(114.217054336753,114.458046552175,114.955695923168,
115.453345294161,115.950994665155,116.448644036148,116.946293407141,117.443942778134,
117.941592149128,118.439241520121,118.936890891114,119.434540262107,119.932189633101,
120.429839004094,120.500239643933),.UNSPECIFIED.);
#9463=B_SPLINE_CURVE_WITH_KNOTS('',3,(#58965,#58966,#58967,#58968,#58969,
#58970,#58971,#58972,#58973,#58974,#58975,#58976,#58977,#58978,#58979,#58980,
#58981,#58982,#58983,#58984,#58985,#58986,#58987,#58988,#58989,#58990,#58991,
#58992,#58993,#58994,#58995,#58996,#58997,#58998,#58999,#59000,#59001,#59002,
#59003,#59004),.UNSPECIFIED.,.F.,.F.,(4,3,3,3,3,3,3,3,3,3,3,3,3,4),(-129.756938863617,
-129.279001628082,-128.78026699655,-128.281532365018,-127.782797733486,
-127.284063101954,-126.785328470421,-126.286593838889,-125.787859207357,
-125.289124575825,-124.790389944293,-124.291655312761,-123.792920681228,
-123.473753556437),.UNSPECIFIED.);
#9464=B_SPLINE_CURVE_WITH_KNOTS('',3,(#59005,#59006,#59007,#59008,#59009,
#59010,#59011,#59012,#59013,#59014,#59015,#59016,#59017,#59018,#59019,#59020,
#59021,#59022,#59023,#59024,#59025,#59026,#59027,#59028,#59029,#59030,#59031,
#59032,#59033,#59034,#59035,#59036,#59037,#59038,#59039,#59040,#59041,#59042,
#59043,#59044),.UNSPECIFIED.,.F.,.F.,(4,3,3,3,3,3,3,3,3,3,3,3,3,4),(120.500239643933,
120.927488375087,121.425137746081,121.922787117074,122.420436488067,122.91808585906,
123.415735230054,123.913384601047,124.41103397204,124.908683343033,125.406332714027,
125.90398208502,126.401631456013,126.783424951112),.UNSPECIFIED.);
#9465=B_SPLINE_CURVE_WITH_KNOTS('',3,(#59049,#59050,#59051,#59052,#59053,
#59054,#59055,#59056,#59057,#59058,#59059,#59060,#59061,#59062,#59063,#59064,
#59065,#59066,#59067,#59068,#59069,#59070,#59071,#59072,#59073,#59074,#59075,
#59076,#59077,#59078,#59079,#59080,#59081,#59082,#59083,#59084,#59085,#59086,
#59087,#59088,#59089,#59090,#59091),.UNSPECIFIED.,.F.,.F.,(4,3,3,3,3,3,
3,3,3,3,3,3,3,3,4),(-136.040124170796,-135.762551838001,-135.263817206469,
-134.765082574936,-134.266347943404,-133.767613311872,-133.26887868034,
-132.770144048808,-132.271409417275,-131.772674785743,-131.273940154211,
-130.775205522679,-130.276470891147,-129.777736259615,-129.756938863617),
 .UNSPECIFIED.);
#9466=B_SPLINE_CURVE_WITH_KNOTS('',3,(#59092,#59093,#59094,#59095,#59096,
#59097,#59098,#59099,#59100,#59101,#59102,#59103,#59104,#59105,#59106,#59107,
#59108,#59109,#59110,#59111,#59112,#59113,#59114,#59115,#59116,#59117,#59118,
#59119,#59120,#59121,#59122,#59123,#59124,#59125,#59126,#59127,#59128,#59129,
#59130,#59131,#59132,#59133,#59134),.UNSPECIFIED.,.F.,.F.,(4,3,3,3,3,3,
3,3,3,3,3,3,3,3,4),(126.783424951112,126.899280827007,127.396930198,127.894579568993,
128.392228939986,128.88987831098,129.387527681973,129.885177052966,130.382826423959,
130.880475794953,131.378125165946,131.875774536939,132.373423907933,132.871073278926,
133.066610258292),.UNSPECIFIED.);
#9467=B_SPLINE_CURVE_WITH_KNOTS('',3,(#59139,#59140,#59141,#59142,#59143,
#59144,#59145,#59146,#59147,#59148,#59149,#59150,#59151,#59152,#59153,#59154,
#59155,#59156,#59157,#59158,#59159,#59160,#59161,#59162,#59163,#59164,#59165,
#59166,#59167,#59168,#59169,#59170,#59171,#59172,#59173,#59174,#59175,#59176,
#59177,#59178,#59179,#59180,#59181),.UNSPECIFIED.,.F.,.F.,(4,3,3,3,3,3,
3,3,3,3,3,3,3,3,4),(-142.323309477976,-142.246102047919,-141.747367416387,
-141.248632784855,-140.749898153322,-140.25116352179,-139.752428890258,
-139.253694258726,-138.754959627194,-138.256224995662,-137.757490364129,
-137.258755732597,-136.760021101065,-136.261286469533,-136.040124170796),
 .UNSPECIFIED.);
#9468=B_SPLINE_CURVE_WITH_KNOTS('',3,(#59182,#59183,#59184,#59185,#59186,
#59187,#59188,#59189,#59190,#59191,#59192,#59193,#59194,#59195,#59196,#59197,
#59198,#59199,#59200,#59201,#59202,#59203,#59204,#59205,#59206,#59207,#59208,
#59209,#59210,#59211,#59212,#59213,#59214,#59215,#59216,#59217,#59218,#59219,
#59220,#59221,#59222,#59223,#59224),.UNSPECIFIED.,.F.,.F.,(4,3,3,3,3,3,
3,3,3,3,3,3,3,3,4),(133.066610258292,133.368722649919,133.866372020912,
134.364021391906,134.861670762899,135.359320133892,135.856969504885,136.354618875879,
136.852268246872,137.349917617865,137.847566988859,138.345216359852,138.842865730845,
139.340515101838,139.349795565472),.UNSPECIFIED.);
#9469=B_SPLINE_CURVE_WITH_KNOTS('',3,(#59229,#59230,#59231,#59232,#59233,
#59234,#59235,#59236,#59237,#59238,#59239,#59240,#59241,#59242,#59243,#59244,
#59245,#59246,#59247,#59248,#59249,#59250,#59251,#59252,#59253,#59254,#59255,
#59256,#59257,#59258,#59259,#59260,#59261,#59262,#59263,#59264,#59265,#59266,
#59267,#59268),.UNSPECIFIED.,.F.,.F.,(4,3,3,3,3,3,3,3,3,3,3,3,3,4),(-148.606494785155,
-148.230917626305,-147.732182994773,-147.233448363241,-146.734713731709,
-146.235979100176,-145.737244468644,-145.238509837112,-144.73977520558,
-144.241040574048,-143.742305942516,-143.243571310983,-142.744836679451,
-142.323309477976),.UNSPECIFIED.);
#9470=B_SPLINE_CURVE_WITH_KNOTS('',3,(#59269,#59270,#59271,#59272,#59273,
#59274,#59275,#59276,#59277,#59278,#59279,#59280,#59281,#59282,#59283,#59284,
#59285,#59286,#59287,#59288,#59289,#59290,#59291,#59292,#59293,#59294,#59295,
#59296,#59297,#59298,#59299,#59300,#59301,#59302,#59303,#59304,#59305,#59306,
#59307,#59308),.UNSPECIFIED.,.F.,.F.,(4,3,3,3,3,3,3,3,3,3,3,3,3,4),(139.349795565472,
139.838164472832,140.335813843825,140.833463214818,141.331112585811,141.828761956805,
142.326411327798,142.824060698791,143.321710069785,143.819359440778,144.317008811771,
144.814658182764,145.312307553758,145.632980872651),.UNSPECIFIED.);
#9471=B_SPLINE_CURVE_WITH_KNOTS('',3,(#59313,#59314,#59315,#59316,#59317,
#59318,#59319,#59320,#59321,#59322,#59323,#59324,#59325,#59326,#59327,#59328,
#59329,#59330,#59331,#59332,#59333,#59334,#59335,#59336,#59337,#59338,#59339,
#59340,#59341,#59342,#59343,#59344,#59345,#59346,#59347,#59348,#59349,#59350,
#59351,#59352,#59353,#59354,#59355),.UNSPECIFIED.,.F.,.F.,(4,3,3,3,3,3,
3,3,3,3,3,3,3,3,4),(-154.889680092335,-154.714467836223,-154.215733204691,
-153.716998573159,-153.218263941627,-152.719529310095,-152.220794678563,
-151.72206004703,-151.223325415498,-150.724590783966,-150.225856152434,
-149.727121520902,-149.228386889369,-148.729652257837,-148.606494785155),
 .UNSPECIFIED.);
#9472=B_SPLINE_CURVE_WITH_KNOTS('',3,(#59356,#59357,#59358,#59359,#59360,
#59361,#59362,#59363,#59364,#59365,#59366,#59367,#59368,#59369,#59370,#59371,
#59372,#59373,#59374,#59375,#59376,#59377,#59378,#59379,#59380,#59381,#59382,
#59383,#59384,#59385,#59386,#59387,#59388,#59389,#59390,#59391,#59392,#59393,
#59394,#59395,#59396,#59397,#59398),.UNSPECIFIED.,.F.,.F.,(4,3,3,3,3,3,
3,3,3,3,3,3,3,3,4),(145.632980872651,145.809956924751,146.307606295744,
146.805255666737,147.302905037731,147.800554408724,148.298203779717,148.795853150711,
149.293502521704,149.791151892697,150.28880126369,150.786450634684,151.284100005677,
151.78174937667,151.916166179831),.UNSPECIFIED.);
#9473=B_SPLINE_CURVE_WITH_KNOTS('',3,(#59403,#59404,#59405,#59406,#59407,
#59408,#59409,#59410,#59411,#59412,#59413,#59414,#59415,#59416,#59417,#59418,
#59419,#59420,#59421,#59422,#59423,#59424,#59425,#59426,#59427,#59428,#59429,
#59430,#59431,#59432,#59433,#59434,#59435,#59436,#59437,#59438,#59439,#59440,
#59441,#59442),.UNSPECIFIED.,.F.,.F.,(4,3,3,3,3,3,3,3,3,3,3,3,3,4),(-161.172865399514,
-160.69928341461,-160.200548783077,-159.701814151545,-159.203079520013,
-158.704344888481,-158.205610256949,-157.706875625417,-157.208140993884,
-156.709406362352,-156.21067173082,-155.711937099288,-155.213202467756,
-154.889680092335),.UNSPECIFIED.);
#9474=B_SPLINE_CURVE_WITH_KNOTS('',3,(#59443,#59444,#59445,#59446,#59447,
#59448,#59449,#59450,#59451,#59452,#59453,#59454,#59455,#59456,#59457,#59458,
#59459,#59460,#59461,#59462,#59463,#59464,#59465,#59466,#59467,#59468,#59469,
#59470,#59471,#59472,#59473,#59474,#59475,#59476,#59477,#59478,#59479,#59480,
#59481,#59482),.UNSPECIFIED.,.F.,.F.,(4,3,3,3,3,3,3,3,3,3,3,3,3,4),(151.916166179831,
152.279398747663,152.777048118657,153.27469748965,153.772346860643,154.269996231636,
154.76764560263,155.265294973623,155.762944344616,156.26059371561,156.758243086603,
157.255892457596,157.753541828589,158.19935148701),.UNSPECIFIED.);
#9475=B_SPLINE_CURVE_WITH_KNOTS('',3,(#59487,#59488,#59489,#59490,#59491,
#59492,#59493,#59494,#59495,#59496,#59497,#59498,#59499,#59500,#59501,#59502,
#59503,#59504,#59505,#59506,#59507,#59508,#59509,#59510,#59511,#59512,#59513,
#59514,#59515,#59516,#59517,#59518,#59519,#59520,#59521,#59522,#59523,#59524,
#59525,#59526,#59527,#59528,#59529),.UNSPECIFIED.,.F.,.F.,(4,3,3,3,3,3,
3,3,3,3,3,3,3,3,4),(-167.456050706694,-167.182833624528,-166.684098992996,
-166.185364361464,-165.686629729931,-165.187895098399,-164.689160466867,
-164.190425835335,-163.691691203803,-163.19295657227,-162.694221940738,
-162.195487309206,-161.696752677674,-161.198018046142,-161.172865399514),
 .UNSPECIFIED.);
#9476=B_SPLINE_CURVE_WITH_KNOTS('',3,(#59530,#59531,#59532,#59533,#59534,
#59535,#59536,#59537,#59538,#59539,#59540,#59541,#59542,#59543,#59544,#59545,
#59546,#59547,#59548,#59549,#59550,#59551,#59552,#59553,#59554,#59555,#59556,
#59557,#59558,#59559,#59560,#59561,#59562,#59563,#59564,#59565,#59566,#59567,
#59568,#59569,#59570,#59571,#59572),.UNSPECIFIED.,.F.,.F.,(4,3,3,3,3,3,
3,3,3,3,3,3,3,3,4),(158.19935148701,158.251191199583,158.748840570576,159.246489941569,
159.744139312562,160.241788683556,160.739438054549,161.237087425542,161.734736796536,
162.232386167529,162.730035538522,163.227684909515,163.725334280509,164.222983651502,
164.48253679419),.UNSPECIFIED.);
#9477=B_SPLINE_CURVE_WITH_KNOTS('',3,(#59577,#59578,#59579,#59580,#59581,
#59582,#59583,#59584,#59585,#59586,#59587,#59588,#59589,#59590,#59591,#59592,
#59593,#59594,#59595,#59596,#59597,#59598,#59599,#59600,#59601,#59602,#59603,
#59604,#59605,#59606,#59607,#59608,#59609,#59610,#59611,#59612,#59613,#59614,
#59615,#59616,#59617,#59618,#59619),.UNSPECIFIED.,.F.,.F.,(4,3,3,3,3,3,
3,3,3,3,3,3,3,3,4),(-173.739236013873,-173.666383834446,-173.167649202914,
-172.668914571382,-172.17017993985,-171.671445308317,-171.172710676785,
-170.673976045253,-170.175241413721,-169.676506782189,-169.177772150657,
-168.679037519124,-168.180302887592,-167.68156825606,-167.456050706694),
 .UNSPECIFIED.);
#9478=B_SPLINE_CURVE_WITH_KNOTS('',3,(#59620,#59621,#59622,#59623,#59624,
#59625,#59626,#59627,#59628,#59629,#59630,#59631,#59632,#59633,#59634,#59635,
#59636,#59637,#59638,#59639,#59640,#59641,#59642,#59643,#59644,#59645,#59646,
#59647,#59648,#59649,#59650,#59651,#59652,#59653,#59654,#59655,#59656,#59657,
#59658,#59659,#59660,#59661,#59662),.UNSPECIFIED.,.F.,.F.,(4,3,3,3,3,3,
3,3,3,3,3,3,3,3,4),(164.48253679419,164.720633022495,165.218282393488,165.715931764482,
166.213581135475,166.711230506468,167.208879877462,167.706529248455,168.204178619448,
168.701827990441,169.199477361435,169.697126732428,170.194776103421,170.692425474415,
170.765722101369),.UNSPECIFIED.);
#9479=B_SPLINE_CURVE_WITH_KNOTS('',3,(#59669,#59670,#59671,#59672,#59673,
#59674,#59675,#59676,#59677,#59678,#59679,#59680,#59681,#59682,#59683,#59684,
#59685,#59686,#59687,#59688,#59689,#59690,#59691,#59692,#59693,#59694,#59695,
#59696,#59697,#59698,#59699,#59700,#59701,#59702),.UNSPECIFIED.,.F.,.F.,
(4,3,3,3,3,3,3,3,3,3,3,4),(-179.1524647813,-178.653730149768,-178.154995518236,
-177.656260886704,-177.157526255171,-176.658791623639,-176.160056992107,
-175.661322360575,-175.162587729043,-174.663853097511,-174.165118465978,
-173.739236013873),.UNSPECIFIED.);
#9480=B_SPLINE_CURVE_WITH_KNOTS('',3,(#59703,#59704,#59705,#59706,#59707,
#59708,#59709,#59710,#59711,#59712,#59713,#59714,#59715,#59716,#59717,#59718,
#59719,#59720,#59721,#59722,#59723,#59724,#59725,#59726,#59727,#59728,#59729,
#59730,#59731,#59732,#59733,#59734,#59735,#59736,#59737,#59738,#59739,#59740,
#59741,#59742),.UNSPECIFIED.,.F.,.F.,(4,3,3,3,3,3,3,3,3,3,3,3,3,4),(170.765722101369,
171.190074845408,171.687724216401,172.185373587394,172.683022958388,173.180672329381,
173.678321700374,174.175971071367,174.673620442361,175.171269813354,175.668919184347,
176.166568555341,176.664217926334,177.048907408549),.UNSPECIFIED.);
#9481=B_SPLINE_CURVE_WITH_KNOTS('',3,(#59748,#59749,#59750,#59751,#59752,
#59753,#59754,#59755,#59756,#59757),.UNSPECIFIED.,.F.,.F.,(4,1,1,1,1,1,
1,4),(185.353966561798,185.779849013903,186.278583645435,186.777318276967,
187.276052908499,187.774787540031,188.273522171564,188.695836455269),
 .UNSPECIFIED.);
#9482=B_SPLINE_CURVE_WITH_KNOTS('',3,(#59760,#59761,#59762,#59763,#59764,
#59765,#59766,#59767),.UNSPECIFIED.,.F.,.F.,(4,1,1,1,1,4),(185.353966561798,
185.466926450576,185.964575821569,186.462225192562,186.959874563556,187.457523934549),
 .UNSPECIFIED.);
#9483=B_SPLINE_CURVE_WITH_KNOTS('',3,(#59772,#59773,#59774,#59775,#59776,
#59777,#59778,#59779,#59780,#59781,#59782,#59783,#59784,#59785,#59786,#59787,
#59788),.UNSPECIFIED.,.F.,.F.,(4,1,1,1,1,1,1,1,1,1,1,1,1,1,4),(179.070781254618,
179.296298803984,179.795033435517,180.293768067049,180.792502698581,181.291237330113,
181.789971961645,182.288706593177,182.78744122471,183.286175856242,183.784910487774,
184.283645119306,184.782379750838,185.281114382371,185.353966561798),
 .UNSPECIFIED.);
#9484=B_SPLINE_CURVE_WITH_KNOTS('',3,(#59789,#59790,#59791,#59792,#59793,
#59794,#59795,#59796,#59797,#59798,#59799,#59800,#59801,#59802,#59803,#59804),
 .UNSPECIFIED.,.F.,.F.,(4,1,1,1,1,1,1,1,1,1,1,1,1,4),(179.070781254618,
179.495133998657,179.99278336965,180.490432740643,180.988082111636,181.48573148263,
181.983380853623,182.481030224616,182.97867959561,183.476328966603,183.973978337596,
184.471627708589,184.969277079583,185.353966561798),.UNSPECIFIED.);
#9485=B_SPLINE_CURVE_WITH_KNOTS('',3,(#59809,#59810,#59811,#59812,#59813,
#59814,#59815,#59816,#59817,#59818,#59819,#59820,#59821,#59822,#59823,#59824,
#59825),.UNSPECIFIED.,.F.,.F.,(4,1,1,1,1,1,1,1,1,1,1,1,1,1,4),(172.787595947439,
172.812748594066,173.311483225598,173.81021785713,174.308952488663,174.807687120195,
175.306421751727,175.805156383259,176.303891014791,176.802625646324,177.301360277856,
177.800094909388,178.29882954092,178.797564172452,179.070781254618),
 .UNSPECIFIED.);
#9486=B_SPLINE_CURVE_WITH_KNOTS('',3,(#59826,#59827,#59828,#59829,#59830,
#59831,#59832,#59833,#59834,#59835,#59836,#59837,#59838,#59839,#59840,#59841,
#59842),.UNSPECIFIED.,.F.,.F.,(4,1,1,1,1,1,1,1,1,1,1,1,1,1,4),(172.787595947439,
173.025692175744,173.523341546737,174.020990917731,174.518640288724,175.016289659717,
175.51393903071,176.011588401704,176.509237772697,177.00688714369,177.504536514684,
178.002185885677,178.49983525667,178.997484627663,179.070781254618),
 .UNSPECIFIED.);
#9487=B_SPLINE_CURVE_WITH_KNOTS('',3,(#59847,#59848,#59849,#59850,#59851,
#59852,#59853,#59854,#59855,#59856,#59857,#59858,#59859,#59860,#59861,#59862),
 .UNSPECIFIED.,.F.,.F.,(4,1,1,1,1,1,1,1,1,1,1,1,1,4),(166.504410640259,
166.82793301568,167.326667647212,167.825402278744,168.324136910276,168.822871541809,
169.321606173341,169.820340804873,170.319075436405,170.817810067937,171.31654469947,
171.815279331002,172.314013962534,172.787595947439),.UNSPECIFIED.);
#9488=B_SPLINE_CURVE_WITH_KNOTS('',3,(#59863,#59864,#59865,#59866,#59867,
#59868,#59869,#59870,#59871,#59872,#59873,#59874,#59875,#59876,#59877,#59878,
#59879),.UNSPECIFIED.,.F.,.F.,(4,1,1,1,1,1,1,1,1,1,1,1,1,1,4),(166.504410640259,
166.556250352832,167.053899723825,167.551549094818,168.049198465811,168.546847836805,
169.044497207798,169.542146578791,170.039795949784,170.537445320778,171.035094691771,
171.532744062764,172.030393433758,172.528042804751,172.787595947439),
 .UNSPECIFIED.);
#9489=B_SPLINE_CURVE_WITH_KNOTS('',3,(#59884,#59885,#59886,#59887,#59888,
#59889,#59890,#59891,#59892,#59893,#59894,#59895,#59896,#59897,#59898,#59899,
#59900),.UNSPECIFIED.,.F.,.F.,(4,1,1,1,1,1,1,1,1,1,1,1,1,1,4),(160.22122533308,
160.344382805762,160.843117437294,161.341852068826,161.840586700358,162.33932133189,
162.838055963423,163.336790594955,163.835525226487,164.334259858019,164.832994489551,
165.331729121083,165.830463752616,166.329198384148,166.504410640259),
 .UNSPECIFIED.);
#9490=B_SPLINE_CURVE_WITH_KNOTS('',3,(#59901,#59902,#59903,#59904,#59905,
#59906,#59907,#59908,#59909,#59910,#59911,#59912,#59913,#59914,#59915,#59916),
 .UNSPECIFIED.,.F.,.F.,(4,1,1,1,1,1,1,1,1,1,1,1,1,4),(160.22122533308,160.584457900912,
161.082107271906,161.579756642899,162.077406013892,162.575055384885,163.072704755879,
163.570354126872,164.068003497865,164.565652868858,165.063302239852,165.560951610845,
166.058600981838,166.504410640259),.UNSPECIFIED.);
#9491=B_SPLINE_CURVE_WITH_KNOTS('',3,(#59921,#59922,#59923,#59924,#59925,
#59926,#59927,#59928,#59929,#59930,#59931,#59932,#59933,#59934,#59935,#59936),
 .UNSPECIFIED.,.F.,.F.,(4,1,1,1,1,1,1,1,1,1,1,1,1,4),(153.9380400259,154.359567227376,
154.858301858908,155.35703649044,155.855771121972,156.354505753504,156.853240385036,
157.351975016569,157.850709648101,158.349444279633,158.848178911165,159.346913542697,
159.845648174229,160.22122533308),.UNSPECIFIED.);
#9492=B_SPLINE_CURVE_WITH_KNOTS('',3,(#59937,#59938,#59939,#59940,#59941,
#59942,#59943,#59944,#59945,#59946,#59947,#59948,#59949,#59950,#59951,#59952,
#59953),.UNSPECIFIED.,.F.,.F.,(4,1,1,1,1,1,1,1,1,1,1,1,1,1,4),(153.9380400259,
154.115016078,154.612665448993,155.110314819986,155.60796419098,156.105613561973,
156.603262932966,157.100912303959,157.598561674953,158.096211045946,158.593860416939,
159.091509787932,159.589159158926,160.086808529919,160.22122533308),
 .UNSPECIFIED.);
#9493=B_SPLINE_CURVE_WITH_KNOTS('',3,(#59958,#59959,#59960,#59961,#59962,
#59963,#59964,#59965,#59966,#59967,#59968,#59969,#59970,#59971,#59972,#59973,
#59974),.UNSPECIFIED.,.F.,.F.,(4,1,1,1,1,1,1,1,1,1,1,1,1,1,4),(147.65485471872,
147.876017017457,148.374751648989,148.873486280522,149.372220912054,149.870955543586,
150.369690175118,150.86842480665,151.367159438182,151.865894069715,152.364628701247,
152.863363332779,153.362097964311,153.860832595843,153.9380400259),
 .UNSPECIFIED.);
#9494=B_SPLINE_CURVE_WITH_KNOTS('',3,(#59975,#59976,#59977,#59978,#59979,
#59980,#59981,#59982,#59983,#59984,#59985,#59986,#59987,#59988,#59989,#59990),
 .UNSPECIFIED.,.F.,.F.,(4,1,1,1,1,1,1,1,1,1,1,1,1,4),(147.65485471872,148.14322362608,
148.640872997074,149.138522368067,149.63617173906,150.133821110054,150.631470481047,
151.12911985204,151.626769223033,152.124418594027,152.62206796502,153.119717336013,
153.617366707006,153.9380400259),.UNSPECIFIED.);
#9495=B_SPLINE_CURVE_WITH_KNOTS('',3,(#59995,#59996,#59997,#59998,#59999,
#60000,#60001,#60002,#60003,#60004,#60005,#60006,#60007,#60008,#60009,#60010,
#60011),.UNSPECIFIED.,.F.,.F.,(4,1,1,1,1,1,1,1,1,1,1,1,1,1,4),(141.371669411541,
141.392466807539,141.891201439071,142.389936070603,142.888670702135,143.387405333668,
143.8861399652,144.384874596732,144.883609228264,145.382343859796,145.881078491329,
146.379813122861,146.878547754393,147.377282385925,147.65485471872),
 .UNSPECIFIED.);
#9496=B_SPLINE_CURVE_WITH_KNOTS('',3,(#60012,#60013,#60014,#60015,#60016,
#60017,#60018,#60019,#60020,#60021,#60022,#60023,#60024,#60025,#60026,#60027,
#60028),.UNSPECIFIED.,.F.,.F.,(4,1,1,1,1,1,1,1,1,1,1,1,1,1,4),(141.371669411541,
141.673781803168,142.171431174161,142.669080545154,143.166729916148,143.664379287141,
144.162028658134,144.659678029128,145.157327400121,145.654976771114,146.152626142107,
146.650275513101,147.147924884094,147.645574255087,147.65485471872),
 .UNSPECIFIED.);
#9497=B_SPLINE_CURVE_WITH_KNOTS('',3,(#60033,#60034,#60035,#60036,#60037,
#60038,#60039,#60040,#60041,#60042,#60043,#60044,#60045,#60046,#60047,#60048),
 .UNSPECIFIED.,.F.,.F.,(4,1,1,1,1,1,1,1,1,1,1,1,1,4),(135.088484104361,
135.407651229153,135.906385860685,136.405120492217,136.903855123749,137.402589755281,
137.901324386814,138.400059018346,138.898793649878,139.39752828141,139.896262912942,
140.394997544475,140.893732176007,141.371669411541),.UNSPECIFIED.);
#9498=B_SPLINE_CURVE_WITH_KNOTS('',3,(#60049,#60050,#60051,#60052,#60053,
#60054,#60055,#60056,#60057,#60058,#60059,#60060,#60061,#60062,#60063,#60064,
#60065),.UNSPECIFIED.,.F.,.F.,(4,1,1,1,1,1,1,1,1,1,1,1,1,1,4),(135.088484104361,
135.204339980255,135.701989351249,136.199638722242,136.697288093235,137.194937464228,
137.692586835222,138.190236206215,138.687885577208,139.185534948202,139.683184319195,
140.180833690188,140.678483061181,141.176132432175,141.371669411541),
 .UNSPECIFIED.);
#9499=B_SPLINE_CURVE_WITH_KNOTS('',3,(#60070,#60071,#60072,#60073,#60074,
#60075,#60076,#60077,#60078,#60079,#60080,#60081,#60082,#60083,#60084,#60085,
#60086),.UNSPECIFIED.,.F.,.F.,(4,1,1,1,1,1,1,1,1,1,1,1,1,1,4),(128.805298797182,
128.924101019234,129.422835650767,129.921570282299,130.420304913831,130.919039545363,
131.417774176895,131.916508808428,132.41524343996,132.913978071492,133.412712703024,
133.911447334556,134.410181966088,134.908916597621,135.088484104361),
 .UNSPECIFIED.);
#9500=B_SPLINE_CURVE_WITH_KNOTS('',3,(#60087,#60088,#60089,#60090,#60091,
#60092,#60093,#60094,#60095,#60096,#60097,#60098,#60099,#60100,#60101,#60102),
 .UNSPECIFIED.,.F.,.F.,(4,1,1,1,1,1,1,1,1,1,1,1,1,4),(128.805298797182,
129.232547528336,129.730196899329,130.227846270323,130.725495641316,131.223145012309,
131.720794383302,132.218443754296,132.716093125289,133.213742496282,133.711391867276,
134.209041238269,134.706690609262,135.088484104361),.UNSPECIFIED.);
#9501=B_SPLINE_CURVE_WITH_KNOTS('',3,(#60107,#60108,#60109,#60110,#60111,
#60112,#60113,#60114,#60115,#60116,#60117,#60118,#60119,#60120,#60121,#60122),
 .UNSPECIFIED.,.F.,.F.,(4,1,1,1,1,1,1,1,1,1,1,1,1,4),(122.522113490002,
122.939285440848,123.43802007238,123.936754703913,124.435489335445,124.934223966977,
125.432958598509,125.931693230041,126.430427861574,126.929162493106,127.427897124638,
127.92663175617,128.425366387702,128.805298797182),.UNSPECIFIED.);
#9502=B_SPLINE_CURVE_WITH_KNOTS('',3,(#60123,#60124,#60125,#60126,#60127,
#60128,#60129,#60130,#60131,#60132,#60133,#60134,#60135,#60136,#60137,#60138,
#60139),.UNSPECIFIED.,.F.,.F.,(4,1,1,1,1,1,1,1,1,1,1,1,1,1,4),(122.522113490002,
122.763105705424,123.260755076417,123.75840444741,124.256053818403,124.753703189397,
125.25135256039,125.749001931383,126.246651302376,126.74430067337,127.241950044363,
127.739599415356,128.23724878635,128.734898157343,128.805298797182),
 .UNSPECIFIED.);
#9503=B_SPLINE_CURVE_WITH_KNOTS('',3,(#60144,#60145,#60146,#60147,#60148,
#60149,#60150,#60151,#60152,#60153,#60154,#60155,#60156,#60157,#60158,#60159,
#60160),.UNSPECIFIED.,.F.,.F.,(4,1,1,1,1,1,1,1,1,1,1,1,1,1,4),(116.238928182823,
116.45573523093,116.954469862462,117.453204493994,117.951939125527,118.450673757059,
118.949408388591,119.448143020123,119.946877651655,120.445612283187,120.94434691472,
121.443081546252,121.941816177784,122.440550809316,122.522113490002),
 .UNSPECIFIED.);
#9504=B_SPLINE_CURVE_WITH_KNOTS('',3,(#60161,#60162,#60163,#60164,#60165,
#60166,#60167,#60168,#60169,#60170,#60171,#60172,#60173,#60174,#60175,#60176,
#60177),.UNSPECIFIED.,.F.,.F.,(4,1,1,1,1,1,1,1,1,1,1,1,1,1,4),(116.238928182823,
116.293663882511,116.791313253504,117.288962624498,117.786611995491,118.284261366484,
118.781910737477,119.279560108471,119.777209479464,120.274858850457,120.77250822145,
121.270157592444,121.767806963437,122.26545633443,122.522113490002),
 .UNSPECIFIED.);
#9505=B_SPLINE_CURVE_WITH_KNOTS('',3,(#60182,#60183,#60184,#60185,#60186,
#60187,#60188,#60189,#60190,#60191,#60192,#60193,#60194,#60195,#60196,#60197,
#60198),.UNSPECIFIED.,.F.,.F.,(4,1,1,1,1,1,1,1,1,1,1,1,1,1,4),(109.955742875643,
109.972185021012,110.470919652544,110.969654284076,111.468388915608,111.96712354714,
112.465858178673,112.964592810205,113.463327441737,113.962062073269,114.460796704801,
114.959531336333,115.458265967866,115.957000599398,116.238928182823),
 .UNSPECIFIED.);
#9506=B_SPLINE_CURVE_WITH_KNOTS('',3,(#60199,#60200,#60201,#60202,#60203,
#60204,#60205,#60206,#60207,#60208,#60209,#60210,#60211,#60212,#60213,#60214),
 .UNSPECIFIED.,.F.,.F.,(4,1,1,1,1,1,1,1,1,1,1,1,1,4),(109.955742875643,
110.321871430592,110.819520801585,111.317170172578,111.814819543572,112.312468914565,
112.810118285558,113.307767656551,113.805417027545,114.303066398538,114.800715769531,
115.298365140524,115.796014511518,116.238928182823),.UNSPECIFIED.);
#9507=B_SPLINE_CURVE_WITH_KNOTS('',3,(#60219,#60220,#60221,#60222,#60223,
#60224,#60225,#60226,#60227,#60228,#60229,#60230,#60231,#60232,#60233,#60234),
 .UNSPECIFIED.,.F.,.F.,(4,1,1,1,1,1,1,1,1,1,1,1,1,4),(103.672557568463,
103.987369442626,104.486104074158,104.98483870569,105.483573337222,105.982307968754,
106.481042600286,106.979777231819,107.478511863351,107.977246494883,108.475981126415,
108.974715757947,109.47345038948,109.955742875643),.UNSPECIFIED.);
#9508=B_SPLINE_CURVE_WITH_KNOTS('',3,(#60235,#60236,#60237,#60238,#60239,
#60240,#60241,#60242,#60243,#60244,#60245,#60246,#60247,#60248,#60249,#60250,
#60251),.UNSPECIFIED.,.F.,.F.,(4,1,1,1,1,1,1,1,1,1,1,1,1,1,4),(103.672557568463,
103.852429607679,104.350078978673,104.847728349666,105.345377720659,105.843027091652,
106.340676462646,106.838325833639,107.335975204632,107.833624575625,108.331273946619,
108.828923317612,109.326572688605,109.824222059598,109.955742875643),
 .UNSPECIFIED.);
#9509=B_SPLINE_CURVE_WITH_KNOTS('',3,(#60256,#60257,#60258,#60259,#60260,
#60261,#60262,#60263,#60264,#60265,#60266,#60267,#60268,#60269,#60270,#60271,
#60272),.UNSPECIFIED.,.F.,.F.,(4,1,1,1,1,1,1,1,1,1,1,1,1,1,4),(97.3893722612837,
97.5038192327072,98.0025538642394,98.5012884957716,99.0000231273038,99.4987577588359,
99.9974923903681,100.4962270219,100.994961653432,101.493696284965,101.992430916497,
102.491165548029,102.989900179561,103.488634811093,103.672557568463),
 .UNSPECIFIED.);
#9510=B_SPLINE_CURVE_WITH_KNOTS('',3,(#60273,#60274,#60275,#60276,#60277,
#60278,#60279,#60280,#60281,#60282,#60283,#60284,#60285,#60286,#60287,#60288),
 .UNSPECIFIED.,.F.,.F.,(4,1,1,1,1,1,1,1,1,1,1,1,1,4),(97.3893722612837,
97.88063715576,98.3782865267532,98.8759358977465,99.3735852687398,99.8712346397331,
100.368884010726,100.86653338172,101.364182752713,101.861832123706,102.359481494699,
102.857130865693,103.354780236686,103.672557568463),.UNSPECIFIED.);
#9511=B_SPLINE_CURVE_WITH_KNOTS('',3,(#60293,#60294,#60295,#60296,#60297,
#60298,#60299,#60300,#60301,#60302,#60303,#60304,#60305,#60306,#60307,#60308),
 .UNSPECIFIED.,.F.,.F.,(4,1,1,1,1,1,1,1,1,1,1,1,1,4),(91.1061869541041,
91.5190036543211,92.0177382858533,92.5164729173855,93.0152075489176,93.5139421804498,
94.012676811982,94.5114114435142,95.0101460750464,95.5088807065785,96.0076153381107,
96.5063499696429,97.0050846011751,97.3893722612837),.UNSPECIFIED.);
#9512=B_SPLINE_CURVE_WITH_KNOTS('',3,(#60309,#60310,#60311,#60312,#60313,
#60314,#60315,#60316,#60317,#60318,#60319,#60320,#60321,#60322,#60323,#60324,
#60325),.UNSPECIFIED.,.F.,.F.,(4,1,1,1,1,1,1,1,1,1,1,1,1,1,4),(91.1061869541041,
91.4111953328474,91.9088447038407,92.406494074834,92.9041434458272,93.4017928168205,
93.8994421878138,94.3970915588071,94.8947409298003,95.3923903007936,95.8900396717869,
96.3876890427802,96.8853384137734,97.3829877847667,97.3893722612837),
 .UNSPECIFIED.);
#9513=B_SPLINE_CURVE_WITH_KNOTS('',3,(#60330,#60331,#60332,#60333,#60334,
#60335,#60336,#60337,#60338,#60339,#60340,#60341,#60342,#60343,#60344,#60345,
#60346),.UNSPECIFIED.,.F.,.F.,(4,1,1,1,1,1,1,1,1,1,1,1,1,1,4),(84.8230016469246,
85.0354534444028,85.534188075935,86.0329227074672,86.5316573389993,87.0303919705315,
87.5291266020637,88.0278612335959,88.526595865128,89.0253304966602,89.5240651281924,
90.0227997597246,90.5215343912568,91.0202690227889,91.1061869541041),
 .UNSPECIFIED.);
#9514=B_SPLINE_CURVE_WITH_KNOTS('',3,(#60347,#60348,#60349,#60350,#60351,
#60352,#60353,#60354,#60355,#60356,#60357,#60358,#60359,#60360,#60361,#60362,
#60363),.UNSPECIFIED.,.F.,.F.,(4,1,1,1,1,1,1,1,1,1,1,1,1,1,4),(84.8230016469246,
84.9417535099349,85.4394028809282,85.9370522519214,86.4347016229147,86.932350993908,
87.4300003649012,87.9276497358945,88.4252991068878,88.9229484778811,89.4205978488743,
89.9182472198676,90.4158965908609,90.9135459618542,91.1061869541041),
 .UNSPECIFIED.);
#9515=B_SPLINE_CURVE_WITH_KNOTS('',3,(#60368,#60369,#60370,#60371,#60372,
#60373,#60374,#60375,#60376,#60377,#60378,#60379,#60380,#60381,#60382,#60383,
#60384),.UNSPECIFIED.,.F.,.F.,(4,1,1,1,1,1,1,1,1,1,1,1,1,1,4),(78.539816339745,
78.5519032344845,79.0506378660167,79.5493724975488,80.048107129081,80.5468417606132,
81.0455763921454,81.5443110236776,82.0430456552097,82.5417802867419,83.0405149182741,
83.5392495498063,84.0379841813384,84.5367188128706,84.8230016469246),
 .UNSPECIFIED.);
#9516=B_SPLINE_CURVE_WITH_KNOTS('',3,(#60385,#60386,#60387,#60388,#60389,
#60390,#60391,#60392,#60393,#60394,#60395,#60396,#60397,#60398,#60399,#60400),
 .UNSPECIFIED.,.F.,.F.,(4,1,1,1,1,1,1,1,1,1,1,1,1,4),(78.539816339745,78.9699610580156,
79.4676104290089,79.9652598000022,80.4629091709954,80.9605585419887,81.458207912982,
81.9558572839753,82.4535066549685,82.9511560259618,83.4488053969551,83.9464547679483,
84.4441041389416,84.8230016469246),.UNSPECIFIED.);
#9517=B_SPLINE_CURVE_WITH_KNOTS('',3,(#60405,#60406,#60407,#60408,#60409,
#60410,#60411,#60412,#60413,#60414,#60415,#60416,#60417,#60418,#60419,#60420),
 .UNSPECIFIED.,.F.,.F.,(4,1,1,1,1,1,1,1,1,1,1,1,1,4),(72.2566310325654,
72.5670876560984,73.0658222876305,73.5645569191627,74.0632915506949,74.5620261822271,
75.0607608137592,75.5594954452914,76.0582300768236,76.5569647083558,77.055699339888,
77.5544339714201,78.0531686029523,78.539816339745),.UNSPECIFIED.);
#9518=B_SPLINE_CURVE_WITH_KNOTS('',3,(#60421,#60422,#60423,#60424,#60425,
#60426,#60427,#60428,#60429,#60430,#60431,#60432,#60433,#60434,#60435,#60436,
#60437),.UNSPECIFIED.,.F.,.F.,(4,1,1,1,1,1,1,1,1,1,1,1,1,1,4),(72.2566310325654,
72.5005192351031,72.9981686060964,73.4958179770896,73.9934673480829,74.4911167190762,
74.9887660900694,75.4864154610627,75.984064832056,76.4817142030493,76.9793635740425,
77.4770129450358,77.9746623160291,78.4723116870224,78.539816339745),
 .UNSPECIFIED.);
#9519=B_SPLINE_CURVE_WITH_KNOTS('',3,(#60442,#60443,#60444,#60445,#60446,
#60447,#60448,#60449,#60450,#60451,#60452,#60453,#60454,#60455,#60456,#60457,
#60458),.UNSPECIFIED.,.F.,.F.,(4,1,1,1,1,1,1,1,1,1,1,1,1,1,4),(65.9734457253857,
66.08353744618,66.5822720777122,67.0810067092444,67.5797413407766,68.0784759723088,
68.5772106038409,69.0759452353731,69.5746798669053,70.0734144984375,70.5721491299696,
71.0708837615018,71.569618393034,72.0683530245662,72.2566310325654),
 .UNSPECIFIED.);
#9520=B_SPLINE_CURVE_WITH_KNOTS('',3,(#60459,#60460,#60461,#60462,#60463,
#60464,#60465,#60466,#60467,#60468,#60469,#60470,#60471,#60472,#60473,#60474,
#60475),.UNSPECIFIED.,.F.,.F.,(4,1,1,1,1,1,1,1,1,1,1,1,1,1,4),(65.9734457253857,
66.0310774121906,66.5287267831838,67.0263761541771,67.5240255251704,68.0216748961636,
68.5193242671569,69.0169736381502,69.5146230091434,70.0122723801367,70.50992175113,
71.0075711221233,71.5052204931165,72.0028698641098,72.2566310325654),
 .UNSPECIFIED.);
#9521=B_SPLINE_CURVE_WITH_KNOTS('',3,(#60480,#60481,#60482,#60483,#60484,
#60485,#60486,#60487,#60488,#60489,#60490,#60491,#60492,#60493,#60494,#60495),
 .UNSPECIFIED.,.F.,.F.,(4,1,1,1,1,1,1,1,1,1,1,1,1,4),(59.6902604182062,
60.0987218677939,60.5974564993261,61.0961911308583,61.5949257623904,62.0936603939226,
62.5923950254548,63.091129656987,63.5898642885191,64.0885989200513,64.5873335515835,
65.0860681831157,65.5848028146479,65.9734457253857),.UNSPECIFIED.);
#9522=B_SPLINE_CURVE_WITH_KNOTS('',3,(#60496,#60497,#60498,#60499,#60500,
#60501,#60502,#60503,#60504,#60505,#60506,#60507,#60508,#60509,#60510,#60511),
 .UNSPECIFIED.,.F.,.F.,(4,1,1,1,1,1,1,1,1,1,1,1,1,4),(59.6902604182062,
60.0592849602713,60.5569343312646,61.0545837022578,61.5522330732511,62.0498824442444,
62.5475318152376,63.0451811862309,63.5428305572242,64.0404799282175,64.5381292992107,
65.035778670204,65.5334280411973,65.9734457253857),.UNSPECIFIED.);
#9523=B_SPLINE_CURVE_WITH_KNOTS('',3,(#60516,#60517,#60518,#60519,#60520,
#60521,#60522,#60523,#60524,#60525,#60526,#60527,#60528,#60529,#60530,#60531,
#60532),.UNSPECIFIED.,.F.,.F.,(4,1,1,1,1,1,1,1,1,1,1,1,1,1,4),(53.4070751110266,
53.6151716578756,54.1139062894078,54.6126409209399,55.1113755524721,55.6101101840043,
56.1088448155365,56.6075794470687,57.1063140786008,57.605048710133,58.1037833416652,
58.6025179731974,59.1012526047295,59.5999872362617,59.6902604182062),
 .UNSPECIFIED.);
#9524=B_SPLINE_CURVE_WITH_KNOTS('',3,(#60533,#60534,#60535,#60536,#60537,
#60538,#60539,#60540,#60541,#60542,#60543,#60544,#60545,#60546,#60547,#60548,
#60549),.UNSPECIFIED.,.F.,.F.,(4,1,1,1,1,1,1,1,1,1,1,1,1,1,4),(53.4070751110266,
53.5898431373587,54.087492508352,54.5851418793453,55.0827912503386,55.5804406213318,
56.0780899923251,56.5757393633184,57.0733887343116,57.5710381053049,58.0686874762982,
58.5663368472915,59.0639862182847,59.561635589278,59.6902604182062),
 .UNSPECIFIED.);
#9525=B_SPLINE_CURVE_WITH_KNOTS('',3,(#60554,#60555,#60556,#60557,#60558,
#60559,#60560,#60561,#60562,#60563,#60564,#60565,#60566,#60567,#60568,#60569,
#60570),.UNSPECIFIED.,.F.,.F.,(4,1,1,1,1,1,1,1,1,1,1,1,1,1,4),(47.123889803847,
47.1316214479573,47.6303560794895,48.1290907110216,48.6278253425538,49.126559974086,
49.6252946056182,50.1240292371503,50.6227638686825,51.1214985002147,51.6202331317469,
52.1189677632791,52.6177023948112,53.1164370263434,53.4070751110266),
 .UNSPECIFIED.);
#9526=B_SPLINE_CURVE_WITH_KNOTS('',3,(#60571,#60572,#60573,#60574,#60575,
#60576,#60577,#60578,#60579,#60580,#60581,#60582,#60583,#60584,#60585,#60586),
 .UNSPECIFIED.,.F.,.F.,(4,1,1,1,1,1,1,1,1,1,1,1,1,4),(47.123889803847,47.6180506854395,
48.1157000564327,48.613349427426,49.1109987984193,49.6086481694126,50.1062975404058,
50.6039469113991,51.1015962823924,51.5992456533857,52.0968950243789,52.5945443953722,
53.0921937663655,53.4070751110266),.UNSPECIFIED.);
#9527=B_SPLINE_CURVE_WITH_KNOTS('',3,(#60591,#60592,#60593,#60594,#60595,
#60596,#60597,#60598,#60599,#60600,#60601,#60602,#60603,#60604,#60605,#60606),
 .UNSPECIFIED.,.F.,.F.,(4,1,1,1,1,1,1,1,1,1,1,1,1,4),(40.8407044966674,
41.1468058695711,41.6455405011033,42.1442751326355,42.6430097641677,43.1417443956999,
43.640479027232,44.1392136587642,44.6379482902964,45.1366829218286,45.6354175533607,
46.1341521848929,46.6328868164251,47.123889803847),.UNSPECIFIED.);
#9528=B_SPLINE_CURVE_WITH_KNOTS('',3,(#60607,#60608,#60609,#60610,#60611,
#60612,#60613,#60614,#60615,#60616,#60617,#60618,#60619,#60620,#60621,#60622,
#60623),.UNSPECIFIED.,.F.,.F.,(4,1,1,1,1,1,1,1,1,1,1,1,1,1,4),(40.8407044966674,
41.1486088625269,41.6462582335202,42.1439076045135,42.6415569755068,43.1392063465,
43.6368557174933,44.1345050884866,44.6321544594798,45.1298038304731,45.6274532014664,
46.1251025724597,46.6227519434529,47.1204013144462,47.123889803847),
 .UNSPECIFIED.);
#9529=B_SPLINE_CURVE_WITH_KNOTS('',3,(#60628,#60629,#60630,#60631,#60632,
#60633,#60634,#60635,#60636,#60637,#60638,#60639,#60640,#60641,#60642,#60643,
#60644),.UNSPECIFIED.,.F.,.F.,(4,1,1,1,1,1,1,1,1,1,1,1,1,1,4),(34.5575191894878,
34.6632556596528,35.161990291185,35.6607249227172,36.1594595542494,36.6581941857815,
37.1569288173137,37.6556634488459,38.1543980803781,38.6531327119103,39.1518673434424,
39.6506019749746,40.1493366065068,40.648071238039,40.8407044966674),
 .UNSPECIFIED.);
#9530=B_SPLINE_CURVE_WITH_KNOTS('',3,(#60645,#60646,#60647,#60648,#60649,
#60650,#60651,#60652,#60653,#60654,#60655,#60656,#60657,#60658,#60659,#60660,
#60661),.UNSPECIFIED.,.F.,.F.,(4,1,1,1,1,1,1,1,1,1,1,1,1,1,4),(34.5575191894878,
34.6791670396144,35.1768164106077,35.6744657816009,36.1721151525942,36.6697645235875,
37.1674138945808,37.665063265574,38.1627126365673,38.6603620075606,39.1580113785539,
39.6556607495471,40.1533101205404,40.6509594915337,40.8407044966674),
 .UNSPECIFIED.);
#9531=B_SPLINE_CURVE_WITH_KNOTS('',3,(#60666,#60667,#60668,#60669,#60670,
#60671,#60672,#60673,#60674,#60675,#60676,#60677,#60678,#60679,#60680,#60681),
 .UNSPECIFIED.,.F.,.F.,(4,1,1,1,1,1,1,1,1,1,1,1,1,4),(28.2743338823082,
28.6784400812667,29.1771747127989,29.6759093443311,30.1746439758632,30.6733786073954,
31.1721132389276,31.6708478704598,32.1695825019919,32.6683171335241,33.1670517650563,
33.6657863965885,34.1645210281207,34.5575191894878),.UNSPECIFIED.);
#9532=B_SPLINE_CURVE_WITH_KNOTS('',3,(#60682,#60683,#60684,#60685,#60686,
#60687,#60688,#60689,#60690,#60691,#60692,#60693,#60694,#60695,#60696,#60697),
 .UNSPECIFIED.,.F.,.F.,(4,1,1,1,1,1,1,1,1,1,1,1,1,4),(28.2743338823082,
28.7073745876951,29.2050239586884,29.7026733296817,30.2003227006749,30.6979720716682,
31.1956214426615,31.6932708136548,32.190920184648,32.6885695556413,33.1862189266346,
33.6838682976279,34.1815176686211,34.5575191894878),.UNSPECIFIED.);
#9533=B_SPLINE_CURVE_WITH_KNOTS('',3,(#60702,#60703,#60704,#60705,#60706,
#60707,#60708,#60709,#60710,#60711,#60712,#60713,#60714,#60715,#60716,#60717,
#60718),.UNSPECIFIED.,.F.,.F.,(4,1,1,1,1,1,1,1,1,1,1,1,1,1,4),(21.9911485751286,
22.1948898713484,22.6936245028806,23.1923591344127,23.6910937659449,24.1898283974771,
24.6885630290093,25.1872976605415,25.6860322920736,26.1847669236058,26.683501555138,
27.1822361866702,27.6809708182023,28.1797054497345,28.2743338823082),
 .UNSPECIFIED.);
#9534=B_SPLINE_CURVE_WITH_KNOTS('',3,(#60719,#60720,#60721,#60722,#60723,
#60724,#60725,#60726,#60727,#60728,#60729,#60730,#60731,#60732,#60733,#60734,
#60735),.UNSPECIFIED.,.F.,.F.,(4,1,1,1,1,1,1,1,1,1,1,1,1,1,4),(21.9911485751286,
22.2379327647826,22.7355821357759,23.2332315067691,23.7308808777624,24.2285302487557,
24.726179619749,25.2238289907422,25.7214783617355,26.2191277327288,26.716777103722,
27.2144264747153,27.7120758457086,28.2097252167019,28.2743338823082),
 .UNSPECIFIED.);
#9535=B_SPLINE_CURVE_WITH_KNOTS('',3,(#60740,#60741,#60742,#60743,#60744,
#60745,#60746,#60747,#60748,#60749,#60750,#60751,#60752,#60753,#60754,#60755,
#60756),.UNSPECIFIED.,.F.,.F.,(4,1,1,1,1,1,1,1,1,1,1,1,1,1,4),(15.707963267949,
15.7113396614301,16.2100742929623,16.7088089244944,17.2075435560266,17.7062781875588,
18.205012819091,18.7037474506231,19.2024820821553,19.7012167136875,20.1999513452197,
20.6986859767519,21.197420608284,21.6961552398162,21.9911485751286),
 .UNSPECIFIED.);
#9536=B_SPLINE_CURVE_WITH_KNOTS('',3,(#60757,#60758,#60759,#60760,#60761,
#60762,#60763,#60764,#60765,#60766,#60767,#60768,#60769,#60770,#60771,#60772,
#60773),.UNSPECIFIED.,.F.,.F.,(4,1,1,1,1,1,1,1,1,1,1,1,1,1,4),(15.707963267949,
15.7684909418701,16.2661403128633,16.7637896838566,17.2614390548499,17.7590884258431,
18.2567377968364,18.7543871678297,19.252036538823,19.7496859098162,20.2473352808095,
20.7449846518028,21.242634022796,21.7402833937893,21.9911485751286),
 .UNSPECIFIED.);
#9537=B_SPLINE_CURVE_WITH_KNOTS('',3,(#60865,#60866,#60867,#60868,#60869,
#60870,#60871,#60872,#60873,#60874,#60875,#60876,#60877,#60878,#60879,#60880,
#60881,#60882,#60883,#60884,#60885,#60886),.UNSPECIFIED.,.T.,.F.,(4,1,1,
1,1,1,1,1,1,1,1,1,1,1,1,1,1,1,1,4),(1.5707963267949,2.01959527730772,2.46839422782055,
2.76759352816244,3.06679282850432,3.36599212884621,3.66519142918809,3.96439072952998,
4.26359002987186,4.56278933021375,4.86198863055563,5.16118793089752,5.4603872312394,
5.75958653158129,6.05878583192317,6.20838548209412,6.35798513226506,6.95638373294883,
7.40518268346166,7.85398163397448),.UNSPECIFIED.);
#9538=B_SPLINE_CURVE_WITH_KNOTS('',3,(#60887,#60888,#60889,#60890,#60891,
#60892,#60893,#60894,#60895,#60896,#60897,#60898,#60899,#60900,#60901,#60902,
#60903,#60904,#60905,#60906,#60907,#60908),.UNSPECIFIED.,.T.,.F.,(4,1,1,
1,1,1,1,1,1,1,1,1,1,1,1,1,1,1,1,4),(-7.85398163397448,-7.40518268346166,
-6.95638373294883,-6.35798513226506,-6.20838548209412,-6.05878583192317,
-5.75958653158129,-5.4603872312394,-5.16118793089752,-4.86198863055563,
-4.56278933021375,-4.26359002987186,-3.96439072952998,-3.66519142918809,
-3.36599212884621,-3.06679282850432,-2.76759352816244,-2.46839422782055,
-2.01959527730772,-1.5707963267949),.UNSPECIFIED.);
#9539=B_SPLINE_CURVE_WITH_KNOTS('',3,(#61060,#61061,#61062,#61063,#61064,
#61065,#61066,#61067,#61068,#61069,#61070,#61071,#61072,#61073,#61074,#61075,
#61076,#61077,#61078,#61079,#61080,#61081,#61082,#61083,#61084,#61085,#61086,
#61087,#61088,#61089,#61090,#61091,#61092,#61093,#61094,#61095,#61096,#61097,
#61098,#61099,#61100,#61101,#61102,#61103,#61104,#61105,#61106,#61107,#61108,
#61109,#61110,#61111,#61112,#61113,#61114,#61115,#61116,#61117,#61118,#61119,
#61120),.UNSPECIFIED.,.T.,.F.,(4,3,3,3,3,3,3,3,3,3,3,3,3,3,3,3,3,3,3,3,
4),(-7.85398163397448,-7.40518268346166,-6.95638373294883,-6.65718443260694,
-6.35798513226506,-6.20838548209412,-6.05878583192317,-5.75958653158129,
-5.4603872312394,-5.16118793089752,-4.86198863055563,-4.56278933021375,
-4.26359002987186,-3.96439072952998,-3.66519142918809,-3.36599212884621,
-3.06679282850432,-2.76759352816244,-2.46839422782055,-2.01959527730772,
-1.5707963267949),.UNSPECIFIED.);
#9540=B_SPLINE_CURVE_WITH_KNOTS('',3,(#61219,#61220,#61221,#61222,#61223,
#61224,#61225,#61226,#61227,#61228,#61229,#61230,#61231),.UNSPECIFIED.,
 .F.,.F.,(4,1,1,1,1,1,1,1,1,1,4),(1.5707963267949,2.01959527730772,2.46839422782055,
2.76759352816244,3.06679282850432,3.36599212884621,3.66519142918809,3.96439072952998,
4.26359002987186,4.56278933021375,4.71238073889391),.UNSPECIFIED.);
#9541=B_SPLINE_CURVE_WITH_KNOTS('',3,(#61232,#61233,#61234,#61235,#61236,
#61237,#61238,#61239,#61240,#61241,#61242,#61243,#61244,#61245),
 .UNSPECIFIED.,.F.,.F.,(4,1,1,1,1,1,1,1,1,1,1,4),(4.71238073889391,4.86198863055563,
5.16118793089752,5.4603872312394,5.75958653158129,6.05878583192317,6.20838548209412,
6.35798513226506,6.65718443260694,6.95638373294883,7.40518268346166,7.85398163397448),
 .UNSPECIFIED.);
#9542=B_SPLINE_CURVE_WITH_KNOTS('',3,(#61250,#61251,#61252,#61253,#61254,
#61255,#61256,#61257,#61258,#61259,#61260,#61261,#61262,#61263),
 .UNSPECIFIED.,.F.,.F.,(4,1,1,1,1,1,1,1,1,1,1,4),(-7.85398163397448,-7.40518268346166,
-6.95638373294883,-6.65718443260694,-6.35798513226506,-6.20838548209412,
-6.05878583192317,-5.75958653158129,-5.4603872312394,-5.16118793089752,
-4.86198863055563,-4.71239722187547),.UNSPECIFIED.);
#9543=B_SPLINE_CURVE_WITH_KNOTS('',3,(#61264,#61265,#61266,#61267,#61268,
#61269,#61270,#61271,#61272,#61273,#61274,#61275,#61276),.UNSPECIFIED.,
 .F.,.F.,(4,1,1,1,1,1,1,1,1,1,4),(-4.71239722187547,-4.56278933021375,-4.26359002987186,
-3.96439072952998,-3.66519142918809,-3.36599212884621,-3.06679282850432,
-2.76759352816244,-2.46839422782055,-2.01959527730772,-1.5707963267949),
 .UNSPECIFIED.);
#9544=B_SPLINE_CURVE_WITH_KNOTS('',3,(#61371,#61372,#61373,#61374,#61375,
#61376,#61377,#61378,#61379,#61380,#61381,#61382,#61383,#61384,#61385,#61386,
#61387,#61388,#61389,#61390,#61391,#61392,#61393),.UNSPECIFIED.,.T.,.F.,
(4,1,1,1,1,1,1,1,1,1,1,1,1,1,1,1,1,1,1,1,4),(1.5707963267949,2.01959527730772,
2.46839422782055,2.76759352816244,3.06679282850432,3.36599212884621,3.66519142918809,
3.96439072952998,4.26359002987186,4.56278933021375,4.86198863055563,5.16118793089752,
5.4603872312394,5.75958653158129,6.05878583192317,6.20838548209412,6.35798513226506,
6.65718443260694,6.95638373294883,7.40518268346166,7.85398163397448),
 .UNSPECIFIED.);
#9545=B_SPLINE_CURVE_WITH_KNOTS('',3,(#61777,#61778,#61779,#61780,#61781,
#61782),.UNSPECIFIED.,.F.,.F.,(4,2,4),(-0.000574846406454606,0.,0.0607530860081951),
 .UNSPECIFIED.);
#9546=B_SPLINE_CURVE_WITH_KNOTS('',3,(#61784,#61785,#61786,#61787),
 .UNSPECIFIED.,.F.,.F.,(4,4),(-5.27137424194997,-4.17539678580906),
 .UNSPECIFIED.);
#9547=B_SPLINE_CURVE_WITH_KNOTS('',3,(#61789,#61790,#61791,#61792,#61793,
#61794),.UNSPECIFIED.,.F.,.F.,(4,2,4),(0.,0.0605840139117386,0.0611572605565729),
 .UNSPECIFIED.);
#9548=B_SPLINE_CURVE_WITH_KNOTS('',3,(#61796,#61797,#61798,#61799,#61800,
#61801,#61802,#61803),.UNSPECIFIED.,.F.,.F.,(4,2,2,4),(0.,0.227902635573531,
0.336919078603134,0.368774184575231),.UNSPECIFIED.);
#9549=B_SPLINE_CURVE_WITH_KNOTS('',3,(#61805,#61806,#61807,#61808),
 .UNSPECIFIED.,.F.,.F.,(4,4),(4.45436462279932,4.99240640495978),
 .UNSPECIFIED.);
#9550=B_SPLINE_CURVE_WITH_KNOTS('',3,(#61809,#61810,#61811,#61812,#61813,
#61814,#61815,#61816,#61817,#61818),.UNSPECIFIED.,.F.,.F.,(4,2,2,2,4),(0.0513690276673274,
0.0678730027793273,0.112680650009656,0.165458501883772,0.226614451837517),
 .UNSPECIFIED.);
#9551=B_SPLINE_CURVE_WITH_KNOTS('',3,(#61843,#61844,#61845,#61846),
 .UNSPECIFIED.,.F.,.F.,(4,4),(-5.27136346380212,-4.17538600473639),
 .UNSPECIFIED.);
#9552=B_SPLINE_CURVE_WITH_KNOTS('',3,(#61848,#61849,#61850,#61851,#61852,
#61853),.UNSPECIFIED.,.F.,.F.,(4,2,4),(0.,0.0605840138982659,0.0611572605449778),
 .UNSPECIFIED.);
#9553=B_SPLINE_CURVE_WITH_KNOTS('',3,(#61855,#61856,#61857,#61858,#61859,
#61860,#61861,#61862),.UNSPECIFIED.,.F.,.F.,(4,2,2,4),(0.,0.227902635580422,
0.33691907860954,0.368774184575218),.UNSPECIFIED.);
#9554=B_SPLINE_CURVE_WITH_KNOTS('',3,(#61864,#61865,#61866,#61867),
 .UNSPECIFIED.,.F.,.F.,(4,4),(4.45435383946072,4.99239561273659),
 .UNSPECIFIED.);
#9555=B_SPLINE_CURVE_WITH_KNOTS('',3,(#61869,#61870,#61871,#61872,#61873,
#61874,#61875,#61876,#61877,#61878),.UNSPECIFIED.,.F.,.F.,(4,2,2,2,4),(-0.226614451833939,
-0.165458501895676,-0.112680650009599,-0.0678730027789982,-0.0513690276667455),
 .UNSPECIFIED.);
#9556=B_SPLINE_CURVE_WITH_KNOTS('',3,(#61879,#61880,#61881,#61882,#61883,
#61884),.UNSPECIFIED.,.F.,.F.,(4,2,4),(-0.060753086025328,0.,0.000574846408183778),
 .UNSPECIFIED.);
#9557=B_SPLINE_CURVE_WITH_KNOTS('',3,(#61907,#61908,#61909,#61910,#61911),
 .UNSPECIFIED.,.F.,.F.,(4,1,4),(8.48626880569866,9.5374231246245,11.0747361748566),
 .UNSPECIFIED.);
#9558=B_SPLINE_CURVE_WITH_KNOTS('',3,(#61914,#61915,#61916,#61917,#61918),
 .UNSPECIFIED.,.F.,.F.,(4,1,4),(-11.0747361748566,-9.5374231246245,-8.38443833695044),
 .UNSPECIFIED.);
#9559=B_SPLINE_CURVE_WITH_KNOTS('',3,(#61919,#61920,#61921,#61922),
 .UNSPECIFIED.,.F.,.F.,(4,4),(-8.48626880569866,-8.42427114782367),
 .UNSPECIFIED.);
#9560=B_SPLINE_CURVE_WITH_KNOTS('',3,(#61948,#61949,#61950,#61951,#61952,
#61953),.UNSPECIFIED.,.F.,.F.,(4,1,1,4),(-2.31999627410953E-6,0.644940971614267,
1.07490316602129,1.50486536042832),.UNSPECIFIED.);
#9561=B_SPLINE_CURVE_WITH_KNOTS('',3,(#61956,#61957,#61958,#61959,#61960,
#61961),.UNSPECIFIED.,.F.,.F.,(4,1,1,4),(-1.50486536042832,-1.07490316602129,
-0.644940971614267,8.85875174522468E-9),.UNSPECIFIED.);
#9562=B_SPLINE_CURVE_WITH_KNOTS('',3,(#61969,#61970,#61971,#61972),
 .UNSPECIFIED.,.F.,.F.,(4,4),(2.58846118365668,2.65046396645372),
 .UNSPECIFIED.);
#9563=B_SPLINE_CURVE_WITH_KNOTS('',3,(#61974,#61975,#61976,#61977,#61978),
 .UNSPECIFIED.,.F.,.F.,(4,1,4),(-2.31999443863861E-6,1.15298346196168,2.58846118365668),
 .UNSPECIFIED.);
#9564=B_SPLINE_CURVE_WITH_KNOTS('',3,(#61980,#61981,#61982,#61983,#61984),
 .UNSPECIFIED.,.F.,.F.,(4,1,4),(0.,0.644978914561078,1.50495080064252),
 .UNSPECIFIED.);
#9565=B_SPLINE_CURVE_WITH_KNOTS('',3,(#61985,#61986,#61987,#61988,#61989,
#61990,#61991),.UNSPECIFIED.,.F.,.F.,(4,1,1,1,4),(4.94996091805957,5.23536222982578,
5.80616485335821,6.37696747689064,6.94777010042307),.UNSPECIFIED.);
#9566=B_SPLINE_CURVE_WITH_KNOTS('',3,(#62053,#62054,#62055,#62056,#62057,
#62058,#62059),.UNSPECIFIED.,.F.,.F.,(4,1,1,1,4),(3.95106839828752,4.52186525716006,
4.8072636866506,5.37806054563167,5.94885740461274),.UNSPECIFIED.);
#9567=B_SPLINE_CURVE_WITH_KNOTS('',3,(#62062,#62063,#62064,#62065,#62066,
#62067,#62068,#62069,#62070,#62071,#62072,#62073,#62074,#62075,#62076,#62077,
#62078,#62079,#62080,#62081,#62082,#62083,#62084,#62085,#62086,#62087,#62088,
#62089,#62090,#62091,#62092,#62093,#62094,#62095,#62096,#62097,#62098,#62099,
#62100,#62101,#62102,#62103,#62104,#62105,#62106,#62107,#62108,#62109,#62110,
#62111,#62112,#62113,#62114,#62115,#62116,#62117,#62118,#62119,#62120,#62121,
#62122,#62123,#62124,#62125,#62126,#62127,#62128,#62129,#62130,#62131,#62132,
#62133,#62134),.UNSPECIFIED.,.F.,.F.,(4,3,3,3,3,3,3,3,3,3,3,3,3,3,3,3,3,
3,3,3,3,3,3,3,4),(-5.94885740461274,-5.86069693643025,-5.77088679319017,
-5.68121548115588,-5.59307645638642,-5.57724400806727,-5.49129151433642,
-5.40628539075431,-5.37781645040822,-5.2928587935222,-5.22646888161542,
-5.12018182868751,-5.01315048929543,-4.90734870686176,-4.88618634924932,
-4.80732469970942,-4.70560380101566,-4.60276419364428,-4.54687848896698,
-4.52188420367477,-4.41771788139319,-4.30863486714169,-4.19955185289018,
-4.04704298736789,-3.95106839817899),.UNSPECIFIED.);
#9568=B_SPLINE_CURVE_WITH_KNOTS('',3,(#62160,#62161,#62162,#62163,#62164,
#62165),.UNSPECIFIED.,.F.,.F.,(4,1,1,4),(-1.50508323116232,-0.860046566380066,
-0.430022123191898,8.85874817556907E-9),.UNSPECIFIED.);
#9569=B_SPLINE_CURVE_WITH_KNOTS('',3,(#62168,#62169,#62170,#62171,#62172,
#62173),.UNSPECIFIED.,.F.,.F.,(4,1,1,4),(-2.31999627050912E-6,0.430022123191898,
0.860046566380066,1.50508323116232),.UNSPECIFIED.);
#9570=B_SPLINE_CURVE_WITH_KNOTS('',3,(#62176,#62177,#62178,#62179,#62180),
 .UNSPECIFIED.,.F.,.F.,(4,1,4),(-1.71170449066025,-0.851718551084393,-0.206729096402498),
 .UNSPECIFIED.);
#9571=B_SPLINE_CURVE_WITH_KNOTS('',3,(#62205,#62206,#62207,#62208,#62209),
 .UNSPECIFIED.,.F.,.F.,(4,1,4),(-1.50495080064252,-0.644978914561078,0.),
 .UNSPECIFIED.);
#9572=B_SPLINE_CURVE_WITH_KNOTS('',3,(#62234,#62235,#62236,#62237,#62238),
 .UNSPECIFIED.,.F.,.F.,(4,1,4),(-2.57862308600535,-1.15298346196168,9.47324368820803E-9),
 .UNSPECIFIED.);
#9573=B_SPLINE_CURVE_WITH_KNOTS('',3,(#62239,#62240,#62241,#62242),
 .UNSPECIFIED.,.F.,.F.,(4,4),(2.57862308600535,2.69029783790316),
 .UNSPECIFIED.);
#9574=B_SPLINE_CURVE_WITH_KNOTS('',3,(#62283,#62284,#62285,#62286,#62287),
 .UNSPECIFIED.,.F.,.F.,(4,1,4),(-2.57862306394281,-1.15298346196168,9.47324703083255E-9),
 .UNSPECIFIED.);
#9575=B_SPLINE_CURVE_WITH_KNOTS('',3,(#62289,#62290,#62291,#62292),
 .UNSPECIFIED.,.F.,.F.,(4,4),(2.57862306394281,2.69029783790317),
 .UNSPECIFIED.);
#9576=B_SPLINE_CURVE_WITH_KNOTS('',3,(#62294,#62295,#62296,#62297),
 .UNSPECIFIED.,.F.,.F.,(4,4),(-5.2712893858124,-4.17531192673851),
 .UNSPECIFIED.);
#9577=B_SPLINE_CURVE_WITH_KNOTS('',3,(#62299,#62300,#62301,#62302,#62303),
 .UNSPECIFIED.,.F.,.F.,(4,1,4),(-11.0747361748565,-9.53742312462444,-8.38443833695038),
 .UNSPECIFIED.);
#9578=B_SPLINE_CURVE_WITH_KNOTS('',3,(#62307,#62308,#62309,#62310,#62311),
 .UNSPECIFIED.,.F.,.F.,(4,1,4),(-2.57862310024277,-1.15298346196168,9.47324497094032E-9),
 .UNSPECIFIED.);
#9579=B_SPLINE_CURVE_WITH_KNOTS('',3,(#62312,#62313,#62314,#62315),
 .UNSPECIFIED.,.F.,.F.,(4,4),(2.57862310024277,2.69029783790317),
 .UNSPECIFIED.);
#9580=B_SPLINE_CURVE_WITH_KNOTS('',3,(#62317,#62318,#62319,#62320),
 .UNSPECIFIED.,.F.,.F.,(4,4),(8.38443833694999,8.49611308884275),
 .UNSPECIFIED.);
#9581=B_SPLINE_CURVE_WITH_KNOTS('',3,(#62322,#62323,#62324,#62325,#62326),
 .UNSPECIFIED.,.F.,.F.,(4,1,4),(-11.0747361843298,-9.92175271289341,-8.49611308884275),
 .UNSPECIFIED.);
#9582=B_SPLINE_CURVE_WITH_KNOTS('',3,(#62330,#62331,#62332,#62333,#62334),
 .UNSPECIFIED.,.F.,.F.,(4,1,4),(-2.69029783626567,-1.15298346125989,9.47324711740778E-9),
 .UNSPECIFIED.);
#9583=B_SPLINE_CURVE_WITH_KNOTS('',3,(#62336,#62337,#62338,#62339),
 .UNSPECIFIED.,.F.,.F.,(4,4),(-5.24456940723389,-4.17431363002051),
 .UNSPECIFIED.);
#9584=B_SPLINE_CURVE_WITH_KNOTS('',3,(#62341,#62342,#62343,#62344),
 .UNSPECIFIED.,.F.,.F.,(4,4),(5.24456940723389,5.27029108627002),
 .UNSPECIFIED.);
#9585=B_SPLINE_CURVE_WITH_KNOTS('',3,(#62346,#62347,#62348,#62349,#62350),
 .UNSPECIFIED.,.F.,.F.,(4,1,4),(-9.47324123199628E-9,1.15298346196206,2.69029783790404),
 .UNSPECIFIED.);
#9586=B_SPLINE_CURVE_WITH_KNOTS('',3,(#62354,#62355,#62356,#62357,#62358),
 .UNSPECIFIED.,.F.,.F.,(4,1,4),(-2.57862306194136,-1.15298346125614,9.47324546639064E-9),
 .UNSPECIFIED.);
#9587=B_SPLINE_CURVE_WITH_KNOTS('',3,(#62360,#62361,#62362,#62363),
 .UNSPECIFIED.,.F.,.F.,(4,4),(2.57862306194136,2.69029783625691),
 .UNSPECIFIED.);
#9588=B_SPLINE_CURVE_WITH_KNOTS('',3,(#62365,#62366,#62367,#62368),
 .UNSPECIFIED.,.F.,.F.,(4,4),(-5.27130879387958,-4.17533133480784),
 .UNSPECIFIED.);
#9589=B_SPLINE_CURVE_WITH_KNOTS('',3,(#62369,#62370,#62371,#62372,#62373),
 .UNSPECIFIED.,.F.,.F.,(4,1,4),(-11.2201550062119,-9.68284195691921,-8.52985716994968),
 .UNSPECIFIED.);
#9590=B_SPLINE_CURVE_WITH_KNOTS('',3,(#62375,#62376,#62377,#62378,#62379),
 .UNSPECIFIED.,.F.,.F.,(4,1,4),(-2.69029783626566,-1.15298346125989,9.47324556754925E-9),
 .UNSPECIFIED.);
#9591=B_SPLINE_CURVE_WITH_KNOTS('',3,(#62381,#62382,#62383,#62384),
 .UNSPECIFIED.,.F.,.F.,(4,4),(-5.27137424194994,-4.17539678580906),
 .UNSPECIFIED.);
#9592=B_SPLINE_CURVE_WITH_KNOTS('',3,(#62386,#62387,#62388,#62389,#62390),
 .UNSPECIFIED.,.F.,.F.,(4,1,4),(-11.2196221181042,-9.68230906880774,-8.52932428183543),
 .UNSPECIFIED.);
#9593=B_SPLINE_CURVE_WITH_KNOTS('',3,(#62413,#62414,#62415,#62416,#62417,
#62418),.UNSPECIFIED.,.F.,.F.,(4,2,4),(-0.0611572605514445,-0.0605840139056089,
0.),.UNSPECIFIED.);
#9594=B_SPLINE_CURVE_WITH_KNOTS('',3,(#62420,#62421,#62422,#62423,#62424,
#62425,#62426,#62427,#62428,#62429),.UNSPECIFIED.,.F.,.F.,(4,2,2,2,4),(-0.357338823622728,
-0.315971023517638,-0.202638138270996,-0.0264825934181576,0.),
 .UNSPECIFIED.);
#9595=B_SPLINE_CURVE_WITH_KNOTS('',3,(#62431,#62432,#62433,#62434),
 .UNSPECIFIED.,.F.,.F.,(4,4),(4.45436462279932,4.99240640495978),
 .UNSPECIFIED.);
#9596=B_SPLINE_CURVE_WITH_KNOTS('',3,(#62436,#62437,#62438,#62439,#62440,
#62441,#62442,#62443,#62444,#62445),.UNSPECIFIED.,.F.,.F.,(4,2,2,2,4),(-0.226614451839263,
-0.165458501884473,-0.112680650009616,-0.0678730027791403,-0.0513690276667193),
 .UNSPECIFIED.);
#9597=B_SPLINE_CURVE_WITH_KNOTS('',3,(#62446,#62447,#62448,#62449,#62450,
#62451),.UNSPECIFIED.,.F.,.F.,(4,2,4),(-0.0607530860235367,0.,0.00057484640812516),
 .UNSPECIFIED.);
#9598=B_SPLINE_CURVE_WITH_KNOTS('',3,(#62495,#62496,#62497,#62498,#62499,
#62500,#62501,#62502,#62503,#62504,#62505,#62506,#62507,#62508,#62509,#62510,
#62511,#62512,#62513,#62514,#62515,#62516,#62517,#62518,#62519,#62520,#62521,
#62522,#62523,#62524,#62525,#62526,#62527,#62528,#62529,#62530,#62531,#62532,
#62533,#62534,#62535,#62536,#62537,#62538,#62539,#62540,#62541,#62542,#62543,
#62544,#62545,#62546,#62547,#62548,#62549,#62550,#62551,#62552,#62553,#62554,
#62555,#62556,#62557,#62558,#62559,#62560,#62561,#62562,#62563,#62564,#62565,
#62566,#62567),.UNSPECIFIED.,.F.,.F.,(4,3,3,3,3,3,3,3,3,3,3,3,3,3,3,3,3,
3,3,3,3,3,3,3,4),(-7.9466464122711,-7.85757426245866,-7.76709951843425,
-7.69816295633529,-7.60640515072815,-7.51504697731427,-7.42454212635978,
-7.37561227111267,-7.3508363202585,-7.24397791060106,-7.13602736376904,
-7.0270196075735,-7.01152845997615,-6.91723749819949,-6.82297570925328,
-6.80512855355305,-6.71012742819247,-6.67124592761005,-6.56069887569449,
-6.51971715131434,-6.40647264324666,-6.3204708011582,-6.19502812240143,
-6.0692197803777,-5.94885740461274),.UNSPECIFIED.);
#9599=B_SPLINE_CURVE_WITH_KNOTS('',3,(#62570,#62571,#62572,#62573,#62574,
#62575,#62576),.UNSPECIFIED.,.F.,.F.,(4,1,1,1,4),(5.94885740461274,6.5196542639437,
6.80505269360918,7.37584955294014,7.94664641093795),.UNSPECIFIED.);
#9600=B_SPLINE_CURVE_WITH_KNOTS('',3,(#62598,#62599,#62600,#62601,#62602),
 .UNSPECIFIED.,.F.,.F.,(4,1,4),(0.206729096402498,0.851718551084393,1.71170449066025),
 .UNSPECIFIED.);
#9601=B_SPLINE_CURVE_WITH_KNOTS('',3,(#62625,#62626,#62627,#62628,#62629),
 .UNSPECIFIED.,.F.,.F.,(4,1,4),(-2.31999444043195E-6,1.15298346125989,2.588461190451),
 .UNSPECIFIED.);
#9602=B_SPLINE_CURVE_WITH_KNOTS('',3,(#62630,#62631,#62632,#62633),
 .UNSPECIFIED.,.F.,.F.,(4,4),(-2.65046396614434,-2.588461190451),
 .UNSPECIFIED.);
#9603=B_SPLINE_CURVE_WITH_KNOTS('',3,(#62656,#62657,#62658,#62659,#62660),
 .UNSPECIFIED.,.F.,.F.,(4,1,4),(8.63115475890037,9.68230906880774,11.2196221181042),
 .UNSPECIFIED.);
#9604=B_SPLINE_CURVE_WITH_KNOTS('',3,(#62662,#62663,#62664,#62665),
 .UNSPECIFIED.,.F.,.F.,(4,4),(-8.63115475890038,-8.56915709422042),
 .UNSPECIFIED.);
#9605=B_SPLINE_CURVE_WITH_KNOTS('',3,(#62686,#62687,#62688,#62689,#62690),
 .UNSPECIFIED.,.F.,.F.,(4,1,4),(-2.31999627648449E-6,0.85992278978735,1.50486662212507),
 .UNSPECIFIED.);
#9606=B_SPLINE_CURVE_WITH_KNOTS('',3,(#62695,#62696,#62697,#62698,#62699),
 .UNSPECIFIED.,.F.,.F.,(4,1,4),(-1.50486662212507,-0.85992278978735,8.85875352486674E-9),
 .UNSPECIFIED.);
#9607=B_SPLINE_CURVE_WITH_KNOTS('',3,(#62714,#62715,#62716,#62717,#62718,
#62719,#62720,#62721,#62722,#62723,#62724,#62725,#62726,#62727,#62728,#62729,
#62730,#62731,#62732,#62733,#62734,#62735,#62736,#62737,#62738,#62739,#62740,
#62741,#62742,#62743,#62744,#62745,#62746,#62747,#62748,#62749,#62750,#62751,
#62752,#62753,#62754,#62755,#62756,#62757,#62758,#62759,#62760,#62761,#62762,
#62763,#62764,#62765,#62766,#62767,#62768,#62769,#62770,#62771,#62772,#62773,
#62774,#62775,#62776,#62777,#62778,#62779,#62780,#62781,#62782,#62783,#62784,
#62785,#62786,#62787,#62788,#62789,#62790,#62791,#62792,#62793,#62794,#62795,
#62796,#62797,#62798),.UNSPECIFIED.,.F.,.F.,(4,3,3,3,3,3,3,3,3,3,3,3,3,
3,3,3,3,3,3,3,3,3,3,3,3,3,3,3,4),(-6.94777010041813,-6.85455068095993,-6.7597783456048,
-6.73904767757639,-6.63572828455797,-6.53287577437175,-6.43126906112607,
-6.38027211805784,-6.37674668089816,-6.29068294601615,-6.20469800416214,
-6.16409279217385,-6.08059986970485,-5.99767656546386,-5.9488568756778,
-5.86487907045254,-5.80596511193711,-5.72281846929729,-5.63898221754222,
-5.61006206702274,-5.51578314435451,-5.42071477668994,-5.32637474331624,
-5.26492483575683,-5.23521811218339,-5.16148034851913,-5.08715409816934,
-5.0117930664328,-4.94996091806724),.UNSPECIFIED.);
#9608=B_SPLINE_CURVE_WITH_KNOTS('',3,(#62802,#62803,#62804,#62805,#62806,
#62807,#62808,#62809,#62810,#62811,#62812,#62813,#62814,#62815,#62816,#62817,
#62818,#62819,#62820,#62821,#62822,#62823,#62824,#62825,#62826,#62827,#62828,
#62829,#62830,#62831,#62832,#62833,#62834,#62835,#62836,#62837,#62838,#62839,
#62840,#62841,#62842,#62843,#62844,#62845,#62846,#62847,#62848,#62849,#62850,
#62851,#62852,#62853,#62854,#62855,#62856,#62857,#62858,#62859,#62860,#62861,
#62862,#62863,#62864,#62865,#62866,#62867,#62868,#62869,#62870,#62871,#62872,
#62873,#62874,#62875,#62876,#62877,#62878,#62879,#62880),.UNSPECIFIED.,
 .F.,.F.,(4,3,3,3,3,3,3,3,3,3,3,3,3,3,3,3,3,3,3,3,3,3,3,3,3,3,4),(-6.94777010041813,
-6.80589560482806,-6.76360702598265,-6.73694709261346,-6.61205678580534,
-6.48749262436621,-6.38027211805784,-6.37694173120473,-6.29065355376979,
-6.20461705062999,-6.16409279217385,-6.09147809619365,-6.01442162734269,
-5.9488568756778,-5.84777694274893,-5.74655744024335,-5.64670293342734,
-5.61006206702274,-5.52775431802231,-5.52098532502223,-5.43849985069856,
-5.3517123432277,-5.26492483575683,-5.17566714511047,-5.08613487358801,
-4.99780308351251,-4.94996091806794),.UNSPECIFIED.);
#9609=B_SPLINE_CURVE_WITH_KNOTS('',3,(#62884,#62885,#62886,#62887,#62888,
#62889,#62890,#62891,#62892,#62893,#62894,#62895,#62896,#62897,#62898,#62899,
#62900,#62901,#62902,#62903,#62904,#62905,#62906,#62907,#62908,#62909,#62910,
#62911,#62912,#62913,#62914,#62915,#62916,#62917,#62918,#62919,#62920,#62921,
#62922,#62923,#62924,#62925,#62926,#62927,#62928,#62929,#62930,#62931,#62932,
#62933,#62934,#62935,#62936,#62937,#62938,#62939,#62940,#62941,#62942,#62943,
#62944,#62945,#62946,#62947,#62948,#62949,#62950,#62951,#62952,#62953,#62954,
#62955,#62956,#62957,#62958,#62959,#62960,#62961,#62962,#62963,#62964,#62965,
#62966,#62967,#62968),.UNSPECIFIED.,.F.,.F.,(4,3,3,3,3,3,3,3,3,3,3,3,3,
3,3,3,3,3,3,3,3,3,3,3,3,3,3,3,4),(-6.94777010041813,-6.85454181347915,-6.75976365757834,
-6.7390476775764,-6.63588829170932,-6.53319704934699,-6.43174682810582,
-6.38027211805784,-6.37674963803592,-6.29084061678197,-6.20501554909631,
-6.16409279217385,-6.08058380241542,-5.99764526758615,-5.9488568756778,
-5.86489026670279,-5.80596772458804,-5.72283239635377,-5.63900785451474,
-5.61006206702274,-5.51573905289243,-5.42062447789676,-5.32624375888541,
-5.26492483575683,-5.2352185988914,-5.16146456719849,-5.08712162926062,
-5.01174427267612,-4.94996091806794),.UNSPECIFIED.);
#9610=B_SPLINE_CURVE_WITH_KNOTS('',3,(#62970,#62971,#62972,#62973,#62974,
#62975,#62976,#62977,#62978,#62979,#62980,#62981,#62982,#62983,#62984,#62985,
#62986,#62987,#62988,#62989,#62990,#62991,#62992,#62993,#62994,#62995,#62996,
#62997,#62998,#62999,#63000,#63001,#63002,#63003,#63004,#63005,#63006,#63007,
#63008,#63009,#63010,#63011,#63012,#63013,#63014,#63015,#63016,#63017,#63018,
#63019,#63020,#63021,#63022,#63023,#63024,#63025,#63026,#63027,#63028,#63029,
#63030,#63031,#63032,#63033,#63034,#63035,#63036,#63037,#63038,#63039,#63040,
#63041,#63042,#63043,#63044,#63045,#63046,#63047,#63048,#63049,#63050,#63051,
#63052,#63053,#63054),.UNSPECIFIED.,.F.,.F.,(4,3,3,3,3,3,3,3,3,3,3,3,3,
3,3,3,3,3,3,3,3,3,3,3,3,3,3,3,4),(-6.94777010041813,-6.85455068095717,-6.75977834560242,
-6.73904767757639,-6.6357282845608,-6.53287577437409,-6.43126906112939,
-6.38027211805784,-6.37674668090181,-6.29068294602099,-6.20469800415847,
-6.16409279217385,-6.08059986969781,-5.99767656546224,-5.9488568756778,
-5.86487907045173,-5.80596511193947,-5.72281846930225,-5.63898221754871,
-5.61006206702274,-5.51578314435305,-5.42071477668969,-5.32637474331668,
-5.26492483575683,-5.23521811218446,-5.16148034852062,-5.08715409817098,
-5.01179306643379,-4.94996091806794),.UNSPECIFIED.);
#9611=B_SPLINE_CURVE_WITH_KNOTS('',3,(#63078,#63079,#63080,#63081,#63082,
#63083),.UNSPECIFIED.,.F.,.F.,(4,2,4),(0.,0.0605840131572603,0.0611572605613591),
 .UNSPECIFIED.);
#9612=B_SPLINE_CURVE_WITH_KNOTS('',3,(#63085,#63086,#63087,#63088,#63089,
#63090,#63091,#63092),.UNSPECIFIED.,.F.,.F.,(4,2,2,4),(0.,0.187166895768669,
0.311915370525459,0.366032938932827),.UNSPECIFIED.);
#9613=B_SPLINE_CURVE_WITH_KNOTS('',3,(#63094,#63095,#63096,#63097),
 .UNSPECIFIED.,.F.,.F.,(4,4),(4.45429916952982,4.99234094280284),
 .UNSPECIFIED.);
#9614=B_SPLINE_CURVE_WITH_KNOTS('',3,(#63099,#63100,#63101,#63102,#63103,
#63104,#63105,#63106,#63107,#63108),.UNSPECIFIED.,.F.,.F.,(4,2,2,2,4),(-0.226614491360217,
-0.165458328163798,-0.112680756090081,-0.0678730247966914,-0.0513690276540772),
 .UNSPECIFIED.);
#9615=B_SPLINE_CURVE_WITH_KNOTS('',3,(#63109,#63110,#63111,#63112,#63113,
#63114),.UNSPECIFIED.,.F.,.F.,(4,2,4),(-0.0607530852768461,0.,0.000574847168889258),
 .UNSPECIFIED.);
#9616=B_SPLINE_CURVE_WITH_KNOTS('',3,(#63136,#63137,#63138,#63139,#63140),
 .UNSPECIFIED.,.F.,.F.,(4,1,4),(8.63168765941227,9.68284195691921,11.2201550062119),
 .UNSPECIFIED.);
#9617=B_SPLINE_CURVE_WITH_KNOTS('',3,(#63141,#63142,#63143,#63144),
 .UNSPECIFIED.,.F.,.F.,(4,4),(-8.63168765941227,-8.56968998446986),
 .UNSPECIFIED.);
#9618=B_SPLINE_CURVE_WITH_KNOTS('',3,(#63178,#63179,#63180,#63181,#63182,
#63183),.UNSPECIFIED.,.F.,.F.,(4,1,1,4),(0.207327684708445,0.637351476682114,
1.06737526865578,1.71241095661629),.UNSPECIFIED.);
#9619=B_SPLINE_CURVE_WITH_KNOTS('',3,(#63185,#63186,#63187,#63188,#63189,
#63190),.UNSPECIFIED.,.F.,.F.,(4,1,1,4),(-1.71241095661629,-1.06737526865578,
-0.637351476682114,-0.207327684708445),.UNSPECIFIED.);
#9620=B_SPLINE_CURVE_WITH_KNOTS('',3,(#63212,#63213,#63214,#63215,#63216),
 .UNSPECIFIED.,.F.,.F.,(4,1,4),(-2.31999443730624E-6,1.15298346125614,2.58846116811262),
 .UNSPECIFIED.);
#9621=B_SPLINE_CURVE_WITH_KNOTS('',3,(#63217,#63218,#63219,#63220),
 .UNSPECIFIED.,.F.,.F.,(4,4),(2.58846116811262,2.65046396240323),
 .UNSPECIFIED.);
#9622=B_SPLINE_CURVE_WITH_KNOTS('',3,(#63247,#63248,#63249,#63250,#63251,
#63252),.UNSPECIFIED.,.F.,.F.,(4,1,1,4),(-1.5048844204457,-1.0749174431755,
-0.644950465905299,0.),.UNSPECIFIED.);
#9623=B_SPLINE_CURVE_WITH_KNOTS('',3,(#63255,#63256,#63257,#63258,#63259,
#63260),.UNSPECIFIED.,.F.,.F.,(4,1,1,4),(0.,0.644950465905299,1.0749174431755,
1.5048844204457),.UNSPECIFIED.);
#9624=B_SPLINE_CURVE_WITH_KNOTS('',3,(#63282,#63283,#63284,#63285,#63286,
#63287),.UNSPECIFIED.,.F.,.F.,(4,2,4),(-0.0607530860059133,0.,0.000574846391605915),
 .UNSPECIFIED.);
#9625=B_SPLINE_CURVE_WITH_KNOTS('',3,(#63288,#63289,#63290,#63291,#63292),
 .UNSPECIFIED.,.F.,.F.,(4,1,4),(-2.65046396791738,-1.15298346196206,2.3199944317628E-6),
 .UNSPECIFIED.);
#9626=B_SPLINE_CURVE_WITH_KNOTS('',3,(#63340,#63341,#63342,#63343,#63344,
#63345,#63346),.UNSPECIFIED.,.F.,.F.,(4,1,1,1,4),(4.94996091805913,5.2353622298247,
5.80616485335585,6.37696747688699,6.94777010041813),.UNSPECIFIED.);
#9627=B_SPLINE_CURVE_WITH_KNOTS('',3,(#63373,#63374,#63375,#63376,#63377),
 .UNSPECIFIED.,.F.,.F.,(4,1,4),(-1.50495079029869,-0.85997188017068,0.),
 .UNSPECIFIED.);
#9628=B_SPLINE_CURVE_WITH_KNOTS('',3,(#63380,#63381,#63382,#63383,#63384),
 .UNSPECIFIED.,.F.,.F.,(4,1,4),(0.,0.85997188017068,1.50495079029869),
 .UNSPECIFIED.);
#9629=B_SPLINE_CURVE_WITH_KNOTS('',3,(#63411,#63412,#63413,#63414,#63415),
 .UNSPECIFIED.,.F.,.F.,(4,1,4),(8.48627499119542,9.92175271289341,11.074738494851),
 .UNSPECIFIED.);
#9630=B_SPLINE_CURVE_WITH_KNOTS('',3,(#63416,#63417,#63418,#63419),
 .UNSPECIFIED.,.F.,.F.,(4,4),(8.42427220840034,8.48627499119542),
 .UNSPECIFIED.);
#9631=B_SPLINE_CURVE_WITH_KNOTS('',3,(#63423,#63424,#63425,#63426,#63427),
 .UNSPECIFIED.,.F.,.F.,(4,1,4),(-1.71167751650087,-0.851711715694741,-0.206737365090144),
 .UNSPECIFIED.);
#9632=B_SPLINE_CURVE_WITH_KNOTS('',3,(#63456,#63457,#63458,#63459,#63460),
 .UNSPECIFIED.,.F.,.F.,(4,1,4),(-1.50488716129577,-0.644951640555328,0.),
 .UNSPECIFIED.);
#9633=B_SPLINE_CURVE_WITH_KNOTS('',3,(#63461,#63462,#63463,#63464,#63465),
 .UNSPECIFIED.,.F.,.F.,(4,1,4),(0.,0.644951640555328,1.50488716129577),
 .UNSPECIFIED.);
#9634=B_SPLINE_CURVE_WITH_KNOTS('',3,(#63487,#63488,#63489,#63490,#63491),
 .UNSPECIFIED.,.F.,.F.,(4,1,4),(-2.31999443914823E-6,1.15298346196168,2.5884611924141),
 .UNSPECIFIED.);
#9635=B_SPLINE_CURVE_WITH_KNOTS('',3,(#63492,#63493,#63494,#63495),
 .UNSPECIFIED.,.F.,.F.,(4,4),(2.5884611924141,2.65046396791737),
 .UNSPECIFIED.);
#9636=B_SPLINE_CURVE_WITH_KNOTS('',3,(#63497,#63498,#63499,#63500,#63501,
#63502,#63503),.UNSPECIFIED.,.F.,.F.,(4,1,1,1,4),(4.94996091841328,5.52076354159657,
6.09156616512519,6.37696747688951,6.94777010041813),.UNSPECIFIED.);
#9637=B_SPLINE_CURVE_WITH_KNOTS('',3,(#63571,#63572,#63573,#63574,#63575,
#63576),.UNSPECIFIED.,.F.,.F.,(4,2,4),(0.,0.0605840131564532,0.0611572605603469),
 .UNSPECIFIED.);
#9638=B_SPLINE_CURVE_WITH_KNOTS('',3,(#63578,#63579,#63580,#63581,#63582,
#63583,#63584,#63585),.UNSPECIFIED.,.F.,.F.,(4,2,2,4),(0.,0.187166892255563,
0.311915369245822,0.366032938789283),.UNSPECIFIED.);
#9639=B_SPLINE_CURVE_WITH_KNOTS('',3,(#63587,#63588,#63589,#63590),
 .UNSPECIFIED.,.F.,.F.,(4,4),(4.45427976145965,4.99232153473166),
 .UNSPECIFIED.);
#9640=B_SPLINE_CURVE_WITH_KNOTS('',3,(#63592,#63593,#63594,#63595,#63596,
#63597,#63598,#63599,#63600,#63601),.UNSPECIFIED.,.F.,.F.,(4,2,2,2,4),(-0.226614491339767,
-0.165458328247082,-0.112680756037836,-0.0678730247858201,-0.0513690276539791),
 .UNSPECIFIED.);
#9641=B_SPLINE_CURVE_WITH_KNOTS('',3,(#63602,#63603,#63604,#63605,#63606,
#63607),.UNSPECIFIED.,.F.,.F.,(4,2,4),(-0.0607530852467481,0.,0.000574847167102605),
 .UNSPECIFIED.);
#9642=B_SPLINE_CURVE_WITH_KNOTS('',3,(#63630,#63631,#63632,#63633,#63634),
 .UNSPECIFIED.,.F.,.F.,(4,1,4),(8.48626882609487,9.53742312462444,11.0747361748565),
 .UNSPECIFIED.);
#9643=B_SPLINE_CURVE_WITH_KNOTS('',3,(#63636,#63637,#63638,#63639),
 .UNSPECIFIED.,.F.,.F.,(4,4),(-8.48626882609487,-8.42427115133595),
 .UNSPECIFIED.);
#9644=B_SPLINE_CURVE_WITH_KNOTS('',3,(#63665,#63666,#63667,#63668,#63669,
#63670),.UNSPECIFIED.,.F.,.F.,(4,1,1,4),(-2.3199962741138E-6,0.644939523401962,
1.07490075233412,1.50486198126628),.UNSPECIFIED.);
#9645=B_SPLINE_CURVE_WITH_KNOTS('',3,(#63672,#63673,#63674,#63675,#63676,
#63677),.UNSPECIFIED.,.F.,.F.,(4,1,1,4),(-1.50486198126628,-1.07490075233412,
-0.644939523401962,8.8587499697081E-9),.UNSPECIFIED.);
#9646=B_SPLINE_CURVE_WITH_KNOTS('',3,(#63683,#63684,#63685,#63686),
 .UNSPECIFIED.,.F.,.F.,(4,4),(2.58846117008605,2.65046396418562),
 .UNSPECIFIED.);
#9647=B_SPLINE_CURVE_WITH_KNOTS('',3,(#63688,#63689,#63690,#63691,#63692),
 .UNSPECIFIED.,.F.,.F.,(4,1,4),(-2.31999443732384E-6,1.15298346196168,2.58846117008605),
 .UNSPECIFIED.);
#9648=B_SPLINE_CURVE_WITH_KNOTS('',3,(#63694,#63695,#63696,#63697,#63698,
#63699),.UNSPECIFIED.,.F.,.F.,(4,1,1,4),(0.,0.429964410955918,0.859928821911836,
1.50487543834571),.UNSPECIFIED.);
#9649=B_SPLINE_CURVE_WITH_KNOTS('',3,(#63700,#63701,#63702,#63703,#63704,
#63705,#63706),.UNSPECIFIED.,.F.,.F.,(4,1,1,1,4),(4.94996091865684,5.23536222983225,
5.80616485336088,6.3769674768895,6.94777009982943),.UNSPECIFIED.);
#9650=B_SPLINE_CURVE_WITH_KNOTS('',3,(#63734,#63735,#63736,#63737,#63738,
#63739),.UNSPECIFIED.,.F.,.F.,(4,1,1,4),(-1.50487543834571,-0.859928821911836,
-0.429964410955918,0.),.UNSPECIFIED.);
#9651=B_SPLINE_CURVE_WITH_KNOTS('',3,(#63881,#63882,#63883,#63884,#63885),
 .UNSPECIFIED.,.F.,.F.,(4,1,4),(0.206737365090144,0.851711715694741,1.71167751650087),
 .UNSPECIFIED.);
#9652=B_SPLINE_CURVE_WITH_KNOTS('',3,(#63917,#63918,#63919,#63920),
 .UNSPECIFIED.,.F.,.F.,(4,4),(4.45328146709785,4.99132324919268),
 .UNSPECIFIED.);
#9653=B_SPLINE_CURVE_WITH_KNOTS('',3,(#63921,#63922,#63923,#63924,#63925,
#63926,#63927,#63928,#63929,#63930),.UNSPECIFIED.,.F.,.F.,(4,2,2,2,4),(0.0513690276671499,
0.0678730023326088,0.112680647857527,0.165458505409967,0.226614451037283),
 .UNSPECIFIED.);
#9654=B_SPLINE_CURVE_WITH_KNOTS('',3,(#63932,#63933,#63934,#63935,#63936,
#63937),.UNSPECIFIED.,.F.,.F.,(4,2,4),(-0.0611572605516308,-0.0605840139211158,
0.),.UNSPECIFIED.);
#9655=B_SPLINE_CURVE_WITH_KNOTS('',3,(#63938,#63939,#63940,#63941,#63942,
#63943,#63944,#63945,#63946,#63947),.UNSPECIFIED.,.F.,.F.,(4,2,2,2,4),(-0.357336678121665,
-0.315971745211139,-0.202641379507773,-0.026488271066986,0.),
 .UNSPECIFIED.);
#9656=B_SPLINE_CURVE_WITH_KNOTS('',3,(#63969,#63970,#63971,#63972,#63973),
 .UNSPECIFIED.,.F.,.F.,(4,1,4),(-2.31999444274574E-6,1.15298346125989,2.58846118169352),
 .UNSPECIFIED.);
#9657=B_SPLINE_CURVE_WITH_KNOTS('',3,(#63974,#63975,#63976,#63977),
 .UNSPECIFIED.,.F.,.F.,(4,4),(-2.65046396468069,-2.58846118169352),
 .UNSPECIFIED.);
#9658=B_SPLINE_CURVE_WITH_KNOTS('',3,(#64092,#64093,#64094,#64095,#64096,
#64097,#64098,#64099,#64100,#64101,#64102,#64103,#64104,#64105,#64106,#64107,
#64108,#64109,#64110,#64111,#64112,#64113,#64114,#64115,#64116,#64117,#64118,
#64119,#64120,#64121,#64122,#64123,#64124,#64125,#64126,#64127,#64128,#64129,
#64130,#64131,#64132,#64133,#64134,#64135,#64136,#64137,#64138,#64139,#64140,
#64141,#64142,#64143,#64144,#64145,#64146,#64147,#64148,#64149,#64150,#64151,
#64152,#64153,#64154,#64155,#64156,#64157,#64158,#64159,#64160,#64161,#64162,
#64163,#64164,#64165,#64166,#64167,#64168,#64169,#64170,#64171,#64172,#64173,
#64174,#64175,#64176,#64177,#64178,#64179,#64180,#64181,#64182,#64183,#64184,
#64185,#64186,#64187,#64188,#64189,#64190,#64191,#64192,#64193,#64194,#64195,
#64196,#64197,#64198,#64199,#64200,#64201,#64202,#64203,#64204,#64205,#64206,
#64207,#64208,#64209,#64210,#64211,#64212,#64213,#64214,#64215,#64216,#64217,
#64218),.UNSPECIFIED.,.F.,.F.,(4,3,3,3,3,3,3,3,3,3,3,3,3,3,3,3,3,3,3,3,
3,3,3,3,3,3,3,3,3,3,3,3,3,3,3,3,3,3,3,3,3,3,4),(-2.17999453962578,-2.10063266362907,
-2.091873957159,-2.01231930078082,-1.95509746167078,-1.90351425826644,-1.89240573164408,
-1.81344737679712,-1.73464452329454,-1.65646152356078,-1.63044969136215,
-1.6216998126514,-1.61230671184185,-1.55454458790052,-1.47662686180423,
-1.39823531237996,-1.31993995231118,-1.24652491490679,-1.21899427588014,
-1.20849379017684,-1.20113016655519,-1.1237192789258,-1.04649202180132,
-1.0262798026936,-0.948763719975306,-0.871406694475355,-0.825979128285647,
-0.804255152325434,-0.792531137980725,-0.715983069040475,-0.639396489760505,
-0.563554944822673,-0.507986164957696,-0.444487894337984,-0.41670740094186,
-0.39866282444285,-0.390504338414556,-0.315310840123394,-0.236483130092546,
-0.160978626758254,-0.086113044186597,-0.0125791979644417,0.),
 .UNSPECIFIED.);
#9659=B_SPLINE_CURVE_WITH_KNOTS('',3,(#64219,#64220,#64221,#64222,#64223,
#64224,#64225,#64226,#64227,#64228,#64229,#64230,#64231,#64232,#64233,#64234,
#64235,#64236,#64237,#64238,#64239,#64240,#64241,#64242,#64243,#64244,#64245,
#64246,#64247,#64248,#64249,#64250,#64251,#64252,#64253,#64254,#64255,#64256,
#64257,#64258,#64259,#64260,#64261,#64262,#64263,#64264,#64265,#64266,#64267,
#64268,#64269,#64270,#64271,#64272,#64273,#64274,#64275,#64276,#64277,#64278,
#64279,#64280,#64281,#64282,#64283,#64284,#64285,#64286,#64287,#64288,#64289,
#64290,#64291,#64292,#64293,#64294,#64295,#64296,#64297,#64298,#64299,#64300,
#64301,#64302,#64303,#64304,#64305,#64306,#64307,#64308,#64309,#64310,#64311,
#64312,#64313,#64314,#64315,#64316,#64317,#64318,#64319,#64320,#64321,#64322,
#64323,#64324,#64325,#64326,#64327,#64328,#64329,#64330,#64331,#64332,#64333,
#64334,#64335,#64336,#64337,#64338,#64339,#64340,#64341,#64342,#64343,#64344,
#64345),.UNSPECIFIED.,.F.,.F.,(4,3,3,3,3,3,3,3,3,3,3,3,3,3,3,3,3,3,3,3,
3,3,3,3,3,3,3,3,3,3,3,3,3,3,3,3,3,3,3,3,3,3,4),(-2.18372485524367,-2.10640481126137,
-2.03131125946134,-1.95573524274359,-1.93194649951181,-1.92202410445497,
-1.91170450508302,-1.83269909010297,-1.7564214218189,-1.68041659703098,
-1.66133200299936,-1.65026380760144,-1.59568284516281,-1.51987264985015,
-1.4432085302279,-1.36615368002357,-1.29307850985005,-1.26567532103498,
-1.25313620515419,-1.24522285927348,-1.1676749738264,-1.08973332226631,
-1.07385299932949,-0.996301755750286,-0.918414341014846,-0.871341951742027,
-0.850305870621321,-0.841791405545423,-0.832528469227403,-0.75420385700067,
-0.675433230828789,-0.596813388080105,-0.541835226832292,-0.474105823478256,
-0.444474209510865,-0.426199436176823,-0.417758785285843,-0.33948922786048,
-0.260283150602071,-0.18057131451815,-0.101123636762481,-0.0227242047039516,
0.),.UNSPECIFIED.);
#9660=B_SPLINE_CURVE_WITH_KNOTS('',3,(#64414,#64415,#64416,#64417,#64418,
#64419,#64420,#64421,#64422,#64423,#64424,#64425,#64426,#64427,#64428,#64429,
#64430,#64431,#64432,#64433,#64434,#64435,#64436,#64437,#64438,#64439,#64440,
#64441,#64442,#64443,#64444,#64445,#64446,#64447,#64448,#64449,#64450,#64451,
#64452,#64453,#64454,#64455,#64456,#64457,#64458,#64459,#64460,#64461,#64462,
#64463,#64464,#64465,#64466,#64467,#64468,#64469,#64470,#64471,#64472,#64473,
#64474,#64475,#64476,#64477,#64478,#64479,#64480,#64481,#64482,#64483,#64484,
#64485,#64486,#64487,#64488,#64489,#64490,#64491,#64492),.UNSPECIFIED.,
 .F.,.F.,(4,3,3,3,3,3,3,3,3,3,3,3,3,3,3,3,3,3,3,3,3,3,3,3,3,3,4),(-8.28218627679832,
-8.20169292244768,-8.12106721966121,-8.04117813302801,-7.97899102691001,
-7.95058280824722,-7.87166320777918,-7.79148833532417,-7.71110290373465,
-7.6311884763772,-7.61346320952264,-7.53323731961839,-7.45313939207039,
-7.43689242612622,-7.35664991813127,-7.29001895588479,-7.21000395222543,
-7.12971248777295,-7.04986647139956,-6.99609779867531,-6.91598607479632,
-6.89381082847905,-6.8137168964314,-6.75159715694291,-6.68301147408802,
-6.64148280719229,-6.62822738408382),.UNSPECIFIED.);
#9661=B_SPLINE_CURVE_WITH_KNOTS('',3,(#64494,#64495,#64496,#64497,#64498,
#64499,#64500,#64501,#64502,#64503,#64504,#64505,#64506,#64507,#64508,#64509,
#64510,#64511,#64512,#64513,#64514,#64515,#64516,#64517,#64518,#64519,#64520,
#64521,#64522,#64523,#64524,#64525,#64526,#64527,#64528,#64529,#64530,#64531,
#64532,#64533,#64534,#64535,#64536,#64537,#64538,#64539,#64540,#64541,#64542,
#64543,#64544,#64545,#64546,#64547,#64548,#64549,#64550,#64551,#64552,#64553,
#64554,#64555,#64556,#64557,#64558,#64559,#64560,#64561,#64562,#64563,#64564,
#64565,#64566,#64567,#64568,#64569,#64570,#64571,#64572,#64573,#64574,#64575,
#64576,#64577,#64578,#64579,#64580,#64581,#64582,#64583,#64584,#64585,#64586,
#64587,#64588,#64589,#64590,#64591,#64592,#64593,#64594,#64595,#64596,#64597,
#64598,#64599,#64600,#64601,#64602,#64603,#64604,#64605,#64606,#64607,#64608,
#64609,#64610,#64611,#64612,#64613,#64614,#64615,#64616,#64617,#64618,#64619,
#64620,#64621,#64622,#64623,#64624,#64625,#64626,#64627,#64628,#64629,#64630,
#64631,#64632,#64633,#64634,#64635,#64636,#64637,#64638,#64639,#64640,#64641,
#64642,#64643,#64644,#64645,#64646,#64647,#64648,#64649,#64650,#64651,#64652,
#64653,#64654,#64655,#64656,#64657,#64658,#64659,#64660,#64661,#64662,#64663,
#64664,#64665,#64666,#64667,#64668),.UNSPECIFIED.,.F.,.F.,(4,3,3,3,3,3,
3,3,3,3,3,3,3,3,3,3,3,3,3,3,3,3,3,3,3,3,3,3,3,3,3,3,3,3,3,3,3,3,3,3,3,3,
3,3,3,3,3,3,3,3,3,3,3,3,3,3,3,3,4),(-6.60475875209394,-6.58310038414192,
-6.53746941762518,-6.46734709883472,-6.38716674845838,-6.37725009240076,
-6.29742147302148,-6.21718394473677,-6.15615884057328,-6.07526907322315,
-5.9950398840319,-5.91381982760234,-5.83259977117277,-5.8134238068869,-5.73475512678213,
-5.65246555189028,-5.57221692209262,-5.48890687465367,-5.40990936279436,
-5.40559682721471,-5.32558342163483,-5.28850512381517,-5.2087518161826,
-5.12865364516926,-5.04890682581051,-4.98418318714666,-4.90446255300372,
-4.82463877647798,-4.74537568044192,-4.66550794648424,-4.58578539554942,
-4.559484745265,-4.48050032791252,-4.40073625944101,-4.32110097263846,-4.24240676722646,
-4.20416143228768,-4.13427805555411,-4.05596954022464,-3.97677429561084,
-3.89724132793884,-3.81809184744973,-3.74015669692834,-3.70971216734844,
-3.66557074062534,-3.58753484842769,-3.50833229563456,-3.42903494666437,
-3.35047521573115,-3.28643189981048,-3.20749490400406,-3.12949821258403,
-3.05067703552976,-2.9716640523965,-2.89314240828441,-2.86489467266987,
-2.78647378803261,-2.70718175898026,-2.6278897299279),.UNSPECIFIED.);
#9662=B_SPLINE_CURVE_WITH_KNOTS('',3,(#64671,#64672,#64673,#64674,#64675,
#64676,#64677,#64678,#64679,#64680,#64681,#64682,#64683,#64684,#64685,#64686),
 .UNSPECIFIED.,.F.,.F.,(4,3,3,3,3,4),(-0.0359046274749819,-0.0357373982878779,
-0.0224344952039362,-0.0179160747775488,-0.00462092812078184,0.),
 .UNSPECIFIED.);
#9663=B_SPLINE_CURVE_WITH_KNOTS('',3,(#66140,#66141,#66142,#66143,#66144,
#66145,#66146,#66147,#66148,#66149,#66150,#66151,#66152,#66153,#66154,#66155,
#66156,#66157,#66158,#66159,#66160,#66161,#66162,#66163,#66164,#66165,#66166,
#66167,#66168,#66169,#66170,#66171,#66172,#66173,#66174,#66175,#66176,#66177,
#66178,#66179,#66180,#66181,#66182,#66183,#66184,#66185,#66186,#66187,#66188,
#66189,#66190,#66191,#66192,#66193,#66194,#66195,#66196,#66197,#66198,#66199,
#66200,#66201,#66202,#66203,#66204,#66205,#66206,#66207,#66208,#66209,#66210,
#66211,#66212,#66213,#66214,#66215,#66216,#66217,#66218,#66219,#66220,#66221,
#66222,#66223,#66224,#66225,#66226,#66227,#66228,#66229,#66230,#66231,#66232,
#66233,#66234,#66235,#66236,#66237,#66238,#66239,#66240,#66241,#66242,#66243,
#66244,#66245,#66246,#66247,#66248,#66249,#66250,#66251,#66252,#66253,#66254,
#66255,#66256,#66257),.UNSPECIFIED.,.F.,.F.,(4,3,3,3,3,3,3,3,3,3,3,3,3,
3,3,3,3,3,3,3,3,3,3,3,3,3,3,3,3,3,3,3,3,3,3,3,3,3,3,4),(-2.18372485524376,
-2.1080836132479,-2.10067445865023,-2.02554364211438,-1.97122025763592,
-1.94231974546435,-1.92754171670523,-1.91459124648127,-1.83886496105845,
-1.76258470621486,-1.6865379800221,-1.65856899219342,-1.65041313088924,
-1.59095656628675,-1.51509963942128,-1.43840807790671,-1.36135050703557,
-1.28855588873818,-1.26125790687666,-1.25248255692291,-1.24392346223787,
-1.16637145545167,-1.08842971125478,-1.07017203384601,-0.99260224660891,
-0.914715510270571,-0.867783080022901,-0.844451783430773,-0.834689007924211,
-0.756387874815429,-0.677626836552787,-0.599000922678516,-0.539256068289211,
-0.46377131939894,-0.435464538565089,-0.425029568743666,-0.416657160262855,
-0.338503489008845,-0.259212771020976,-0.23731707272813),.UNSPECIFIED.);
#9664=B_SPLINE_CURVE_WITH_KNOTS('',3,(#66258,#66259,#66260,#66261,#66262,
#66263,#66264,#66265,#66266,#66267,#66268,#66269,#66270,#66271),
 .UNSPECIFIED.,.F.,.F.,(4,1,1,1,1,1,1,1,1,1,1,4),(10.3764180272043,10.7919972319373,
11.2896466029306,11.7872959739239,12.2849453449171,12.7825947159104,13.2802440869037,
13.777893457897,14.2755428288902,14.7731921998835,15.2708415708768,15.707963267949),
 .UNSPECIFIED.);
#9665=B_SPLINE_CURVE_WITH_KNOTS('',3,(#66272,#66273,#66274,#66275),
 .UNSPECIFIED.,.F.,.F.,(4,4),(177.048907408549,177.081105907345),
 .UNSPECIFIED.);
#9666=B_SPLINE_CURVE_WITH_KNOTS('',3,(#66312,#66313,#66314,#66315),
 .UNSPECIFIED.,.F.,.F.,(4,4),(2.38752198326049,2.59689972411661),
 .UNSPECIFIED.);
#9667=B_SPLINE_CURVE_WITH_KNOTS('',3,(#66317,#66318,#66319,#66320,#66321,
#66322,#66323,#66324,#66325,#66326),.UNSPECIFIED.,.F.,.F.,(4,2,2,2,4),(-0.89334799527249,
-0.744300931247914,-0.364358329298144,0.,0.0053107731540207),
 .UNSPECIFIED.);
#9668=B_SPLINE_CURVE_WITH_KNOTS('',3,(#66328,#66329,#66330,#66331,#66332,
#66333,#66334,#66335),.UNSPECIFIED.,.F.,.F.,(4,2,2,4),(0.361811982156075,
0.592933792628361,0.87034240784702,1.12767208658309),.UNSPECIFIED.);
#9669=B_SPLINE_CURVE_WITH_KNOTS('',3,(#66336,#66337,#66338,#66339),
 .UNSPECIFIED.,.F.,.F.,(4,4),(0.,0.247638878335359),.UNSPECIFIED.);
#9670=B_SPLINE_CURVE_WITH_KNOTS('',3,(#66342,#66343,#66344,#66345,#66346,
#66347,#66348,#66349,#66350,#66351,#66352,#66353,#66354,#66355,#66356,#66357,
#66358,#66359,#66360,#66361,#66362,#66363,#66364,#66365,#66366,#66367,#66368,
#66369,#66370,#66371,#66372,#66373,#66374,#66375,#66376,#66377,#66378,#66379,
#66380,#66381,#66382,#66383,#66384,#66385,#66386,#66387,#66388,#66389,#66390,
#66391,#66392,#66393,#66394,#66395,#66396,#66397,#66398,#66399),
 .UNSPECIFIED.,.F.,.F.,(4,3,3,3,3,3,3,3,3,3,3,3,3,3,3,3,3,3,3,4),(10.4929728200354,
10.5444708718562,10.5613571367491,10.5734229444277,10.6504408601189,10.7283038540831,
10.8061128647024,10.8831396541727,10.9049572346023,10.9709195580298,10.983448388147,
11.0603712677518,11.1381797388444,11.2163620372511,11.2941737976529,11.3634148098376,
11.3824774676397,11.3906958616324,11.4326558220224,11.4638916704572),
 .UNSPECIFIED.);
#9671=B_SPLINE_CURVE_WITH_KNOTS('',3,(#66416,#66417,#66418,#66419,#66420,
#66421,#66422,#66423,#66424,#66425,#66426,#66427,#66428,#66429,#66430,#66431,
#66432,#66433,#66434,#66435,#66436,#66437,#66438,#66439,#66440,#66441,#66442,
#66443,#66444,#66445,#66446,#66447,#66448,#66449,#66450,#66451,#66452,#66453,
#66454,#66455,#66456,#66457,#66458,#66459,#66460,#66461,#66462,#66463,#66464,
#66465,#66466,#66467,#66468,#66469,#66470,#66471,#66472,#66473,#66474,#66475,
#66476),.UNSPECIFIED.,.F.,.F.,(4,3,3,3,3,3,3,3,3,3,3,3,3,3,3,3,3,3,3,3,
4),(-1.66480832705423,-1.63227747630844,-1.55243434084099,-1.47556156715774,
-1.39780685101578,-1.32009524930909,-1.24316869333914,-1.21961413936388,
-1.14239372456762,-1.06514562100159,-1.03036760933897,-0.953055464575741,
-0.875884864276646,-0.809706214516272,-0.732914922349529,-0.65592218719066,
-0.579508457494233,-0.512582701340628,-0.435709040867744,-0.402987998031786,
-0.377742144895607),.UNSPECIFIED.);
#9672=B_SPLINE_CURVE_WITH_KNOTS('',3,(#66493,#66494,#66495,#66496,#66497,
#66498),.UNSPECIFIED.,.F.,.F.,(4,1,1,4),(10.5690204901905,10.7239933461083,
11.2227279776405,11.6147305479244),.UNSPECIFIED.);
#9673=B_SPLINE_CURVE_WITH_KNOTS('',3,(#66499,#66500,#66501,#66502,#66503,
#66504,#66505,#66506,#66507,#66508,#66509,#66510),.UNSPECIFIED.,.F.,.F.,
(4,1,1,1,1,1,1,1,1,4),(11.6147305479244,11.7214626091727,12.2201972407048,
12.718931872237,13.2176665037692,13.7164011353014,14.2151357668335,14.7138703983657,
15.2126050298979,15.707963267949),.UNSPECIFIED.);
#10358=LINE('',#57287,#12852);
#10359=LINE('',#57297,#12853);
#10360=LINE('',#57383,#12854);
#10361=LINE('',#57473,#12855);
#10362=LINE('',#57560,#12856);
#10363=LINE('',#57647,#12857);
#10364=LINE('',#57734,#12858);
#10365=LINE('',#57824,#12859);
#10366=LINE('',#57911,#12860);
#10367=LINE('',#57998,#12861);
#10368=LINE('',#58085,#12862);
#10369=LINE('',#58172,#12863);
#10370=LINE('',#58262,#12864);
#10371=LINE('',#58349,#12865);
#10372=LINE('',#58436,#12866);
#10373=LINE('',#58526,#12867);
#10374=LINE('',#58610,#12868);
#10375=LINE('',#58700,#12869);
#10376=LINE('',#58787,#12870);
#10377=LINE('',#58874,#12871);
#10378=LINE('',#58964,#12872);
#10379=LINE('',#59048,#12873);
#10380=LINE('',#59138,#12874);
#10381=LINE('',#59228,#12875);
#10382=LINE('',#59312,#12876);
#10383=LINE('',#59402,#12877);
#10384=LINE('',#59486,#12878);
#10385=LINE('',#59576,#12879);
#10386=LINE('',#59666,#12880);
#10387=LINE('',#59746,#12881);
#10388=LINE('',#59771,#12882);
#10389=LINE('',#59808,#12883);
#10390=LINE('',#59846,#12884);
#10391=LINE('',#59883,#12885);
#10392=LINE('',#59920,#12886);
#10393=LINE('',#59957,#12887);
#10394=LINE('',#59994,#12888);
#10395=LINE('',#60032,#12889);
#10396=LINE('',#60069,#12890);
#10397=LINE('',#60106,#12891);
#10398=LINE('',#60143,#12892);
#10399=LINE('',#60181,#12893);
#10400=LINE('',#60218,#12894);
#10401=LINE('',#60255,#12895);
#10402=LINE('',#60292,#12896);
#10403=LINE('',#60329,#12897);
#10404=LINE('',#60367,#12898);
#10405=LINE('',#60404,#12899);
#10406=LINE('',#60441,#12900);
#10407=LINE('',#60479,#12901);
#10408=LINE('',#60515,#12902);
#10409=LINE('',#60553,#12903);
#10410=LINE('',#60590,#12904);
#10411=LINE('',#60627,#12905);
#10412=LINE('',#60665,#12906);
#10413=LINE('',#60701,#12907);
#10414=LINE('',#60739,#12908);
#10415=LINE('',#61248,#12909);
#10416=LINE('',#61610,#12910);
#10417=LINE('',#61615,#12911);
#10418=LINE('',#61635,#12912);
#10419=LINE('',#61647,#12913);
#10420=LINE('',#61651,#12914);
#10421=LINE('',#61655,#12915);
#10422=LINE('',#61659,#12916);
#10423=LINE('',#61663,#12917);
#10424=LINE('',#61667,#12918);
#10425=LINE('',#61671,#12919);
#10426=LINE('',#61675,#12920);
#10427=LINE('',#61679,#12921);
#10428=LINE('',#61683,#12922);
#10429=LINE('',#61687,#12923);
#10430=LINE('',#61691,#12924);
#10431=LINE('',#61695,#12925);
#10432=LINE('',#61699,#12926);
#10433=LINE('',#61703,#12927);
#10434=LINE('',#61707,#12928);
#10435=LINE('',#61711,#12929);
#10436=LINE('',#61715,#12930);
#10437=LINE('',#61719,#12931);
#10438=LINE('',#61723,#12932);
#10439=LINE('',#61727,#12933);
#10440=LINE('',#61731,#12934);
#10441=LINE('',#61735,#12935);
#10442=LINE('',#61739,#12936);
#10443=LINE('',#61743,#12937);
#10444=LINE('',#61747,#12938);
#10445=LINE('',#61751,#12939);
#10446=LINE('',#61754,#12940);
#10447=LINE('',#63894,#12941);
#10448=LINE('',#63980,#12942);
#10449=LINE('',#63983,#12943);
#10450=LINE('',#63986,#12944);
#10451=LINE('',#63990,#12945);
#10452=LINE('',#63994,#12946);
#10453=LINE('',#63998,#12947);
#10454=LINE('',#64002,#12948);
#10455=LINE('',#64006,#12949);
#10456=LINE('',#64010,#12950);
#10457=LINE('',#64014,#12951);
#10458=LINE('',#64018,#12952);
#10459=LINE('',#64022,#12953);
#10460=LINE('',#64026,#12954);
#10461=LINE('',#64030,#12955);
#10462=LINE('',#64034,#12956);
#10463=LINE('',#64038,#12957);
#10464=LINE('',#64042,#12958);
#10465=LINE('',#64046,#12959);
#10466=LINE('',#64050,#12960);
#10467=LINE('',#64054,#12961);
#10468=LINE('',#64058,#12962);
#10469=LINE('',#64062,#12963);
#10470=LINE('',#64066,#12964);
#10471=LINE('',#64070,#12965);
#10472=LINE('',#64074,#12966);
#10473=LINE('',#64078,#12967);
#10474=LINE('',#64082,#12968);
#10475=LINE('',#64086,#12969);
#10476=LINE('',#64089,#12970);
#10477=LINE('',#64347,#12971);
#10478=LINE('',#64348,#12972);
#10479=LINE('',#64350,#12973);
#10480=LINE('',#64351,#12974);
#10481=LINE('',#64353,#12975);
#10482=LINE('',#64354,#12976);
#10483=LINE('',#64356,#12977);
#10484=LINE('',#64357,#12978);
#10485=LINE('',#64359,#12979);
#10486=LINE('',#64360,#12980);
#10487=LINE('',#64362,#12981);
#10488=LINE('',#64363,#12982);
#10489=LINE('',#64365,#12983);
#10490=LINE('',#64366,#12984);
#10491=LINE('',#64368,#12985);
#10492=LINE('',#64369,#12986);
#10493=LINE('',#64371,#12987);
#10494=LINE('',#64372,#12988);
#10495=LINE('',#64374,#12989);
#10496=LINE('',#64375,#12990);
#10497=LINE('',#64377,#12991);
#10498=LINE('',#64378,#12992);
#10499=LINE('',#64380,#12993);
#10500=LINE('',#64381,#12994);
#10501=LINE('',#64383,#12995);
#10502=LINE('',#64384,#12996);
#10503=LINE('',#64386,#12997);
#10504=LINE('',#64387,#12998);
#10505=LINE('',#64389,#12999);
#10506=LINE('',#64390,#13000);
#10507=LINE('',#64392,#13001);
#10508=LINE('',#64393,#13002);
#10509=LINE('',#64395,#13003);
#10510=LINE('',#64396,#13004);
#10511=LINE('',#64398,#13005);
#10512=LINE('',#64399,#13006);
#10513=LINE('',#64401,#13007);
#10514=LINE('',#64402,#13008);
#10515=LINE('',#64404,#13009);
#10516=LINE('',#64405,#13010);
#10517=LINE('',#64407,#13011);
#10518=LINE('',#64408,#13012);
#10519=LINE('',#64410,#13013);
#10520=LINE('',#64411,#13014);
#10521=LINE('',#66404,#13015);
#10522=LINE('',#66405,#13016);
#10523=LINE('',#66407,#13017);
#10524=LINE('',#66408,#13018);
#10525=LINE('',#66410,#13019);
#10526=LINE('',#66411,#13020);
#10527=LINE('',#66481,#13021);
#10528=LINE('',#66482,#13022);
#10529=LINE('',#66489,#13023);
#10530=LINE('',#67981,#13024);
#12852=VECTOR('',#45302,11.);
#12853=VECTOR('',#45307,11.);
#12854=VECTOR('',#45312,11.);
#12855=VECTOR('',#45315,11.);
#12856=VECTOR('',#45318,11.);
#12857=VECTOR('',#45321,11.);
#12858=VECTOR('',#45324,11.);
#12859=VECTOR('',#45327,11.);
#12860=VECTOR('',#45330,11.);
#12861=VECTOR('',#45333,11.);
#12862=VECTOR('',#45336,11.);
#12863=VECTOR('',#45339,11.);
#12864=VECTOR('',#45342,11.);
#12865=VECTOR('',#45345,11.);
#12866=VECTOR('',#45348,11.);
#12867=VECTOR('',#45351,11.);
#12868=VECTOR('',#45354,11.);
#12869=VECTOR('',#45357,11.);
#12870=VECTOR('',#45360,11.);
#12871=VECTOR('',#45363,11.);
#12872=VECTOR('',#45366,11.);
#12873=VECTOR('',#45369,11.);
#12874=VECTOR('',#45372,11.);
#12875=VECTOR('',#45375,11.);
#12876=VECTOR('',#45378,11.);
#12877=VECTOR('',#45381,11.);
#12878=VECTOR('',#45384,11.);
#12879=VECTOR('',#45387,11.);
#12880=VECTOR('',#45390,11.);
#12881=VECTOR('',#45395,10.0685);
#12882=VECTOR('',#45400,10.0685);
#12883=VECTOR('',#45403,10.0685);
#12884=VECTOR('',#45406,10.0685);
#12885=VECTOR('',#45409,10.0685);
#12886=VECTOR('',#45412,10.0685);
#12887=VECTOR('',#45415,10.0685);
#12888=VECTOR('',#45418,10.0685);
#12889=VECTOR('',#45421,10.0685);
#12890=VECTOR('',#45424,10.0685);
#12891=VECTOR('',#45427,10.0685);
#12892=VECTOR('',#45430,10.0685);
#12893=VECTOR('',#45433,10.0685);
#12894=VECTOR('',#45436,10.0685);
#12895=VECTOR('',#45439,10.0685);
#12896=VECTOR('',#45442,10.0685);
#12897=VECTOR('',#45445,10.0685);
#12898=VECTOR('',#45448,10.0685);
#12899=VECTOR('',#45451,10.0685);
#12900=VECTOR('',#45454,10.0685);
#12901=VECTOR('',#45457,10.0685);
#12902=VECTOR('',#45460,10.0685);
#12903=VECTOR('',#45463,10.0685);
#12904=VECTOR('',#45466,10.0685);
#12905=VECTOR('',#45469,10.0685);
#12906=VECTOR('',#45472,10.0685);
#12907=VECTOR('',#45475,10.0685);
#12908=VECTOR('',#45478,10.0685);
#12909=VECTOR('',#45489,45.25);
#12910=VECTOR('',#45510,29.5);
#12911=VECTOR('',#45517,33.);
#12912=VECTOR('',#45544,17.);
#12913=VECTOR('',#45557,10.);
#12914=VECTOR('',#45560,10.);
#12915=VECTOR('',#45563,10.);
#12916=VECTOR('',#45566,10.);
#12917=VECTOR('',#45569,10.);
#12918=VECTOR('',#45572,10.);
#12919=VECTOR('',#45575,10.);
#12920=VECTOR('',#45578,10.);
#12921=VECTOR('',#45581,10.);
#12922=VECTOR('',#45584,10.);
#12923=VECTOR('',#45587,10.);
#12924=VECTOR('',#45590,10.);
#12925=VECTOR('',#45593,10.);
#12926=VECTOR('',#45596,10.);
#12927=VECTOR('',#45599,10.);
#12928=VECTOR('',#45602,10.);
#12929=VECTOR('',#45605,10.);
#12930=VECTOR('',#45608,10.);
#12931=VECTOR('',#45611,10.);
#12932=VECTOR('',#45614,10.);
#12933=VECTOR('',#45617,10.);
#12934=VECTOR('',#45620,10.);
#12935=VECTOR('',#45623,10.);
#12936=VECTOR('',#45626,10.);
#12937=VECTOR('',#45629,10.);
#12938=VECTOR('',#45632,10.);
#12939=VECTOR('',#45635,10.);
#12940=VECTOR('',#45640,14.);
#12941=VECTOR('',#45879,40.);
#12942=VECTOR('',#45882,10.);
#12943=VECTOR('',#45885,10.);
#12944=VECTOR('',#45888,10.);
#12945=VECTOR('',#45891,10.);
#12946=VECTOR('',#45894,10.);
#12947=VECTOR('',#45897,10.);
#12948=VECTOR('',#45900,10.);
#12949=VECTOR('',#45903,10.);
#12950=VECTOR('',#45906,10.);
#12951=VECTOR('',#45909,10.);
#12952=VECTOR('',#45912,10.);
#12953=VECTOR('',#45915,10.);
#12954=VECTOR('',#45918,10.);
#12955=VECTOR('',#45921,10.);
#12956=VECTOR('',#45924,10.);
#12957=VECTOR('',#45927,10.);
#12958=VECTOR('',#45930,10.);
#12959=VECTOR('',#45933,10.);
#12960=VECTOR('',#45936,10.);
#12961=VECTOR('',#45939,10.);
#12962=VECTOR('',#45942,10.);
#12963=VECTOR('',#45945,10.);
#12964=VECTOR('',#45948,10.);
#12965=VECTOR('',#45951,10.);
#12966=VECTOR('',#45954,10.);
#12967=VECTOR('',#45957,10.);
#12968=VECTOR('',#45960,10.);
#12969=VECTOR('',#45963,10.);
#12970=VECTOR('',#45966,10.);
#12971=VECTOR('',#45971,10.);
#12972=VECTOR('',#45972,10.);
#12973=VECTOR('',#45975,10.);
#12974=VECTOR('',#45976,10.);
#12975=VECTOR('',#45979,10.);
#12976=VECTOR('',#45980,10.);
#12977=VECTOR('',#45983,10.);
#12978=VECTOR('',#45984,10.);
#12979=VECTOR('',#45987,10.);
#12980=VECTOR('',#45988,10.);
#12981=VECTOR('',#45991,10.);
#12982=VECTOR('',#45992,10.);
#12983=VECTOR('',#45995,10.);
#12984=VECTOR('',#45996,10.);
#12985=VECTOR('',#45999,10.);
#12986=VECTOR('',#46000,10.);
#12987=VECTOR('',#46003,10.);
#12988=VECTOR('',#46004,10.);
#12989=VECTOR('',#46007,10.);
#12990=VECTOR('',#46008,10.);
#12991=VECTOR('',#46011,10.);
#12992=VECTOR('',#46012,10.);
#12993=VECTOR('',#46015,10.);
#12994=VECTOR('',#46016,10.);
#12995=VECTOR('',#46019,10.);
#12996=VECTOR('',#46020,10.);
#12997=VECTOR('',#46023,10.);
#12998=VECTOR('',#46024,10.);
#12999=VECTOR('',#46027,10.);
#13000=VECTOR('',#46028,10.);
#13001=VECTOR('',#46031,10.);
#13002=VECTOR('',#46032,10.);
#13003=VECTOR('',#46035,10.);
#13004=VECTOR('',#46036,10.);
#13005=VECTOR('',#46039,10.);
#13006=VECTOR('',#46040,10.);
#13007=VECTOR('',#46043,10.);
#13008=VECTOR('',#46044,10.);
#13009=VECTOR('',#46047,10.);
#13010=VECTOR('',#46048,10.);
#13011=VECTOR('',#46051,10.);
#13012=VECTOR('',#46052,10.);
#13013=VECTOR('',#46055,10.);
#13014=VECTOR('',#46056,10.);
#13015=VECTOR('',#46069,10.);
#13016=VECTOR('',#46070,10.);
#13017=VECTOR('',#46073,10.);
#13018=VECTOR('',#46074,10.);
#13019=VECTOR('',#46077,10.);
#13020=VECTOR('',#46078,10.);
#13021=VECTOR('',#46091,10.);
#13022=VECTOR('',#46092,10.);
#13023=VECTOR('',#46101,2.5);
#13024=VECTOR('',#46108,2.5);
#15346=VERTEX_POINT('',#57285);
#15347=VERTEX_POINT('',#57286);
#15348=VERTEX_POINT('',#57288);
#15349=VERTEX_POINT('',#57295);
#15350=VERTEX_POINT('',#57296);
#15351=VERTEX_POINT('',#57341);
#15352=VERTEX_POINT('',#57381);
#15353=VERTEX_POINT('',#57382);
#15354=VERTEX_POINT('',#57471);
#15355=VERTEX_POINT('',#57472);
#15356=VERTEX_POINT('',#57558);
#15357=VERTEX_POINT('',#57559);
#15358=VERTEX_POINT('',#57645);
#15359=VERTEX_POINT('',#57646);
#15360=VERTEX_POINT('',#57732);
#15361=VERTEX_POINT('',#57733);
#15362=VERTEX_POINT('',#57822);
#15363=VERTEX_POINT('',#57823);
#15364=VERTEX_POINT('',#57909);
#15365=VERTEX_POINT('',#57910);
#15366=VERTEX_POINT('',#57996);
#15367=VERTEX_POINT('',#57997);
#15368=VERTEX_POINT('',#58083);
#15369=VERTEX_POINT('',#58084);
#15370=VERTEX_POINT('',#58170);
#15371=VERTEX_POINT('',#58171);
#15372=VERTEX_POINT('',#58260);
#15373=VERTEX_POINT('',#58261);
#15374=VERTEX_POINT('',#58347);
#15375=VERTEX_POINT('',#58348);
#15376=VERTEX_POINT('',#58434);
#15377=VERTEX_POINT('',#58435);
#15378=VERTEX_POINT('',#58524);
#15379=VERTEX_POINT('',#58525);
#15380=VERTEX_POINT('',#58608);
#15381=VERTEX_POINT('',#58609);
#15382=VERTEX_POINT('',#58698);
#15383=VERTEX_POINT('',#58699);
#15384=VERTEX_POINT('',#58785);
#15385=VERTEX_POINT('',#58786);
#15386=VERTEX_POINT('',#58872);
#15387=VERTEX_POINT('',#58873);
#15388=VERTEX_POINT('',#58962);
#15389=VERTEX_POINT('',#58963);
#15390=VERTEX_POINT('',#59046);
#15391=VERTEX_POINT('',#59047);
#15392=VERTEX_POINT('',#59136);
#15393=VERTEX_POINT('',#59137);
#15394=VERTEX_POINT('',#59226);
#15395=VERTEX_POINT('',#59227);
#15396=VERTEX_POINT('',#59310);
#15397=VERTEX_POINT('',#59311);
#15398=VERTEX_POINT('',#59400);
#15399=VERTEX_POINT('',#59401);
#15400=VERTEX_POINT('',#59484);
#15401=VERTEX_POINT('',#59485);
#15402=VERTEX_POINT('',#59574);
#15403=VERTEX_POINT('',#59575);
#15404=VERTEX_POINT('',#59664);
#15405=VERTEX_POINT('',#59665);
#15406=VERTEX_POINT('',#59667);
#15407=VERTEX_POINT('',#59744);
#15408=VERTEX_POINT('',#59745);
#15409=VERTEX_POINT('',#59747);
#15410=VERTEX_POINT('',#59758);
#15411=VERTEX_POINT('',#59769);
#15412=VERTEX_POINT('',#59770);
#15413=VERTEX_POINT('',#59806);
#15414=VERTEX_POINT('',#59807);
#15415=VERTEX_POINT('',#59844);
#15416=VERTEX_POINT('',#59845);
#15417=VERTEX_POINT('',#59881);
#15418=VERTEX_POINT('',#59882);
#15419=VERTEX_POINT('',#59918);
#15420=VERTEX_POINT('',#59919);
#15421=VERTEX_POINT('',#59955);
#15422=VERTEX_POINT('',#59956);
#15423=VERTEX_POINT('',#59992);
#15424=VERTEX_POINT('',#59993);
#15425=VERTEX_POINT('',#60030);
#15426=VERTEX_POINT('',#60031);
#15427=VERTEX_POINT('',#60067);
#15428=VERTEX_POINT('',#60068);
#15429=VERTEX_POINT('',#60104);
#15430=VERTEX_POINT('',#60105);
#15431=VERTEX_POINT('',#60141);
#15432=VERTEX_POINT('',#60142);
#15433=VERTEX_POINT('',#60179);
#15434=VERTEX_POINT('',#60180);
#15435=VERTEX_POINT('',#60216);
#15436=VERTEX_POINT('',#60217);
#15437=VERTEX_POINT('',#60253);
#15438=VERTEX_POINT('',#60254);
#15439=VERTEX_POINT('',#60290);
#15440=VERTEX_POINT('',#60291);
#15441=VERTEX_POINT('',#60327);
#15442=VERTEX_POINT('',#60328);
#15443=VERTEX_POINT('',#60365);
#15444=VERTEX_POINT('',#60366);
#15445=VERTEX_POINT('',#60402);
#15446=VERTEX_POINT('',#60403);
#15447=VERTEX_POINT('',#60439);
#15448=VERTEX_POINT('',#60440);
#15449=VERTEX_POINT('',#60477);
#15450=VERTEX_POINT('',#60478);
#15451=VERTEX_POINT('',#60513);
#15452=VERTEX_POINT('',#60514);
#15453=VERTEX_POINT('',#60551);
#15454=VERTEX_POINT('',#60552);
#15455=VERTEX_POINT('',#60588);
#15456=VERTEX_POINT('',#60589);
#15457=VERTEX_POINT('',#60625);
#15458=VERTEX_POINT('',#60626);
#15459=VERTEX_POINT('',#60663);
#15460=VERTEX_POINT('',#60664);
#15461=VERTEX_POINT('',#60699);
#15462=VERTEX_POINT('',#60700);
#15463=VERTEX_POINT('',#60737);
#15464=VERTEX_POINT('',#60738);
#15465=VERTEX_POINT('',#60862);
#15466=VERTEX_POINT('',#60863);
#15467=VERTEX_POINT('',#61044);
#15468=VERTEX_POINT('',#61122);
#15469=VERTEX_POINT('',#61216);
#15470=VERTEX_POINT('',#61218);
#15471=VERTEX_POINT('',#61247);
#15472=VERTEX_POINT('',#61249);
#15473=VERTEX_POINT('',#61369);
#15474=VERTEX_POINT('',#61574);
#15475=VERTEX_POINT('',#61595);
#15476=VERTEX_POINT('',#61599);
#15477=VERTEX_POINT('',#61600);
#15478=VERTEX_POINT('',#61603);
#15479=VERTEX_POINT('',#61605);
#15480=VERTEX_POINT('',#61609);
#15481=VERTEX_POINT('',#61611);
#15482=VERTEX_POINT('',#61617);
#15483=VERTEX_POINT('',#61621);
#15484=VERTEX_POINT('',#61624);
#15485=VERTEX_POINT('',#61625);
#15486=VERTEX_POINT('',#61628);
#15487=VERTEX_POINT('',#61632);
#15488=VERTEX_POINT('',#61637);
#15489=VERTEX_POINT('',#61638);
#15490=VERTEX_POINT('',#61641);
#15491=VERTEX_POINT('',#61645);
#15492=VERTEX_POINT('',#61646);
#15493=VERTEX_POINT('',#61648);
#15494=VERTEX_POINT('',#61650);
#15495=VERTEX_POINT('',#61652);
#15496=VERTEX_POINT('',#61654);
#15497=VERTEX_POINT('',#61656);
#15498=VERTEX_POINT('',#61658);
#15499=VERTEX_POINT('',#61660);
#15500=VERTEX_POINT('',#61662);
#15501=VERTEX_POINT('',#61664);
#15502=VERTEX_POINT('',#61666);
#15503=VERTEX_POINT('',#61668);
#15504=VERTEX_POINT('',#61670);
#15505=VERTEX_POINT('',#61672);
#15506=VERTEX_POINT('',#61674);
#15507=VERTEX_POINT('',#61676);
#15508=VERTEX_POINT('',#61678);
#15509=VERTEX_POINT('',#61680);
#15510=VERTEX_POINT('',#61682);
#15511=VERTEX_POINT('',#61684);
#15512=VERTEX_POINT('',#61686);
#15513=VERTEX_POINT('',#61688);
#15514=VERTEX_POINT('',#61690);
#15515=VERTEX_POINT('',#61692);
#15516=VERTEX_POINT('',#61694);
#15517=VERTEX_POINT('',#61696);
#15518=VERTEX_POINT('',#61698);
#15519=VERTEX_POINT('',#61700);
#15520=VERTEX_POINT('',#61702);
#15521=VERTEX_POINT('',#61704);
#15522=VERTEX_POINT('',#61706);
#15523=VERTEX_POINT('',#61708);
#15524=VERTEX_POINT('',#61710);
#15525=VERTEX_POINT('',#61712);
#15526=VERTEX_POINT('',#61714);
#15527=VERTEX_POINT('',#61716);
#15528=VERTEX_POINT('',#61718);
#15529=VERTEX_POINT('',#61720);
#15530=VERTEX_POINT('',#61722);
#15531=VERTEX_POINT('',#61724);
#15532=VERTEX_POINT('',#61726);
#15533=VERTEX_POINT('',#61728);
#15534=VERTEX_POINT('',#61730);
#15535=VERTEX_POINT('',#61732);
#15536=VERTEX_POINT('',#61734);
#15537=VERTEX_POINT('',#61736);
#15538=VERTEX_POINT('',#61738);
#15539=VERTEX_POINT('',#61740);
#15540=VERTEX_POINT('',#61742);
#15541=VERTEX_POINT('',#61744);
#15542=VERTEX_POINT('',#61746);
#15543=VERTEX_POINT('',#61748);
#15544=VERTEX_POINT('',#61750);
#15545=VERTEX_POINT('',#61775);
#15546=VERTEX_POINT('',#61776);
#15547=VERTEX_POINT('',#61783);
#15548=VERTEX_POINT('',#61788);
#15549=VERTEX_POINT('',#61795);
#15550=VERTEX_POINT('',#61804);
#15551=VERTEX_POINT('',#61841);
#15552=VERTEX_POINT('',#61842);
#15553=VERTEX_POINT('',#61847);
#15554=VERTEX_POINT('',#61854);
#15555=VERTEX_POINT('',#61863);
#15556=VERTEX_POINT('',#61868);
#15557=VERTEX_POINT('',#61905);
#15558=VERTEX_POINT('',#61906);
#15559=VERTEX_POINT('',#61912);
#15560=VERTEX_POINT('',#61947);
#15561=VERTEX_POINT('',#61954);
#15562=VERTEX_POINT('',#61963);
#15563=VERTEX_POINT('',#61968);
#15564=VERTEX_POINT('',#61973);
#15565=VERTEX_POINT('',#61979);
#15566=VERTEX_POINT('',#61994);
#15567=VERTEX_POINT('',#61995);
#15568=VERTEX_POINT('',#61997);
#15569=VERTEX_POINT('',#61999);
#15570=VERTEX_POINT('',#62003);
#15571=VERTEX_POINT('',#62007);
#15572=VERTEX_POINT('',#62052);
#15573=VERTEX_POINT('',#62060);
#15574=VERTEX_POINT('',#62159);
#15575=VERTEX_POINT('',#62166);
#15576=VERTEX_POINT('',#62175);
#15577=VERTEX_POINT('',#62202);
#15578=VERTEX_POINT('',#62204);
#15579=VERTEX_POINT('',#62210);
#15580=VERTEX_POINT('',#62233);
#15581=VERTEX_POINT('',#62244);
#15582=VERTEX_POINT('',#62247);
#15583=VERTEX_POINT('',#62276);
#15584=VERTEX_POINT('',#62277);
#15585=VERTEX_POINT('',#62280);
#15586=VERTEX_POINT('',#62282);
#15587=VERTEX_POINT('',#62288);
#15588=VERTEX_POINT('',#62293);
#15589=VERTEX_POINT('',#62298);
#15590=VERTEX_POINT('',#62304);
#15591=VERTEX_POINT('',#62306);
#15592=VERTEX_POINT('',#62316);
#15593=VERTEX_POINT('',#62321);
#15594=VERTEX_POINT('',#62327);
#15595=VERTEX_POINT('',#62329);
#15596=VERTEX_POINT('',#62335);
#15597=VERTEX_POINT('',#62340);
#15598=VERTEX_POINT('',#62345);
#15599=VERTEX_POINT('',#62351);
#15600=VERTEX_POINT('',#62353);
#15601=VERTEX_POINT('',#62359);
#15602=VERTEX_POINT('',#62364);
#15603=VERTEX_POINT('',#62374);
#15604=VERTEX_POINT('',#62380);
#15605=VERTEX_POINT('',#62385);
#15606=VERTEX_POINT('',#62412);
#15607=VERTEX_POINT('',#62419);
#15608=VERTEX_POINT('',#62430);
#15609=VERTEX_POINT('',#62435);
#15610=VERTEX_POINT('',#62494);
#15611=VERTEX_POINT('',#62568);
#15612=VERTEX_POINT('',#62597);
#15613=VERTEX_POINT('',#62624);
#15614=VERTEX_POINT('',#62654);
#15615=VERTEX_POINT('',#62655);
#15616=VERTEX_POINT('',#62691);
#15617=VERTEX_POINT('',#62693);
#15618=VERTEX_POINT('',#62702);
#15619=VERTEX_POINT('',#62709);
#15620=VERTEX_POINT('',#62711);
#15621=VERTEX_POINT('',#62713);
#15622=VERTEX_POINT('',#62799);
#15623=VERTEX_POINT('',#62801);
#15624=VERTEX_POINT('',#62881);
#15625=VERTEX_POINT('',#62883);
#15626=VERTEX_POINT('',#63077);
#15627=VERTEX_POINT('',#63084);
#15628=VERTEX_POINT('',#63093);
#15629=VERTEX_POINT('',#63098);
#15630=VERTEX_POINT('',#63135);
#15631=VERTEX_POINT('',#63146);
#15632=VERTEX_POINT('',#63150);
#15633=VERTEX_POINT('',#63177);
#15634=VERTEX_POINT('',#63211);
#15635=VERTEX_POINT('',#63245);
#15636=VERTEX_POINT('',#63253);
#15637=VERTEX_POINT('',#63281);
#15638=VERTEX_POINT('',#63339);
#15639=VERTEX_POINT('',#63368);
#15640=VERTEX_POINT('',#63369);
#15641=VERTEX_POINT('',#63371);
#15642=VERTEX_POINT('',#63378);
#15643=VERTEX_POINT('',#63388);
#15644=VERTEX_POINT('',#63410);
#15645=VERTEX_POINT('',#63421);
#15646=VERTEX_POINT('',#63429);
#15647=VERTEX_POINT('',#63430);
#15648=VERTEX_POINT('',#63454);
#15649=VERTEX_POINT('',#63486);
#15650=VERTEX_POINT('',#63547);
#15651=VERTEX_POINT('',#63570);
#15652=VERTEX_POINT('',#63577);
#15653=VERTEX_POINT('',#63586);
#15654=VERTEX_POINT('',#63591);
#15655=VERTEX_POINT('',#63628);
#15656=VERTEX_POINT('',#63629);
#15657=VERTEX_POINT('',#63664);
#15658=VERTEX_POINT('',#63682);
#15659=VERTEX_POINT('',#63687);
#15660=VERTEX_POINT('',#63693);
#15661=VERTEX_POINT('',#63733);
#15662=VERTEX_POINT('',#63852);
#15663=VERTEX_POINT('',#63854);
#15664=VERTEX_POINT('',#63880);
#15665=VERTEX_POINT('',#63888);
#15666=VERTEX_POINT('',#63890);
#15667=VERTEX_POINT('',#63915);
#15668=VERTEX_POINT('',#63916);
#15669=VERTEX_POINT('',#63931);
#15670=VERTEX_POINT('',#63968);
#15671=VERTEX_POINT('',#63979);
#15672=VERTEX_POINT('',#63981);
#15673=VERTEX_POINT('',#63985);
#15674=VERTEX_POINT('',#63987);
#15675=VERTEX_POINT('',#63989);
#15676=VERTEX_POINT('',#63991);
#15677=VERTEX_POINT('',#63993);
#15678=VERTEX_POINT('',#63995);
#15679=VERTEX_POINT('',#63997);
#15680=VERTEX_POINT('',#63999);
#15681=VERTEX_POINT('',#64001);
#15682=VERTEX_POINT('',#64003);
#15683=VERTEX_POINT('',#64005);
#15684=VERTEX_POINT('',#64007);
#15685=VERTEX_POINT('',#64009);
#15686=VERTEX_POINT('',#64011);
#15687=VERTEX_POINT('',#64013);
#15688=VERTEX_POINT('',#64015);
#15689=VERTEX_POINT('',#64017);
#15690=VERTEX_POINT('',#64019);
#15691=VERTEX_POINT('',#64021);
#15692=VERTEX_POINT('',#64023);
#15693=VERTEX_POINT('',#64025);
#15694=VERTEX_POINT('',#64027);
#15695=VERTEX_POINT('',#64029);
#15696=VERTEX_POINT('',#64031);
#15697=VERTEX_POINT('',#64033);
#15698=VERTEX_POINT('',#64035);
#15699=VERTEX_POINT('',#64037);
#15700=VERTEX_POINT('',#64039);
#15701=VERTEX_POINT('',#64041);
#15702=VERTEX_POINT('',#64043);
#15703=VERTEX_POINT('',#64045);
#15704=VERTEX_POINT('',#64047);
#15705=VERTEX_POINT('',#64049);
#15706=VERTEX_POINT('',#64051);
#15707=VERTEX_POINT('',#64053);
#15708=VERTEX_POINT('',#64055);
#15709=VERTEX_POINT('',#64057);
#15710=VERTEX_POINT('',#64059);
#15711=VERTEX_POINT('',#64061);
#15712=VERTEX_POINT('',#64063);
#15713=VERTEX_POINT('',#64065);
#15714=VERTEX_POINT('',#64067);
#15715=VERTEX_POINT('',#64069);
#15716=VERTEX_POINT('',#64071);
#15717=VERTEX_POINT('',#64073);
#15718=VERTEX_POINT('',#64075);
#15719=VERTEX_POINT('',#64077);
#15720=VERTEX_POINT('',#64079);
#15721=VERTEX_POINT('',#64081);
#15722=VERTEX_POINT('',#64083);
#15723=VERTEX_POINT('',#64085);
#15724=VERTEX_POINT('',#64087);
#15725=VERTEX_POINT('',#64090);
#15726=VERTEX_POINT('',#64413);
#15727=VERTEX_POINT('',#64493);
#15728=VERTEX_POINT('',#64669);
#15729=VERTEX_POINT('',#66139);
#15730=VERTEX_POINT('',#66311);
#15731=VERTEX_POINT('',#66316);
#15732=VERTEX_POINT('',#66327);
#15733=VERTEX_POINT('',#66341);
#15734=VERTEX_POINT('',#66400);
#15735=VERTEX_POINT('',#66413);
#15736=VERTEX_POINT('',#66478);
#15737=VERTEX_POINT('',#66484);
#15738=VERTEX_POINT('',#66488);
#15739=VERTEX_POINT('',#66492);
#15740=VERTEX_POINT('',#67980);
#19074=EDGE_CURVE('',#15346,#15347,#10358,.T.);
#19075=EDGE_CURVE('',#15346,#15348,#9424,.T.);
#19076=EDGE_CURVE('',#15347,#15348,#7015,.T.);
#19077=EDGE_CURVE('',#15349,#15350,#10359,.T.);
#19078=EDGE_CURVE('',#15349,#15346,#9425,.T.);
#19079=EDGE_CURVE('',#15351,#15347,#7016,.T.);
#19080=EDGE_CURVE('',#15351,#15350,#9426,.T.);
#19081=EDGE_CURVE('',#15352,#15353,#10360,.T.);
#19082=EDGE_CURVE('',#15352,#15349,#9427,.T.);
#19083=EDGE_CURVE('',#15350,#15353,#9428,.T.);
#19084=EDGE_CURVE('',#15354,#15355,#10361,.T.);
#19085=EDGE_CURVE('',#15354,#15352,#9429,.T.);
#19086=EDGE_CURVE('',#15353,#15355,#9430,.T.);
#19087=EDGE_CURVE('',#15356,#15357,#10362,.T.);
#19088=EDGE_CURVE('',#15356,#15354,#9431,.T.);
#19089=EDGE_CURVE('',#15355,#15357,#9432,.T.);
#19090=EDGE_CURVE('',#15358,#15359,#10363,.T.);
#19091=EDGE_CURVE('',#15358,#15356,#9433,.T.);
#19092=EDGE_CURVE('',#15357,#15359,#9434,.T.);
#19093=EDGE_CURVE('',#15360,#15361,#10364,.T.);
#19094=EDGE_CURVE('',#15360,#15358,#9435,.T.);
#19095=EDGE_CURVE('',#15359,#15361,#9436,.T.);
#19096=EDGE_CURVE('',#15362,#15363,#10365,.T.);
#19097=EDGE_CURVE('',#15362,#15360,#9437,.T.);
#19098=EDGE_CURVE('',#15361,#15363,#9438,.T.);
#19099=EDGE_CURVE('',#15364,#15365,#10366,.T.);
#19100=EDGE_CURVE('',#15364,#15362,#9439,.T.);
#19101=EDGE_CURVE('',#15363,#15365,#9440,.T.);
#19102=EDGE_CURVE('',#15366,#15367,#10367,.T.);
#19103=EDGE_CURVE('',#15366,#15364,#9441,.T.);
#19104=EDGE_CURVE('',#15365,#15367,#9442,.T.);
#19105=EDGE_CURVE('',#15368,#15369,#10368,.T.);
#19106=EDGE_CURVE('',#15368,#15366,#9443,.T.);
#19107=EDGE_CURVE('',#15367,#15369,#9444,.T.);
#19108=EDGE_CURVE('',#15370,#15371,#10369,.T.);
#19109=EDGE_CURVE('',#15370,#15368,#9445,.T.);
#19110=EDGE_CURVE('',#15369,#15371,#9446,.T.);
#19111=EDGE_CURVE('',#15372,#15373,#10370,.T.);
#19112=EDGE_CURVE('',#15372,#15370,#9447,.T.);
#19113=EDGE_CURVE('',#15371,#15373,#9448,.T.);
#19114=EDGE_CURVE('',#15374,#15375,#10371,.T.);
#19115=EDGE_CURVE('',#15374,#15372,#9449,.T.);
#19116=EDGE_CURVE('',#15373,#15375,#9450,.T.);
#19117=EDGE_CURVE('',#15376,#15377,#10372,.T.);
#19118=EDGE_CURVE('',#15376,#15374,#9451,.T.);
#19119=EDGE_CURVE('',#15375,#15377,#9452,.T.);
#19120=EDGE_CURVE('',#15378,#15379,#10373,.T.);
#19121=EDGE_CURVE('',#15378,#15376,#9453,.T.);
#19122=EDGE_CURVE('',#15377,#15379,#9454,.T.);
#19123=EDGE_CURVE('',#15380,#15381,#10374,.T.);
#19124=EDGE_CURVE('',#15380,#15378,#9455,.T.);
#19125=EDGE_CURVE('',#15379,#15381,#9456,.T.);
#19126=EDGE_CURVE('',#15382,#15383,#10375,.T.);
#19127=EDGE_CURVE('',#15382,#15380,#9457,.T.);
#19128=EDGE_CURVE('',#15381,#15383,#9458,.T.);
#19129=EDGE_CURVE('',#15384,#15385,#10376,.T.);
#19130=EDGE_CURVE('',#15384,#15382,#9459,.T.);
#19131=EDGE_CURVE('',#15383,#15385,#9460,.T.);
#19132=EDGE_CURVE('',#15386,#15387,#10377,.T.);
#19133=EDGE_CURVE('',#15386,#15384,#9461,.T.);
#19134=EDGE_CURVE('',#15385,#15387,#9462,.T.);
#19135=EDGE_CURVE('',#15388,#15389,#10378,.T.);
#19136=EDGE_CURVE('',#15388,#15386,#9463,.T.);
#19137=EDGE_CURVE('',#15387,#15389,#9464,.T.);
#19138=EDGE_CURVE('',#15390,#15391,#10379,.T.);
#19139=EDGE_CURVE('',#15390,#15388,#9465,.T.);
#19140=EDGE_CURVE('',#15389,#15391,#9466,.T.);
#19141=EDGE_CURVE('',#15392,#15393,#10380,.T.);
#19142=EDGE_CURVE('',#15392,#15390,#9467,.T.);
#19143=EDGE_CURVE('',#15391,#15393,#9468,.T.);
#19144=EDGE_CURVE('',#15394,#15395,#10381,.T.);
#19145=EDGE_CURVE('',#15394,#15392,#9469,.T.);
#19146=EDGE_CURVE('',#15393,#15395,#9470,.T.);
#19147=EDGE_CURVE('',#15396,#15397,#10382,.T.);
#19148=EDGE_CURVE('',#15396,#15394,#9471,.T.);
#19149=EDGE_CURVE('',#15395,#15397,#9472,.T.);
#19150=EDGE_CURVE('',#15398,#15399,#10383,.T.);
#19151=EDGE_CURVE('',#15398,#15396,#9473,.T.);
#19152=EDGE_CURVE('',#15397,#15399,#9474,.T.);
#19153=EDGE_CURVE('',#15400,#15401,#10384,.T.);
#19154=EDGE_CURVE('',#15400,#15398,#9475,.T.);
#19155=EDGE_CURVE('',#15399,#15401,#9476,.T.);
#19156=EDGE_CURVE('',#15402,#15403,#10385,.T.);
#19157=EDGE_CURVE('',#15402,#15400,#9477,.T.);
#19158=EDGE_CURVE('',#15401,#15403,#9478,.T.);
#19159=EDGE_CURVE('',#15404,#15405,#10386,.T.);
#19160=EDGE_CURVE('',#15406,#15404,#7017,.T.);
#19161=EDGE_CURVE('',#15406,#15402,#9479,.T.);
#19162=EDGE_CURVE('',#15403,#15405,#9480,.T.);
#19163=EDGE_CURVE('',#15407,#15408,#10387,.T.);
#19164=EDGE_CURVE('',#15407,#15409,#9481,.T.);
#19165=EDGE_CURVE('',#15410,#15409,#7018,.T.);
#19166=EDGE_CURVE('',#15408,#15410,#9482,.T.);
#19167=EDGE_CURVE('',#15411,#15412,#10388,.T.);
#19168=EDGE_CURVE('',#15411,#15407,#9483,.T.);
#19169=EDGE_CURVE('',#15412,#15408,#9484,.T.);
#19170=EDGE_CURVE('',#15413,#15414,#10389,.T.);
#19171=EDGE_CURVE('',#15413,#15411,#9485,.T.);
#19172=EDGE_CURVE('',#15414,#15412,#9486,.T.);
#19173=EDGE_CURVE('',#15415,#15416,#10390,.T.);
#19174=EDGE_CURVE('',#15415,#15413,#9487,.T.);
#19175=EDGE_CURVE('',#15416,#15414,#9488,.T.);
#19176=EDGE_CURVE('',#15417,#15418,#10391,.T.);
#19177=EDGE_CURVE('',#15417,#15415,#9489,.T.);
#19178=EDGE_CURVE('',#15418,#15416,#9490,.T.);
#19179=EDGE_CURVE('',#15419,#15420,#10392,.T.);
#19180=EDGE_CURVE('',#15419,#15417,#9491,.T.);
#19181=EDGE_CURVE('',#15420,#15418,#9492,.T.);
#19182=EDGE_CURVE('',#15421,#15422,#10393,.T.);
#19183=EDGE_CURVE('',#15421,#15419,#9493,.T.);
#19184=EDGE_CURVE('',#15422,#15420,#9494,.T.);
#19185=EDGE_CURVE('',#15423,#15424,#10394,.T.);
#19186=EDGE_CURVE('',#15423,#15421,#9495,.T.);
#19187=EDGE_CURVE('',#15424,#15422,#9496,.T.);
#19188=EDGE_CURVE('',#15425,#15426,#10395,.T.);
#19189=EDGE_CURVE('',#15425,#15423,#9497,.T.);
#19190=EDGE_CURVE('',#15426,#15424,#9498,.T.);
#19191=EDGE_CURVE('',#15427,#15428,#10396,.T.);
#19192=EDGE_CURVE('',#15427,#15425,#9499,.T.);
#19193=EDGE_CURVE('',#15428,#15426,#9500,.T.);
#19194=EDGE_CURVE('',#15429,#15430,#10397,.T.);
#19195=EDGE_CURVE('',#15429,#15427,#9501,.T.);
#19196=EDGE_CURVE('',#15430,#15428,#9502,.T.);
#19197=EDGE_CURVE('',#15431,#15432,#10398,.T.);
#19198=EDGE_CURVE('',#15431,#15429,#9503,.T.);
#19199=EDGE_CURVE('',#15432,#15430,#9504,.T.);
#19200=EDGE_CURVE('',#15433,#15434,#10399,.T.);
#19201=EDGE_CURVE('',#15433,#15431,#9505,.T.);
#19202=EDGE_CURVE('',#15434,#15432,#9506,.T.);
#19203=EDGE_CURVE('',#15435,#15436,#10400,.T.);
#19204=EDGE_CURVE('',#15435,#15433,#9507,.T.);
#19205=EDGE_CURVE('',#15436,#15434,#9508,.T.);
#19206=EDGE_CURVE('',#15437,#15438,#10401,.T.);
#19207=EDGE_CURVE('',#15437,#15435,#9509,.T.);
#19208=EDGE_CURVE('',#15438,#15436,#9510,.T.);
#19209=EDGE_CURVE('',#15439,#15440,#10402,.T.);
#19210=EDGE_CURVE('',#15439,#15437,#9511,.T.);
#19211=EDGE_CURVE('',#15440,#15438,#9512,.T.);
#19212=EDGE_CURVE('',#15441,#15442,#10403,.T.);
#19213=EDGE_CURVE('',#15441,#15439,#9513,.T.);
#19214=EDGE_CURVE('',#15442,#15440,#9514,.T.);
#19215=EDGE_CURVE('',#15443,#15444,#10404,.T.);
#19216=EDGE_CURVE('',#15443,#15441,#9515,.T.);
#19217=EDGE_CURVE('',#15444,#15442,#9516,.T.);
#19218=EDGE_CURVE('',#15445,#15446,#10405,.T.);
#19219=EDGE_CURVE('',#15445,#15443,#9517,.T.);
#19220=EDGE_CURVE('',#15446,#15444,#9518,.T.);
#19221=EDGE_CURVE('',#15447,#15448,#10406,.T.);
#19222=EDGE_CURVE('',#15447,#15445,#9519,.T.);
#19223=EDGE_CURVE('',#15448,#15446,#9520,.T.);
#19224=EDGE_CURVE('',#15449,#15450,#10407,.T.);
#19225=EDGE_CURVE('',#15449,#15447,#9521,.T.);
#19226=EDGE_CURVE('',#15450,#15448,#9522,.T.);
#19227=EDGE_CURVE('',#15451,#15452,#10408,.T.);
#19228=EDGE_CURVE('',#15451,#15449,#9523,.T.);
#19229=EDGE_CURVE('',#15452,#15450,#9524,.T.);
#19230=EDGE_CURVE('',#15453,#15454,#10409,.T.);
#19231=EDGE_CURVE('',#15453,#15451,#9525,.T.);
#19232=EDGE_CURVE('',#15454,#15452,#9526,.T.);
#19233=EDGE_CURVE('',#15455,#15456,#10410,.T.);
#19234=EDGE_CURVE('',#15455,#15453,#9527,.T.);
#19235=EDGE_CURVE('',#15456,#15454,#9528,.T.);
#19236=EDGE_CURVE('',#15457,#15458,#10411,.T.);
#19237=EDGE_CURVE('',#15457,#15455,#9529,.T.);
#19238=EDGE_CURVE('',#15458,#15456,#9530,.T.);
#19239=EDGE_CURVE('',#15459,#15460,#10412,.T.);
#19240=EDGE_CURVE('',#15459,#15457,#9531,.T.);
#19241=EDGE_CURVE('',#15460,#15458,#9532,.T.);
#19242=EDGE_CURVE('',#15461,#15462,#10413,.T.);
#19243=EDGE_CURVE('',#15461,#15459,#9533,.T.);
#19244=EDGE_CURVE('',#15462,#15460,#9534,.T.);
#19245=EDGE_CURVE('',#15463,#15464,#10414,.T.);
#19246=EDGE_CURVE('',#15463,#15461,#9535,.T.);
#19247=EDGE_CURVE('',#15464,#15462,#9536,.T.);
#19248=EDGE_CURVE('',#15465,#15466,#7019,.T.);
#19249=EDGE_CURVE('',#15466,#15466,#9537,.T.);
#19250=EDGE_CURVE('',#15465,#15465,#9538,.T.);
#19251=EDGE_CURVE('',#15467,#15466,#1828,.T.);
#19252=EDGE_CURVE('',#15467,#15467,#9539,.T.);
#19253=EDGE_CURVE('',#15468,#15468,#7020,.T.);
#19254=EDGE_CURVE('',#15467,#15469,#7021,.T.);
#19255=EDGE_CURVE('',#15469,#15470,#9540,.T.);
#19256=EDGE_CURVE('',#15470,#15469,#9541,.T.);
#19257=EDGE_CURVE('',#15470,#15471,#10415,.T.);
#19258=EDGE_CURVE('',#15472,#15471,#9542,.T.);
#19259=EDGE_CURVE('',#15471,#15472,#9543,.T.);
#19260=EDGE_CURVE('',#15472,#15473,#7022,.T.);
#19261=EDGE_CURVE('',#15473,#15473,#9544,.T.);
#19262=EDGE_CURVE('',#15474,#15473,#1829,.T.);
#19263=EDGE_CURVE('',#15474,#15475,#7023,.T.);
#19264=EDGE_CURVE('',#15475,#15474,#7024,.T.);
#19265=EDGE_CURVE('',#15476,#15477,#7025,.T.);
#19266=EDGE_CURVE('',#15477,#15476,#7026,.T.);
#19267=EDGE_CURVE('',#15476,#15478,#7027,.T.);
#19268=EDGE_CURVE('',#15478,#15479,#7028,.T.);
#19269=EDGE_CURVE('',#15479,#15478,#7029,.T.);
#19270=EDGE_CURVE('',#15479,#15480,#10416,.T.);
#19271=EDGE_CURVE('',#15481,#15480,#7030,.T.);
#19272=EDGE_CURVE('',#15480,#15481,#7031,.T.);
#19273=EDGE_CURVE('',#15475,#15477,#10417,.T.);
#19274=EDGE_CURVE('',#15481,#15482,#7032,.T.);
#19275=EDGE_CURVE('',#15482,#15482,#7033,.T.);
#19276=EDGE_CURVE('',#15483,#15483,#7034,.T.);
#19277=EDGE_CURVE('',#15484,#15485,#7035,.T.);
#19278=EDGE_CURVE('',#15485,#15484,#7036,.T.);
#19279=EDGE_CURVE('',#15484,#15486,#7037,.T.);
#19280=EDGE_CURVE('',#15486,#15486,#7038,.T.);
#19281=EDGE_CURVE('',#15487,#15487,#7039,.T.);
#19282=EDGE_CURVE('',#15483,#15485,#10418,.T.);
#19283=EDGE_CURVE('',#15488,#15489,#7040,.T.);
#19284=EDGE_CURVE('',#15489,#15488,#7041,.T.);
#19285=EDGE_CURVE('',#15488,#15490,#7042,.T.);
#19286=EDGE_CURVE('',#15490,#15490,#7043,.T.);
#19287=EDGE_CURVE('',#15491,#15492,#10419,.T.);
#19288=EDGE_CURVE('',#15491,#15493,#7044,.T.);
#19289=EDGE_CURVE('',#15494,#15493,#10420,.T.);
#19290=EDGE_CURVE('',#15494,#15495,#7045,.T.);
#19291=EDGE_CURVE('',#15496,#15495,#10421,.T.);
#19292=EDGE_CURVE('',#15496,#15497,#7046,.T.);
#19293=EDGE_CURVE('',#15498,#15497,#10422,.T.);
#19294=EDGE_CURVE('',#15498,#15499,#7047,.T.);
#19295=EDGE_CURVE('',#15500,#15499,#10423,.T.);
#19296=EDGE_CURVE('',#15500,#15501,#7048,.T.);
#19297=EDGE_CURVE('',#15502,#15501,#10424,.T.);
#19298=EDGE_CURVE('',#15502,#15503,#7049,.T.);
#19299=EDGE_CURVE('',#15504,#15503,#10425,.T.);
#19300=EDGE_CURVE('',#15504,#15505,#7050,.T.);
#19301=EDGE_CURVE('',#15506,#15505,#10426,.T.);
#19302=EDGE_CURVE('',#15506,#15507,#7051,.T.);
#19303=EDGE_CURVE('',#15508,#15507,#10427,.T.);
#19304=EDGE_CURVE('',#15508,#15509,#7052,.T.);
#19305=EDGE_CURVE('',#15510,#15509,#10428,.T.);
#19306=EDGE_CURVE('',#15510,#15511,#7053,.T.);
#19307=EDGE_CURVE('',#15512,#15511,#10429,.T.);
#19308=EDGE_CURVE('',#15512,#15513,#7054,.T.);
#19309=EDGE_CURVE('',#15514,#15513,#10430,.T.);
#19310=EDGE_CURVE('',#15514,#15515,#7055,.T.);
#19311=EDGE_CURVE('',#15516,#15515,#10431,.T.);
#19312=EDGE_CURVE('',#15516,#15517,#7056,.T.);
#19313=EDGE_CURVE('',#15518,#15517,#10432,.T.);
#19314=EDGE_CURVE('',#15518,#15519,#7057,.T.);
#19315=EDGE_CURVE('',#15520,#15519,#10433,.T.);
#19316=EDGE_CURVE('',#15520,#15521,#7058,.T.);
#19317=EDGE_CURVE('',#15522,#15521,#10434,.T.);
#19318=EDGE_CURVE('',#15522,#15523,#7059,.T.);
#19319=EDGE_CURVE('',#15524,#15523,#10435,.T.);
#19320=EDGE_CURVE('',#15524,#15525,#7060,.T.);
#19321=EDGE_CURVE('',#15526,#15525,#10436,.T.);
#19322=EDGE_CURVE('',#15526,#15527,#7061,.T.);
#19323=EDGE_CURVE('',#15528,#15527,#10437,.T.);
#19324=EDGE_CURVE('',#15528,#15529,#7062,.T.);
#19325=EDGE_CURVE('',#15530,#15529,#10438,.T.);
#19326=EDGE_CURVE('',#15530,#15531,#7063,.T.);
#19327=EDGE_CURVE('',#15532,#15531,#10439,.T.);
#19328=EDGE_CURVE('',#15532,#15533,#7064,.T.);
#19329=EDGE_CURVE('',#15534,#15533,#10440,.T.);
#19330=EDGE_CURVE('',#15534,#15535,#7065,.T.);
#19331=EDGE_CURVE('',#15536,#15535,#10441,.T.);
#19332=EDGE_CURVE('',#15536,#15537,#7066,.T.);
#19333=EDGE_CURVE('',#15538,#15537,#10442,.T.);
#19334=EDGE_CURVE('',#15538,#15539,#7067,.T.);
#19335=EDGE_CURVE('',#15540,#15539,#10443,.T.);
#19336=EDGE_CURVE('',#15540,#15541,#7068,.T.);
#19337=EDGE_CURVE('',#15542,#15541,#10444,.T.);
#19338=EDGE_CURVE('',#15542,#15543,#7069,.T.);
#19339=EDGE_CURVE('',#15544,#15543,#10445,.T.);
#19340=EDGE_CURVE('',#15492,#15544,#7070,.F.);
#19341=EDGE_CURVE('',#15487,#15489,#10446,.T.);
#19342=EDGE_CURVE('',#15545,#15546,#9545,.T.);
#19343=EDGE_CURVE('',#15545,#15547,#9546,.T.);
#19344=EDGE_CURVE('',#15547,#15548,#9547,.F.);
#19345=EDGE_CURVE('',#15548,#15549,#9548,.F.);
#19346=EDGE_CURVE('',#15549,#15550,#9549,.T.);
#19347=EDGE_CURVE('',#15546,#15550,#9550,.T.);
#19348=EDGE_CURVE('',#15550,#15549,#7071,.T.);
#19349=EDGE_CURVE('',#15551,#15552,#9551,.T.);
#19350=EDGE_CURVE('',#15552,#15553,#9552,.F.);
#19351=EDGE_CURVE('',#15553,#15554,#9553,.F.);
#19352=EDGE_CURVE('',#15554,#15555,#9554,.T.);
#19353=EDGE_CURVE('',#15555,#15556,#9555,.T.);
#19354=EDGE_CURVE('',#15556,#15551,#9556,.T.);
#19355=EDGE_CURVE('',#15557,#15558,#9557,.T.);
#19356=EDGE_CURVE('',#15558,#15559,#7072,.T.);
#19357=EDGE_CURVE('',#15559,#15551,#9558,.T.);
#19358=EDGE_CURVE('',#15557,#15556,#9559,.T.);
#19359=EDGE_CURVE('',#15558,#15560,#9560,.T.);
#19360=EDGE_CURVE('',#15560,#15561,#7073,.T.);
#19361=EDGE_CURVE('',#15561,#15559,#9561,.T.);
#19362=EDGE_CURVE('',#15560,#15562,#7074,.T.);
#19363=EDGE_CURVE('',#15562,#15561,#7075,.T.);
#19364=EDGE_CURVE('',#15555,#15554,#7076,.T.);
#19365=EDGE_CURVE('',#15553,#15563,#9562,.F.);
#19366=EDGE_CURVE('',#15564,#15563,#9563,.T.);
#19367=EDGE_CURVE('',#15565,#15564,#9564,.T.);
#19368=EDGE_CURVE('',#15560,#15565,#9565,.T.);
#19369=EDGE_CURVE('',#15566,#15567,#7077,.T.);
#19370=EDGE_CURVE('',#15567,#15568,#7078,.T.);
#19371=EDGE_CURVE('',#15568,#15569,#7079,.T.);
#19372=EDGE_CURVE('',#15569,#15566,#7080,.T.);
#19373=EDGE_CURVE('',#15568,#15570,#7081,.T.);
#19374=EDGE_CURVE('',#15570,#15569,#7082,.T.);
#19375=EDGE_CURVE('',#15566,#15571,#7083,.T.);
#19376=EDGE_CURVE('',#15571,#15567,#7084,.T.);
#19377=EDGE_CURVE('',#15570,#15572,#9566,.T.);
#19378=EDGE_CURVE('',#15572,#15573,#7085,.T.);
#19379=EDGE_CURVE('',#15573,#15569,#9567,.T.);
#19380=EDGE_CURVE('',#15568,#15574,#9568,.T.);
#19381=EDGE_CURVE('',#15575,#15574,#7086,.T.);
#19382=EDGE_CURVE('',#15575,#15570,#9569,.T.);
#19383=EDGE_CURVE('',#15576,#15567,#9570,.T.);
#19384=EDGE_CURVE('',#15574,#15576,#7087,.T.);
#19385=EDGE_CURVE('',#15564,#15577,#7088,.T.);
#19386=EDGE_CURVE('',#15577,#15578,#9571,.T.);
#19387=EDGE_CURVE('',#15578,#15579,#7089,.T.);
#19388=EDGE_CURVE('',#15579,#15565,#7090,.T.);
#19389=EDGE_CURVE('',#15580,#15577,#9572,.T.);
#19390=EDGE_CURVE('',#15580,#15552,#9573,.T.);
#19391=EDGE_CURVE('',#15578,#15581,#7091,.T.);
#19392=EDGE_CURVE('',#15581,#15565,#7092,.T.);
#19393=EDGE_CURVE('',#15579,#15582,#7093,.T.);
#19394=EDGE_CURVE('',#15583,#15584,#7094,.T.);
#19395=EDGE_CURVE('',#15584,#15577,#7095,.T.);
#19396=EDGE_CURVE('',#15559,#15585,#7096,.T.);
#19397=EDGE_CURVE('',#15586,#15585,#9574,.T.);
#19398=EDGE_CURVE('',#15586,#15587,#9575,.T.);
#19399=EDGE_CURVE('',#15588,#15587,#9576,.T.);
#19400=EDGE_CURVE('',#15589,#15588,#9577,.T.);
#19401=EDGE_CURVE('',#15589,#15590,#7097,.T.);
#19402=EDGE_CURVE('',#15591,#15590,#9578,.T.);
#19403=EDGE_CURVE('',#15591,#15547,#9579,.T.);
#19404=EDGE_CURVE('',#15545,#15592,#9580,.T.);
#19405=EDGE_CURVE('',#15593,#15592,#9581,.T.);
#19406=EDGE_CURVE('',#15593,#15594,#7098,.T.);
#19407=EDGE_CURVE('',#15595,#15594,#9582,.T.);
#19408=EDGE_CURVE('',#15596,#15595,#9583,.T.);
#19409=EDGE_CURVE('',#15596,#15597,#9584,.T.);
#19410=EDGE_CURVE('',#15598,#15597,#9585,.T.);
#19411=EDGE_CURVE('',#15598,#15599,#7099,.T.);
#19412=EDGE_CURVE('',#15600,#15599,#9586,.T.);
#19413=EDGE_CURVE('',#15600,#15601,#9587,.T.);
#19414=EDGE_CURVE('',#15602,#15601,#9588,.T.);
#19415=EDGE_CURVE('',#15574,#15602,#9589,.T.);
#19416=EDGE_CURVE('',#15603,#15576,#9590,.T.);
#19417=EDGE_CURVE('',#15604,#15603,#9591,.T.);
#19418=EDGE_CURVE('',#15605,#15604,#9592,.T.);
#19419=EDGE_CURVE('',#15605,#15584,#7100,.T.);
#19420=EDGE_CURVE('',#15603,#15606,#9593,.T.);
#19421=EDGE_CURVE('',#15606,#15607,#9594,.T.);
#19422=EDGE_CURVE('',#15607,#15608,#9595,.T.);
#19423=EDGE_CURVE('',#15608,#15609,#9596,.T.);
#19424=EDGE_CURVE('',#15609,#15604,#9597,.T.);
#19425=EDGE_CURVE('',#15566,#15610,#9598,.T.);
#19426=EDGE_CURVE('',#15610,#15611,#7101,.T.);
#19427=EDGE_CURVE('',#15611,#15571,#9599,.T.);
#19428=EDGE_CURVE('',#15571,#15612,#9600,.T.);
#19429=EDGE_CURVE('',#15612,#15576,#7102,.T.);
#19430=EDGE_CURVE('',#15612,#15613,#9601,.T.);
#19431=EDGE_CURVE('',#15606,#15613,#9602,.T.);
#19432=EDGE_CURVE('',#15614,#15615,#9603,.T.);
#19433=EDGE_CURVE('',#15615,#15605,#7103,.T.);
#19434=EDGE_CURVE('',#15614,#15609,#9604,.T.);
#19435=EDGE_CURVE('',#15615,#15611,#9605,.T.);
#19436=EDGE_CURVE('',#15611,#15616,#7104,.T.);
#19437=EDGE_CURVE('',#15616,#15617,#7105,.T.);
#19438=EDGE_CURVE('',#15617,#15605,#9606,.T.);
#19439=EDGE_CURVE('',#15610,#15617,#7106,.T.);
#19440=EDGE_CURVE('',#15616,#15618,#7107,.T.);
#19441=EDGE_CURVE('',#15578,#15617,#7108,.T.);
#19442=EDGE_CURVE('',#15610,#15581,#7109,.T.);
#19443=EDGE_CURVE('',#15619,#15619,#7110,.T.);
#19444=EDGE_CURVE('',#15620,#15573,#7111,.T.);
#19445=EDGE_CURVE('',#15621,#15620,#9607,.T.);
#19446=EDGE_CURVE('',#15622,#15621,#7112,.T.);
#19447=EDGE_CURVE('',#15623,#15622,#9608,.T.);
#19448=EDGE_CURVE('',#15624,#15623,#7113,.T.);
#19449=EDGE_CURVE('',#15625,#15624,#9609,.T.);
#19450=EDGE_CURVE('',#15562,#15625,#7114,.T.);
#19451=EDGE_CURVE('',#15581,#15562,#9610,.T.);
#19452=EDGE_CURVE('',#15608,#15607,#7115,.T.);
#19453=EDGE_CURVE('',#15601,#15626,#9611,.F.);
#19454=EDGE_CURVE('',#15626,#15627,#9612,.F.);
#19455=EDGE_CURVE('',#15627,#15628,#9613,.T.);
#19456=EDGE_CURVE('',#15628,#15629,#9614,.T.);
#19457=EDGE_CURVE('',#15629,#15602,#9615,.T.);
#19458=EDGE_CURVE('',#15630,#15575,#9616,.T.);
#19459=EDGE_CURVE('',#15630,#15629,#9617,.T.);
#19460=EDGE_CURVE('',#15572,#15631,#7116,.T.);
#19461=EDGE_CURVE('',#15631,#15573,#7117,.T.);
#19462=EDGE_CURVE('',#15631,#15632,#7118,.T.);
#19463=EDGE_CURVE('',#15632,#15620,#7119,.T.);
#19464=EDGE_CURVE('',#15572,#15633,#9618,.T.);
#19465=EDGE_CURVE('',#15633,#15599,#7120,.T.);
#19466=EDGE_CURVE('',#15599,#15631,#9619,.T.);
#19467=EDGE_CURVE('',#15633,#15634,#9620,.T.);
#19468=EDGE_CURVE('',#15626,#15634,#9621,.F.);
#19469=EDGE_CURVE('',#15635,#15632,#7121,.T.);
#19470=EDGE_CURVE('',#15632,#15598,#9622,.T.);
#19471=EDGE_CURVE('',#15598,#15636,#7122,.T.);
#19472=EDGE_CURVE('',#15636,#15635,#9623,.T.);
#19473=EDGE_CURVE('',#15597,#15637,#9624,.F.);
#19474=EDGE_CURVE('',#15637,#15636,#9625,.T.);
#19475=EDGE_CURVE('',#15635,#15620,#7123,.T.);
#19476=EDGE_CURVE('',#15628,#15627,#7124,.T.);
#19477=EDGE_CURVE('',#15635,#15638,#9626,.T.);
#19478=EDGE_CURVE('',#15621,#15638,#7125,.T.);
#19479=EDGE_CURVE('',#15639,#15640,#7126,.T.);
#19480=EDGE_CURVE('',#15640,#15641,#7127,.T.);
#19481=EDGE_CURVE('',#15641,#15593,#9627,.T.);
#19482=EDGE_CURVE('',#15593,#15642,#7128,.T.);
#19483=EDGE_CURVE('',#15642,#15639,#9628,.T.);
#19484=EDGE_CURVE('',#15639,#15622,#7129,.T.);
#19485=EDGE_CURVE('',#15622,#15641,#7130,.T.);
#19486=EDGE_CURVE('',#15643,#15640,#7131,.T.);
#19487=EDGE_CURVE('',#15644,#15642,#9629,.T.);
#19488=EDGE_CURVE('',#15546,#15644,#9630,.T.);
#19489=EDGE_CURVE('',#15645,#15641,#7132,.T.);
#19490=EDGE_CURVE('',#15594,#15645,#9631,.T.);
#19491=EDGE_CURVE('',#15646,#15647,#7133,.T.);
#19492=EDGE_CURVE('',#15647,#15623,#7134,.T.);
#19493=EDGE_CURVE('',#15623,#15646,#7135,.T.);
#19494=EDGE_CURVE('',#15648,#15590,#7136,.T.);
#19495=EDGE_CURVE('',#15590,#15647,#9632,.T.);
#19496=EDGE_CURVE('',#15646,#15648,#9633,.T.);
#19497=EDGE_CURVE('',#15648,#15649,#9634,.T.);
#19498=EDGE_CURVE('',#15548,#15649,#9635,.F.);
#19499=EDGE_CURVE('',#15639,#15646,#9636,.T.);
#19500=EDGE_CURVE('',#15647,#15650,#7137,.T.);
#19501=EDGE_CURVE('',#15624,#15650,#7138,.T.);
#19502=EDGE_CURVE('',#15587,#15651,#9637,.F.);
#19503=EDGE_CURVE('',#15651,#15652,#9638,.F.);
#19504=EDGE_CURVE('',#15652,#15653,#9639,.T.);
#19505=EDGE_CURVE('',#15653,#15654,#9640,.T.);
#19506=EDGE_CURVE('',#15654,#15588,#9641,.T.);
#19507=EDGE_CURVE('',#15655,#15656,#9642,.T.);
#19508=EDGE_CURVE('',#15656,#15589,#7139,.T.);
#19509=EDGE_CURVE('',#15655,#15654,#9643,.T.);
#19510=EDGE_CURVE('',#15656,#15657,#9644,.T.);
#19511=EDGE_CURVE('',#15657,#15650,#7140,.T.);
#19512=EDGE_CURVE('',#15650,#15589,#9645,.T.);
#19513=EDGE_CURVE('',#15657,#15624,#7141,.T.);
#19514=EDGE_CURVE('',#15653,#15652,#7142,.T.);
#19515=EDGE_CURVE('',#15651,#15658,#9646,.F.);
#19516=EDGE_CURVE('',#15659,#15658,#9647,.T.);
#19517=EDGE_CURVE('',#15660,#15659,#9648,.T.);
#19518=EDGE_CURVE('',#15657,#15660,#9649,.T.);
#19519=EDGE_CURVE('',#15659,#15585,#7143,.T.);
#19520=EDGE_CURVE('',#15585,#15661,#9650,.T.);
#19521=EDGE_CURVE('',#15661,#15660,#7144,.T.);
#19522=EDGE_CURVE('',#15661,#15625,#7145,.T.);
#19523=EDGE_CURVE('',#15625,#15660,#7146,.T.);
#19524=EDGE_CURVE('',#15661,#15561,#7147,.T.);
#19525=EDGE_CURVE('',#15645,#15621,#7148,.T.);
#19526=EDGE_CURVE('',#15638,#15662,#7149,.T.);
#19527=EDGE_CURVE('',#15663,#15662,#7150,.T.);
#19528=EDGE_CURVE('',#15662,#15645,#7151,.T.);
#19529=EDGE_CURVE('',#15638,#15664,#9651,.T.);
#19530=EDGE_CURVE('',#15664,#15594,#7152,.T.);
#19531=EDGE_CURVE('',#15619,#15665,#7153,.T.);
#19532=EDGE_CURVE('',#15665,#15666,#7154,.T.);
#19533=EDGE_CURVE('',#15666,#15665,#7155,.T.);
#19534=EDGE_CURVE('',#15666,#15468,#10447,.T.);
#19535=EDGE_CURVE('',#15667,#15668,#9652,.T.);
#19536=EDGE_CURVE('',#15668,#15637,#9653,.F.);
#19537=EDGE_CURVE('',#15595,#15669,#9654,.T.);
#19538=EDGE_CURVE('',#15669,#15667,#9655,.T.);
#19539=EDGE_CURVE('',#15664,#15670,#9656,.T.);
#19540=EDGE_CURVE('',#15669,#15670,#9657,.T.);
#19541=EDGE_CURVE('',#15671,#15491,#10448,.T.);
#19542=EDGE_CURVE('',#15671,#15672,#7156,.T.);
#19543=EDGE_CURVE('',#15672,#15493,#10449,.T.);
#19544=EDGE_CURVE('',#15671,#15673,#10450,.T.);
#19545=EDGE_CURVE('',#15674,#15673,#7157,.T.);
#19546=EDGE_CURVE('',#15674,#15675,#10451,.T.);
#19547=EDGE_CURVE('',#15676,#15675,#7158,.T.);
#19548=EDGE_CURVE('',#15676,#15677,#10452,.T.);
#19549=EDGE_CURVE('',#15678,#15677,#7159,.T.);
#19550=EDGE_CURVE('',#15678,#15679,#10453,.T.);
#19551=EDGE_CURVE('',#15680,#15679,#7160,.T.);
#19552=EDGE_CURVE('',#15680,#15681,#10454,.T.);
#19553=EDGE_CURVE('',#15682,#15681,#7161,.T.);
#19554=EDGE_CURVE('',#15682,#15683,#10455,.T.);
#19555=EDGE_CURVE('',#15684,#15683,#7162,.T.);
#19556=EDGE_CURVE('',#15684,#15685,#10456,.T.);
#19557=EDGE_CURVE('',#15686,#15685,#7163,.T.);
#19558=EDGE_CURVE('',#15686,#15687,#10457,.T.);
#19559=EDGE_CURVE('',#15688,#15687,#7164,.T.);
#19560=EDGE_CURVE('',#15688,#15689,#10458,.T.);
#19561=EDGE_CURVE('',#15690,#15689,#7165,.T.);
#19562=EDGE_CURVE('',#15690,#15691,#10459,.T.);
#19563=EDGE_CURVE('',#15692,#15691,#7166,.T.);
#19564=EDGE_CURVE('',#15692,#15693,#10460,.T.);
#19565=EDGE_CURVE('',#15694,#15693,#7167,.T.);
#19566=EDGE_CURVE('',#15694,#15695,#10461,.T.);
#19567=EDGE_CURVE('',#15696,#15695,#7168,.T.);
#19568=EDGE_CURVE('',#15696,#15697,#10462,.T.);
#19569=EDGE_CURVE('',#15698,#15697,#7169,.T.);
#19570=EDGE_CURVE('',#15698,#15699,#10463,.T.);
#19571=EDGE_CURVE('',#15700,#15699,#7170,.T.);
#19572=EDGE_CURVE('',#15700,#15701,#10464,.T.);
#19573=EDGE_CURVE('',#15702,#15701,#7171,.T.);
#19574=EDGE_CURVE('',#15702,#15703,#10465,.T.);
#19575=EDGE_CURVE('',#15704,#15703,#7172,.T.);
#19576=EDGE_CURVE('',#15704,#15705,#10466,.T.);
#19577=EDGE_CURVE('',#15706,#15705,#7173,.T.);
#19578=EDGE_CURVE('',#15706,#15707,#10467,.T.);
#19579=EDGE_CURVE('',#15708,#15707,#7174,.T.);
#19580=EDGE_CURVE('',#15708,#15709,#10468,.T.);
#19581=EDGE_CURVE('',#15710,#15709,#7175,.T.);
#19582=EDGE_CURVE('',#15710,#15711,#10469,.T.);
#19583=EDGE_CURVE('',#15712,#15711,#7176,.T.);
#19584=EDGE_CURVE('',#15712,#15713,#10470,.T.);
#19585=EDGE_CURVE('',#15714,#15713,#7177,.T.);
#19586=EDGE_CURVE('',#15714,#15715,#10471,.T.);
#19587=EDGE_CURVE('',#15716,#15715,#7178,.T.);
#19588=EDGE_CURVE('',#15716,#15717,#10472,.T.);
#19589=EDGE_CURVE('',#15718,#15717,#7179,.T.);
#19590=EDGE_CURVE('',#15718,#15719,#10473,.T.);
#19591=EDGE_CURVE('',#15720,#15719,#7180,.T.);
#19592=EDGE_CURVE('',#15720,#15721,#10474,.T.);
#19593=EDGE_CURVE('',#15722,#15721,#7181,.T.);
#19594=EDGE_CURVE('',#15722,#15723,#10475,.T.);
#19595=EDGE_CURVE('',#15724,#15723,#7182,.T.);
#19596=EDGE_CURVE('',#15724,#15672,#10476,.T.);
#19597=EDGE_CURVE('',#15404,#15725,#7183,.T.);
#19598=EDGE_CURVE('',#15725,#15410,#9658,.T.);
#19599=EDGE_CURVE('',#15409,#15406,#9659,.T.);
#19600=EDGE_CURVE('',#15724,#15494,#10477,.T.);
#19601=EDGE_CURVE('',#15723,#15495,#10478,.T.);
#19602=EDGE_CURVE('',#15722,#15496,#10479,.T.);
#19603=EDGE_CURVE('',#15721,#15497,#10480,.T.);
#19604=EDGE_CURVE('',#15720,#15498,#10481,.T.);
#19605=EDGE_CURVE('',#15719,#15499,#10482,.T.);
#19606=EDGE_CURVE('',#15718,#15500,#10483,.T.);
#19607=EDGE_CURVE('',#15717,#15501,#10484,.T.);
#19608=EDGE_CURVE('',#15716,#15502,#10485,.T.);
#19609=EDGE_CURVE('',#15715,#15503,#10486,.T.);
#19610=EDGE_CURVE('',#15714,#15504,#10487,.T.);
#19611=EDGE_CURVE('',#15713,#15505,#10488,.T.);
#19612=EDGE_CURVE('',#15712,#15506,#10489,.T.);
#19613=EDGE_CURVE('',#15711,#15507,#10490,.T.);
#19614=EDGE_CURVE('',#15710,#15508,#10491,.T.);
#19615=EDGE_CURVE('',#15709,#15509,#10492,.T.);
#19616=EDGE_CURVE('',#15708,#15510,#10493,.T.);
#19617=EDGE_CURVE('',#15707,#15511,#10494,.T.);
#19618=EDGE_CURVE('',#15706,#15512,#10495,.T.);
#19619=EDGE_CURVE('',#15705,#15513,#10496,.T.);
#19620=EDGE_CURVE('',#15704,#15514,#10497,.T.);
#19621=EDGE_CURVE('',#15703,#15515,#10498,.T.);
#19622=EDGE_CURVE('',#15702,#15516,#10499,.T.);
#19623=EDGE_CURVE('',#15701,#15517,#10500,.T.);
#19624=EDGE_CURVE('',#15700,#15518,#10501,.T.);
#19625=EDGE_CURVE('',#15699,#15519,#10502,.T.);
#19626=EDGE_CURVE('',#15698,#15520,#10503,.T.);
#19627=EDGE_CURVE('',#15697,#15521,#10504,.T.);
#19628=EDGE_CURVE('',#15696,#15522,#10505,.T.);
#19629=EDGE_CURVE('',#15695,#15523,#10506,.T.);
#19630=EDGE_CURVE('',#15694,#15524,#10507,.T.);
#19631=EDGE_CURVE('',#15693,#15525,#10508,.T.);
#19632=EDGE_CURVE('',#15692,#15526,#10509,.T.);
#19633=EDGE_CURVE('',#15691,#15527,#10510,.T.);
#19634=EDGE_CURVE('',#15690,#15528,#10511,.T.);
#19635=EDGE_CURVE('',#15689,#15529,#10512,.T.);
#19636=EDGE_CURVE('',#15688,#15530,#10513,.T.);
#19637=EDGE_CURVE('',#15687,#15531,#10514,.T.);
#19638=EDGE_CURVE('',#15686,#15532,#10515,.T.);
#19639=EDGE_CURVE('',#15685,#15533,#10516,.T.);
#19640=EDGE_CURVE('',#15684,#15534,#10517,.T.);
#19641=EDGE_CURVE('',#15683,#15535,#10518,.T.);
#19642=EDGE_CURVE('',#15682,#15536,#10519,.T.);
#19643=EDGE_CURVE('',#15681,#15537,#10520,.T.);
#19644=EDGE_CURVE('',#15726,#15351,#9660,.T.);
#19645=EDGE_CURVE('',#15348,#15727,#9661,.T.);
#19646=EDGE_CURVE('',#15727,#15728,#7184,.T.);
#19647=EDGE_CURVE('',#15728,#15726,#9662,.T.);
#19648=EDGE_CURVE('',#15729,#15726,#9663,.T.);
#19649=EDGE_CURVE('',#15729,#15464,#9664,.T.);
#19650=EDGE_CURVE('',#15405,#15725,#9665,.T.);
#19651=EDGE_CURVE('',#15728,#15730,#9666,.T.);
#19652=EDGE_CURVE('',#15731,#15730,#9667,.T.);
#19653=EDGE_CURVE('',#15731,#15732,#9668,.F.);
#19654=EDGE_CURVE('',#15729,#15732,#9669,.T.);
#19655=EDGE_CURVE('',#15733,#15727,#9670,.T.);
#19656=EDGE_CURVE('',#15734,#15733,#7185,.T.);
#19657=EDGE_CURVE('',#15730,#15734,#7186,.T.);
#19658=EDGE_CURVE('',#15680,#15538,#10521,.T.);
#19659=EDGE_CURVE('',#15679,#15539,#10522,.T.);
#19660=EDGE_CURVE('',#15673,#15492,#10523,.T.);
#19661=EDGE_CURVE('',#15674,#15544,#10524,.T.);
#19662=EDGE_CURVE('',#15678,#15540,#10525,.T.);
#19663=EDGE_CURVE('',#15677,#15541,#10526,.T.);
#19664=EDGE_CURVE('',#15734,#15735,#7187,.T.);
#19665=EDGE_CURVE('',#15735,#15735,#7188,.T.);
#19666=EDGE_CURVE('',#15733,#15731,#9671,.T.);
#19667=EDGE_CURVE('',#15736,#15736,#7189,.T.);
#19668=EDGE_CURVE('',#15676,#15542,#10527,.T.);
#19669=EDGE_CURVE('',#15675,#15543,#10528,.T.);
#19670=EDGE_CURVE('',#15737,#15737,#7190,.T.);
#19671=EDGE_CURVE('',#15737,#15736,#7191,.T.);
#19672=EDGE_CURVE('',#15737,#15738,#10529,.T.);
#19673=EDGE_CURVE('',#15738,#15738,#7192,.T.);
#19674=EDGE_CURVE('',#15732,#15739,#9672,.T.);
#19675=EDGE_CURVE('',#15739,#15463,#9673,.T.);
#19676=EDGE_CURVE('',#15738,#15740,#10530,.T.);
#19677=EDGE_CURVE('',#15668,#15667,#7193,.T.);
#25125=ORIENTED_EDGE('',*,*,#19074,.F.);
#25126=ORIENTED_EDGE('',*,*,#19075,.T.);
#25127=ORIENTED_EDGE('',*,*,#19076,.F.);
#25128=ORIENTED_EDGE('',*,*,#19077,.F.);
#25129=ORIENTED_EDGE('',*,*,#19078,.T.);
#25130=ORIENTED_EDGE('',*,*,#19074,.T.);
#25131=ORIENTED_EDGE('',*,*,#19079,.F.);
#25132=ORIENTED_EDGE('',*,*,#19080,.T.);
#25133=ORIENTED_EDGE('',*,*,#19081,.F.);
#25134=ORIENTED_EDGE('',*,*,#19082,.T.);
#25135=ORIENTED_EDGE('',*,*,#19077,.T.);
#25136=ORIENTED_EDGE('',*,*,#19083,.T.);
#25137=ORIENTED_EDGE('',*,*,#19084,.F.);
#25138=ORIENTED_EDGE('',*,*,#19085,.T.);
#25139=ORIENTED_EDGE('',*,*,#19081,.T.);
#25140=ORIENTED_EDGE('',*,*,#19086,.T.);
#25141=ORIENTED_EDGE('',*,*,#19087,.F.);
#25142=ORIENTED_EDGE('',*,*,#19088,.T.);
#25143=ORIENTED_EDGE('',*,*,#19084,.T.);
#25144=ORIENTED_EDGE('',*,*,#19089,.T.);
#25145=ORIENTED_EDGE('',*,*,#19090,.F.);
#25146=ORIENTED_EDGE('',*,*,#19091,.T.);
#25147=ORIENTED_EDGE('',*,*,#19087,.T.);
#25148=ORIENTED_EDGE('',*,*,#19092,.T.);
#25149=ORIENTED_EDGE('',*,*,#19093,.F.);
#25150=ORIENTED_EDGE('',*,*,#19094,.T.);
#25151=ORIENTED_EDGE('',*,*,#19090,.T.);
#25152=ORIENTED_EDGE('',*,*,#19095,.T.);
#25153=ORIENTED_EDGE('',*,*,#19096,.F.);
#25154=ORIENTED_EDGE('',*,*,#19097,.T.);
#25155=ORIENTED_EDGE('',*,*,#19093,.T.);
#25156=ORIENTED_EDGE('',*,*,#19098,.T.);
#25157=ORIENTED_EDGE('',*,*,#19099,.F.);
#25158=ORIENTED_EDGE('',*,*,#19100,.T.);
#25159=ORIENTED_EDGE('',*,*,#19096,.T.);
#25160=ORIENTED_EDGE('',*,*,#19101,.T.);
#25161=ORIENTED_EDGE('',*,*,#19102,.F.);
#25162=ORIENTED_EDGE('',*,*,#19103,.T.);
#25163=ORIENTED_EDGE('',*,*,#19099,.T.);
#25164=ORIENTED_EDGE('',*,*,#19104,.T.);
#25165=ORIENTED_EDGE('',*,*,#19105,.F.);
#25166=ORIENTED_EDGE('',*,*,#19106,.T.);
#25167=ORIENTED_EDGE('',*,*,#19102,.T.);
#25168=ORIENTED_EDGE('',*,*,#19107,.T.);
#25169=ORIENTED_EDGE('',*,*,#19108,.F.);
#25170=ORIENTED_EDGE('',*,*,#19109,.T.);
#25171=ORIENTED_EDGE('',*,*,#19105,.T.);
#25172=ORIENTED_EDGE('',*,*,#19110,.T.);
#25173=ORIENTED_EDGE('',*,*,#19111,.F.);
#25174=ORIENTED_EDGE('',*,*,#19112,.T.);
#25175=ORIENTED_EDGE('',*,*,#19108,.T.);
#25176=ORIENTED_EDGE('',*,*,#19113,.T.);
#25177=ORIENTED_EDGE('',*,*,#19114,.F.);
#25178=ORIENTED_EDGE('',*,*,#19115,.T.);
#25179=ORIENTED_EDGE('',*,*,#19111,.T.);
#25180=ORIENTED_EDGE('',*,*,#19116,.T.);
#25181=ORIENTED_EDGE('',*,*,#19117,.F.);
#25182=ORIENTED_EDGE('',*,*,#19118,.T.);
#25183=ORIENTED_EDGE('',*,*,#19114,.T.);
#25184=ORIENTED_EDGE('',*,*,#19119,.T.);
#25185=ORIENTED_EDGE('',*,*,#19120,.F.);
#25186=ORIENTED_EDGE('',*,*,#19121,.T.);
#25187=ORIENTED_EDGE('',*,*,#19117,.T.);
#25188=ORIENTED_EDGE('',*,*,#19122,.T.);
#25189=ORIENTED_EDGE('',*,*,#19123,.F.);
#25190=ORIENTED_EDGE('',*,*,#19124,.T.);
#25191=ORIENTED_EDGE('',*,*,#19120,.T.);
#25192=ORIENTED_EDGE('',*,*,#19125,.T.);
#25193=ORIENTED_EDGE('',*,*,#19126,.F.);
#25194=ORIENTED_EDGE('',*,*,#19127,.T.);
#25195=ORIENTED_EDGE('',*,*,#19123,.T.);
#25196=ORIENTED_EDGE('',*,*,#19128,.T.);
#25197=ORIENTED_EDGE('',*,*,#19129,.F.);
#25198=ORIENTED_EDGE('',*,*,#19130,.T.);
#25199=ORIENTED_EDGE('',*,*,#19126,.T.);
#25200=ORIENTED_EDGE('',*,*,#19131,.T.);
#25201=ORIENTED_EDGE('',*,*,#19132,.F.);
#25202=ORIENTED_EDGE('',*,*,#19133,.T.);
#25203=ORIENTED_EDGE('',*,*,#19129,.T.);
#25204=ORIENTED_EDGE('',*,*,#19134,.T.);
#25205=ORIENTED_EDGE('',*,*,#19135,.F.);
#25206=ORIENTED_EDGE('',*,*,#19136,.T.);
#25207=ORIENTED_EDGE('',*,*,#19132,.T.);
#25208=ORIENTED_EDGE('',*,*,#19137,.T.);
#25209=ORIENTED_EDGE('',*,*,#19138,.F.);
#25210=ORIENTED_EDGE('',*,*,#19139,.T.);
#25211=ORIENTED_EDGE('',*,*,#19135,.T.);
#25212=ORIENTED_EDGE('',*,*,#19140,.T.);
#25213=ORIENTED_EDGE('',*,*,#19141,.F.);
#25214=ORIENTED_EDGE('',*,*,#19142,.T.);
#25215=ORIENTED_EDGE('',*,*,#19138,.T.);
#25216=ORIENTED_EDGE('',*,*,#19143,.T.);
#25217=ORIENTED_EDGE('',*,*,#19144,.F.);
#25218=ORIENTED_EDGE('',*,*,#19145,.T.);
#25219=ORIENTED_EDGE('',*,*,#19141,.T.);
#25220=ORIENTED_EDGE('',*,*,#19146,.T.);
#25221=ORIENTED_EDGE('',*,*,#19147,.F.);
#25222=ORIENTED_EDGE('',*,*,#19148,.T.);
#25223=ORIENTED_EDGE('',*,*,#19144,.T.);
#25224=ORIENTED_EDGE('',*,*,#19149,.T.);
#25225=ORIENTED_EDGE('',*,*,#19150,.F.);
#25226=ORIENTED_EDGE('',*,*,#19151,.T.);
#25227=ORIENTED_EDGE('',*,*,#19147,.T.);
#25228=ORIENTED_EDGE('',*,*,#19152,.T.);
#25229=ORIENTED_EDGE('',*,*,#19153,.F.);
#25230=ORIENTED_EDGE('',*,*,#19154,.T.);
#25231=ORIENTED_EDGE('',*,*,#19150,.T.);
#25232=ORIENTED_EDGE('',*,*,#19155,.T.);
#25233=ORIENTED_EDGE('',*,*,#19156,.F.);
#25234=ORIENTED_EDGE('',*,*,#19157,.T.);
#25235=ORIENTED_EDGE('',*,*,#19153,.T.);
#25236=ORIENTED_EDGE('',*,*,#19158,.T.);
#25237=ORIENTED_EDGE('',*,*,#19159,.F.);
#25238=ORIENTED_EDGE('',*,*,#19160,.F.);
#25239=ORIENTED_EDGE('',*,*,#19161,.T.);
#25240=ORIENTED_EDGE('',*,*,#19156,.T.);
#25241=ORIENTED_EDGE('',*,*,#19162,.T.);
#25242=ORIENTED_EDGE('',*,*,#19163,.F.);
#25243=ORIENTED_EDGE('',*,*,#19164,.T.);
#25244=ORIENTED_EDGE('',*,*,#19165,.F.);
#25245=ORIENTED_EDGE('',*,*,#19166,.F.);
#25246=ORIENTED_EDGE('',*,*,#19167,.F.);
#25247=ORIENTED_EDGE('',*,*,#19168,.T.);
#25248=ORIENTED_EDGE('',*,*,#19163,.T.);
#25249=ORIENTED_EDGE('',*,*,#19169,.F.);
#25250=ORIENTED_EDGE('',*,*,#19170,.F.);
#25251=ORIENTED_EDGE('',*,*,#19171,.T.);
#25252=ORIENTED_EDGE('',*,*,#19167,.T.);
#25253=ORIENTED_EDGE('',*,*,#19172,.F.);
#25254=ORIENTED_EDGE('',*,*,#19173,.F.);
#25255=ORIENTED_EDGE('',*,*,#19174,.T.);
#25256=ORIENTED_EDGE('',*,*,#19170,.T.);
#25257=ORIENTED_EDGE('',*,*,#19175,.F.);
#25258=ORIENTED_EDGE('',*,*,#19176,.F.);
#25259=ORIENTED_EDGE('',*,*,#19177,.T.);
#25260=ORIENTED_EDGE('',*,*,#19173,.T.);
#25261=ORIENTED_EDGE('',*,*,#19178,.F.);
#25262=ORIENTED_EDGE('',*,*,#19179,.F.);
#25263=ORIENTED_EDGE('',*,*,#19180,.T.);
#25264=ORIENTED_EDGE('',*,*,#19176,.T.);
#25265=ORIENTED_EDGE('',*,*,#19181,.F.);
#25266=ORIENTED_EDGE('',*,*,#19182,.F.);
#25267=ORIENTED_EDGE('',*,*,#19183,.T.);
#25268=ORIENTED_EDGE('',*,*,#19179,.T.);
#25269=ORIENTED_EDGE('',*,*,#19184,.F.);
#25270=ORIENTED_EDGE('',*,*,#19185,.F.);
#25271=ORIENTED_EDGE('',*,*,#19186,.T.);
#25272=ORIENTED_EDGE('',*,*,#19182,.T.);
#25273=ORIENTED_EDGE('',*,*,#19187,.F.);
#25274=ORIENTED_EDGE('',*,*,#19188,.F.);
#25275=ORIENTED_EDGE('',*,*,#19189,.T.);
#25276=ORIENTED_EDGE('',*,*,#19185,.T.);
#25277=ORIENTED_EDGE('',*,*,#19190,.F.);
#25278=ORIENTED_EDGE('',*,*,#19191,.F.);
#25279=ORIENTED_EDGE('',*,*,#19192,.T.);
#25280=ORIENTED_EDGE('',*,*,#19188,.T.);
#25281=ORIENTED_EDGE('',*,*,#19193,.F.);
#25282=ORIENTED_EDGE('',*,*,#19194,.F.);
#25283=ORIENTED_EDGE('',*,*,#19195,.T.);
#25284=ORIENTED_EDGE('',*,*,#19191,.T.);
#25285=ORIENTED_EDGE('',*,*,#19196,.F.);
#25286=ORIENTED_EDGE('',*,*,#19197,.F.);
#25287=ORIENTED_EDGE('',*,*,#19198,.T.);
#25288=ORIENTED_EDGE('',*,*,#19194,.T.);
#25289=ORIENTED_EDGE('',*,*,#19199,.F.);
#25290=ORIENTED_EDGE('',*,*,#19200,.F.);
#25291=ORIENTED_EDGE('',*,*,#19201,.T.);
#25292=ORIENTED_EDGE('',*,*,#19197,.T.);
#25293=ORIENTED_EDGE('',*,*,#19202,.F.);
#25294=ORIENTED_EDGE('',*,*,#19203,.F.);
#25295=ORIENTED_EDGE('',*,*,#19204,.T.);
#25296=ORIENTED_EDGE('',*,*,#19200,.T.);
#25297=ORIENTED_EDGE('',*,*,#19205,.F.);
#25298=ORIENTED_EDGE('',*,*,#19206,.F.);
#25299=ORIENTED_EDGE('',*,*,#19207,.T.);
#25300=ORIENTED_EDGE('',*,*,#19203,.T.);
#25301=ORIENTED_EDGE('',*,*,#19208,.F.);
#25302=ORIENTED_EDGE('',*,*,#19209,.F.);
#25303=ORIENTED_EDGE('',*,*,#19210,.T.);
#25304=ORIENTED_EDGE('',*,*,#19206,.T.);
#25305=ORIENTED_EDGE('',*,*,#19211,.F.);
#25306=ORIENTED_EDGE('',*,*,#19212,.F.);
#25307=ORIENTED_EDGE('',*,*,#19213,.T.);
#25308=ORIENTED_EDGE('',*,*,#19209,.T.);
#25309=ORIENTED_EDGE('',*,*,#19214,.F.);
#25310=ORIENTED_EDGE('',*,*,#19215,.F.);
#25311=ORIENTED_EDGE('',*,*,#19216,.T.);
#25312=ORIENTED_EDGE('',*,*,#19212,.T.);
#25313=ORIENTED_EDGE('',*,*,#19217,.F.);
#25314=ORIENTED_EDGE('',*,*,#19218,.F.);
#25315=ORIENTED_EDGE('',*,*,#19219,.T.);
#25316=ORIENTED_EDGE('',*,*,#19215,.T.);
#25317=ORIENTED_EDGE('',*,*,#19220,.F.);
#25318=ORIENTED_EDGE('',*,*,#19221,.F.);
#25319=ORIENTED_EDGE('',*,*,#19222,.T.);
#25320=ORIENTED_EDGE('',*,*,#19218,.T.);
#25321=ORIENTED_EDGE('',*,*,#19223,.F.);
#25322=ORIENTED_EDGE('',*,*,#19224,.F.);
#25323=ORIENTED_EDGE('',*,*,#19225,.T.);
#25324=ORIENTED_EDGE('',*,*,#19221,.T.);
#25325=ORIENTED_EDGE('',*,*,#19226,.F.);
#25326=ORIENTED_EDGE('',*,*,#19227,.F.);
#25327=ORIENTED_EDGE('',*,*,#19228,.T.);
#25328=ORIENTED_EDGE('',*,*,#19224,.T.);
#25329=ORIENTED_EDGE('',*,*,#19229,.F.);
#25330=ORIENTED_EDGE('',*,*,#19230,.F.);
#25331=ORIENTED_EDGE('',*,*,#19231,.T.);
#25332=ORIENTED_EDGE('',*,*,#19227,.T.);
#25333=ORIENTED_EDGE('',*,*,#19232,.F.);
#25334=ORIENTED_EDGE('',*,*,#19233,.F.);
#25335=ORIENTED_EDGE('',*,*,#19234,.T.);
#25336=ORIENTED_EDGE('',*,*,#19230,.T.);
#25337=ORIENTED_EDGE('',*,*,#19235,.F.);
#25338=ORIENTED_EDGE('',*,*,#19236,.F.);
#25339=ORIENTED_EDGE('',*,*,#19237,.T.);
#25340=ORIENTED_EDGE('',*,*,#19233,.T.);
#25341=ORIENTED_EDGE('',*,*,#19238,.F.);
#25342=ORIENTED_EDGE('',*,*,#19239,.F.);
#25343=ORIENTED_EDGE('',*,*,#19240,.T.);
#25344=ORIENTED_EDGE('',*,*,#19236,.T.);
#25345=ORIENTED_EDGE('',*,*,#19241,.F.);
#25346=ORIENTED_EDGE('',*,*,#19242,.F.);
#25347=ORIENTED_EDGE('',*,*,#19243,.T.);
#25348=ORIENTED_EDGE('',*,*,#19239,.T.);
#25349=ORIENTED_EDGE('',*,*,#19244,.F.);
#25350=ORIENTED_EDGE('',*,*,#19245,.F.);
#25351=ORIENTED_EDGE('',*,*,#19246,.T.);
#25352=ORIENTED_EDGE('',*,*,#19242,.T.);
#25353=ORIENTED_EDGE('',*,*,#19247,.F.);
#25354=ORIENTED_EDGE('',*,*,#19248,.T.);
#25355=ORIENTED_EDGE('',*,*,#19249,.T.);
#25356=ORIENTED_EDGE('',*,*,#19248,.F.);
#25357=ORIENTED_EDGE('',*,*,#19250,.T.);
#25358=ORIENTED_EDGE('',*,*,#19249,.F.);
#25359=ORIENTED_EDGE('',*,*,#19251,.F.);
#25360=ORIENTED_EDGE('',*,*,#19252,.F.);
#25361=ORIENTED_EDGE('',*,*,#19251,.T.);
#25362=ORIENTED_EDGE('',*,*,#19250,.F.);
#25363=ORIENTED_EDGE('',*,*,#19253,.F.);
#25364=ORIENTED_EDGE('',*,*,#19254,.T.);
#25365=ORIENTED_EDGE('',*,*,#19255,.T.);
#25366=ORIENTED_EDGE('',*,*,#19256,.T.);
#25367=ORIENTED_EDGE('',*,*,#19254,.F.);
#25368=ORIENTED_EDGE('',*,*,#19252,.T.);
#25369=ORIENTED_EDGE('',*,*,#19255,.F.);
#25370=ORIENTED_EDGE('',*,*,#19256,.F.);
#25371=ORIENTED_EDGE('',*,*,#19257,.T.);
#25372=ORIENTED_EDGE('',*,*,#19258,.F.);
#25373=ORIENTED_EDGE('',*,*,#19259,.F.);
#25374=ORIENTED_EDGE('',*,*,#19257,.F.);
#25375=ORIENTED_EDGE('',*,*,#19260,.T.);
#25376=ORIENTED_EDGE('',*,*,#19261,.T.);
#25377=ORIENTED_EDGE('',*,*,#19260,.F.);
#25378=ORIENTED_EDGE('',*,*,#19258,.T.);
#25379=ORIENTED_EDGE('',*,*,#19259,.T.);
#25380=ORIENTED_EDGE('',*,*,#19261,.F.);
#25381=ORIENTED_EDGE('',*,*,#19262,.F.);
#25382=ORIENTED_EDGE('',*,*,#19263,.T.);
#25383=ORIENTED_EDGE('',*,*,#19264,.T.);
#25384=ORIENTED_EDGE('',*,*,#19262,.T.);
#25385=ORIENTED_EDGE('',*,*,#19265,.T.);
#25386=ORIENTED_EDGE('',*,*,#19266,.T.);
#25387=ORIENTED_EDGE('',*,*,#19267,.T.);
#25388=ORIENTED_EDGE('',*,*,#19268,.T.);
#25389=ORIENTED_EDGE('',*,*,#19269,.T.);
#25390=ORIENTED_EDGE('',*,*,#19267,.F.);
#25391=ORIENTED_EDGE('',*,*,#19269,.F.);
#25392=ORIENTED_EDGE('',*,*,#19270,.T.);
#25393=ORIENTED_EDGE('',*,*,#19271,.F.);
#25394=ORIENTED_EDGE('',*,*,#19272,.F.);
#25395=ORIENTED_EDGE('',*,*,#19270,.F.);
#25396=ORIENTED_EDGE('',*,*,#19268,.F.);
#25397=ORIENTED_EDGE('',*,*,#19263,.F.);
#25398=ORIENTED_EDGE('',*,*,#19264,.F.);
#25399=ORIENTED_EDGE('',*,*,#19273,.T.);
#25400=ORIENTED_EDGE('',*,*,#19265,.F.);
#25401=ORIENTED_EDGE('',*,*,#19266,.F.);
#25402=ORIENTED_EDGE('',*,*,#19273,.F.);
#25403=ORIENTED_EDGE('',*,*,#19271,.T.);
#25404=ORIENTED_EDGE('',*,*,#19272,.T.);
#25405=ORIENTED_EDGE('',*,*,#19274,.T.);
#25406=ORIENTED_EDGE('',*,*,#19275,.T.);
#25407=ORIENTED_EDGE('',*,*,#19274,.F.);
#25408=ORIENTED_EDGE('',*,*,#19275,.F.);
#25409=ORIENTED_EDGE('',*,*,#19276,.T.);
#25410=ORIENTED_EDGE('',*,*,#19277,.T.);
#25411=ORIENTED_EDGE('',*,*,#19278,.T.);
#25412=ORIENTED_EDGE('',*,*,#19279,.T.);
#25413=ORIENTED_EDGE('',*,*,#19280,.T.);
#25414=ORIENTED_EDGE('',*,*,#19279,.F.);
#25415=ORIENTED_EDGE('',*,*,#19280,.F.);
#25416=ORIENTED_EDGE('',*,*,#19281,.T.);
#25417=ORIENTED_EDGE('',*,*,#19276,.F.);
#25418=ORIENTED_EDGE('',*,*,#19282,.T.);
#25419=ORIENTED_EDGE('',*,*,#19277,.F.);
#25420=ORIENTED_EDGE('',*,*,#19278,.F.);
#25421=ORIENTED_EDGE('',*,*,#19282,.F.);
#25422=ORIENTED_EDGE('',*,*,#19283,.T.);
#25423=ORIENTED_EDGE('',*,*,#19284,.T.);
#25424=ORIENTED_EDGE('',*,*,#19285,.T.);
#25425=ORIENTED_EDGE('',*,*,#19286,.T.);
#25426=ORIENTED_EDGE('',*,*,#19285,.F.);
#25427=ORIENTED_EDGE('',*,*,#19286,.F.);
#25428=ORIENTED_EDGE('',*,*,#19287,.F.);
#25429=ORIENTED_EDGE('',*,*,#19288,.T.);
#25430=ORIENTED_EDGE('',*,*,#19289,.F.);
#25431=ORIENTED_EDGE('',*,*,#19290,.T.);
#25432=ORIENTED_EDGE('',*,*,#19291,.F.);
#25433=ORIENTED_EDGE('',*,*,#19292,.T.);
#25434=ORIENTED_EDGE('',*,*,#19293,.F.);
#25435=ORIENTED_EDGE('',*,*,#19294,.T.);
#25436=ORIENTED_EDGE('',*,*,#19295,.F.);
#25437=ORIENTED_EDGE('',*,*,#19296,.T.);
#25438=ORIENTED_EDGE('',*,*,#19297,.F.);
#25439=ORIENTED_EDGE('',*,*,#19298,.T.);
#25440=ORIENTED_EDGE('',*,*,#19299,.F.);
#25441=ORIENTED_EDGE('',*,*,#19300,.T.);
#25442=ORIENTED_EDGE('',*,*,#19301,.F.);
#25443=ORIENTED_EDGE('',*,*,#19302,.T.);
#25444=ORIENTED_EDGE('',*,*,#19303,.F.);
#25445=ORIENTED_EDGE('',*,*,#19304,.T.);
#25446=ORIENTED_EDGE('',*,*,#19305,.F.);
#25447=ORIENTED_EDGE('',*,*,#19306,.T.);
#25448=ORIENTED_EDGE('',*,*,#19307,.F.);
#25449=ORIENTED_EDGE('',*,*,#19308,.T.);
#25450=ORIENTED_EDGE('',*,*,#19309,.F.);
#25451=ORIENTED_EDGE('',*,*,#19310,.T.);
#25452=ORIENTED_EDGE('',*,*,#19311,.F.);
#25453=ORIENTED_EDGE('',*,*,#19312,.T.);
#25454=ORIENTED_EDGE('',*,*,#19313,.F.);
#25455=ORIENTED_EDGE('',*,*,#19314,.T.);
#25456=ORIENTED_EDGE('',*,*,#19315,.F.);
#25457=ORIENTED_EDGE('',*,*,#19316,.T.);
#25458=ORIENTED_EDGE('',*,*,#19317,.F.);
#25459=ORIENTED_EDGE('',*,*,#19318,.T.);
#25460=ORIENTED_EDGE('',*,*,#19319,.F.);
#25461=ORIENTED_EDGE('',*,*,#19320,.T.);
#25462=ORIENTED_EDGE('',*,*,#19321,.F.);
#25463=ORIENTED_EDGE('',*,*,#19322,.T.);
#25464=ORIENTED_EDGE('',*,*,#19323,.F.);
#25465=ORIENTED_EDGE('',*,*,#19324,.T.);
#25466=ORIENTED_EDGE('',*,*,#19325,.F.);
#25467=ORIENTED_EDGE('',*,*,#19326,.T.);
#25468=ORIENTED_EDGE('',*,*,#19327,.F.);
#25469=ORIENTED_EDGE('',*,*,#19328,.T.);
#25470=ORIENTED_EDGE('',*,*,#19329,.F.);
#25471=ORIENTED_EDGE('',*,*,#19330,.T.);
#25472=ORIENTED_EDGE('',*,*,#19331,.F.);
#25473=ORIENTED_EDGE('',*,*,#19332,.T.);
#25474=ORIENTED_EDGE('',*,*,#19333,.F.);
#25475=ORIENTED_EDGE('',*,*,#19334,.T.);
#25476=ORIENTED_EDGE('',*,*,#19335,.F.);
#25477=ORIENTED_EDGE('',*,*,#19336,.T.);
#25478=ORIENTED_EDGE('',*,*,#19337,.F.);
#25479=ORIENTED_EDGE('',*,*,#19338,.T.);
#25480=ORIENTED_EDGE('',*,*,#19339,.F.);
#25481=ORIENTED_EDGE('',*,*,#19340,.F.);
#25482=ORIENTED_EDGE('',*,*,#19281,.F.);
#25483=ORIENTED_EDGE('',*,*,#19341,.T.);
#25484=ORIENTED_EDGE('',*,*,#19283,.F.);
#25485=ORIENTED_EDGE('',*,*,#19284,.F.);
#25486=ORIENTED_EDGE('',*,*,#19341,.F.);
#25487=ORIENTED_EDGE('',*,*,#19342,.F.);
#25488=ORIENTED_EDGE('',*,*,#19343,.T.);
#25489=ORIENTED_EDGE('',*,*,#19344,.T.);
#25490=ORIENTED_EDGE('',*,*,#19345,.T.);
#25491=ORIENTED_EDGE('',*,*,#19346,.T.);
#25492=ORIENTED_EDGE('',*,*,#19347,.F.);
#25493=ORIENTED_EDGE('',*,*,#19346,.F.);
#25494=ORIENTED_EDGE('',*,*,#19348,.F.);
#25495=ORIENTED_EDGE('',*,*,#19349,.T.);
#25496=ORIENTED_EDGE('',*,*,#19350,.T.);
#25497=ORIENTED_EDGE('',*,*,#19351,.T.);
#25498=ORIENTED_EDGE('',*,*,#19352,.T.);
#25499=ORIENTED_EDGE('',*,*,#19353,.T.);
#25500=ORIENTED_EDGE('',*,*,#19354,.T.);
#25501=ORIENTED_EDGE('',*,*,#19355,.T.);
#25502=ORIENTED_EDGE('',*,*,#19356,.T.);
#25503=ORIENTED_EDGE('',*,*,#19357,.T.);
#25504=ORIENTED_EDGE('',*,*,#19354,.F.);
#25505=ORIENTED_EDGE('',*,*,#19358,.F.);
#25506=ORIENTED_EDGE('',*,*,#19356,.F.);
#25507=ORIENTED_EDGE('',*,*,#19359,.T.);
#25508=ORIENTED_EDGE('',*,*,#19360,.T.);
#25509=ORIENTED_EDGE('',*,*,#19361,.T.);
#25510=ORIENTED_EDGE('',*,*,#19360,.F.);
#25511=ORIENTED_EDGE('',*,*,#19362,.T.);
#25512=ORIENTED_EDGE('',*,*,#19363,.T.);
#25513=ORIENTED_EDGE('',*,*,#19359,.F.);
#25514=ORIENTED_EDGE('',*,*,#19355,.F.);
#25515=ORIENTED_EDGE('',*,*,#19358,.T.);
#25516=ORIENTED_EDGE('',*,*,#19353,.F.);
#25517=ORIENTED_EDGE('',*,*,#19364,.T.);
#25518=ORIENTED_EDGE('',*,*,#19351,.F.);
#25519=ORIENTED_EDGE('',*,*,#19365,.T.);
#25520=ORIENTED_EDGE('',*,*,#19366,.F.);
#25521=ORIENTED_EDGE('',*,*,#19367,.F.);
#25522=ORIENTED_EDGE('',*,*,#19368,.F.);
#25523=ORIENTED_EDGE('',*,*,#19352,.F.);
#25524=ORIENTED_EDGE('',*,*,#19364,.F.);
#25525=ORIENTED_EDGE('',*,*,#19369,.T.);
#25526=ORIENTED_EDGE('',*,*,#19370,.T.);
#25527=ORIENTED_EDGE('',*,*,#19371,.T.);
#25528=ORIENTED_EDGE('',*,*,#19372,.T.);
#25529=ORIENTED_EDGE('',*,*,#19373,.T.);
#25530=ORIENTED_EDGE('',*,*,#19374,.T.);
#25531=ORIENTED_EDGE('',*,*,#19371,.F.);
#25532=ORIENTED_EDGE('',*,*,#19369,.F.);
#25533=ORIENTED_EDGE('',*,*,#19375,.T.);
#25534=ORIENTED_EDGE('',*,*,#19376,.T.);
#25535=ORIENTED_EDGE('',*,*,#19374,.F.);
#25536=ORIENTED_EDGE('',*,*,#19377,.T.);
#25537=ORIENTED_EDGE('',*,*,#19378,.T.);
#25538=ORIENTED_EDGE('',*,*,#19379,.T.);
#25539=ORIENTED_EDGE('',*,*,#19373,.F.);
#25540=ORIENTED_EDGE('',*,*,#19380,.T.);
#25541=ORIENTED_EDGE('',*,*,#19381,.F.);
#25542=ORIENTED_EDGE('',*,*,#19382,.T.);
#25543=ORIENTED_EDGE('',*,*,#19370,.F.);
#25544=ORIENTED_EDGE('',*,*,#19383,.F.);
#25545=ORIENTED_EDGE('',*,*,#19384,.F.);
#25546=ORIENTED_EDGE('',*,*,#19380,.F.);
#25547=ORIENTED_EDGE('',*,*,#19385,.T.);
#25548=ORIENTED_EDGE('',*,*,#19386,.T.);
#25549=ORIENTED_EDGE('',*,*,#19387,.T.);
#25550=ORIENTED_EDGE('',*,*,#19388,.T.);
#25551=ORIENTED_EDGE('',*,*,#19367,.T.);
#25552=ORIENTED_EDGE('',*,*,#19389,.T.);
#25553=ORIENTED_EDGE('',*,*,#19385,.F.);
#25554=ORIENTED_EDGE('',*,*,#19366,.T.);
#25555=ORIENTED_EDGE('',*,*,#19365,.F.);
#25556=ORIENTED_EDGE('',*,*,#19350,.F.);
#25557=ORIENTED_EDGE('',*,*,#19390,.F.);
#25558=ORIENTED_EDGE('',*,*,#19387,.F.);
#25559=ORIENTED_EDGE('',*,*,#19391,.T.);
#25560=ORIENTED_EDGE('',*,*,#19392,.T.);
#25561=ORIENTED_EDGE('',*,*,#19388,.F.);
#25562=ORIENTED_EDGE('',*,*,#19393,.T.);
#25563=ORIENTED_EDGE('',*,*,#19393,.F.);
#25564=ORIENTED_EDGE('',*,*,#19394,.T.);
#25565=ORIENTED_EDGE('',*,*,#19395,.T.);
#25566=ORIENTED_EDGE('',*,*,#19389,.F.);
#25567=ORIENTED_EDGE('',*,*,#19390,.T.);
#25568=ORIENTED_EDGE('',*,*,#19349,.F.);
#25569=ORIENTED_EDGE('',*,*,#19357,.F.);
#25570=ORIENTED_EDGE('',*,*,#19396,.T.);
#25571=ORIENTED_EDGE('',*,*,#19397,.F.);
#25572=ORIENTED_EDGE('',*,*,#19398,.T.);
#25573=ORIENTED_EDGE('',*,*,#19399,.F.);
#25574=ORIENTED_EDGE('',*,*,#19400,.F.);
#25575=ORIENTED_EDGE('',*,*,#19401,.T.);
#25576=ORIENTED_EDGE('',*,*,#19402,.F.);
#25577=ORIENTED_EDGE('',*,*,#19403,.T.);
#25578=ORIENTED_EDGE('',*,*,#19343,.F.);
#25579=ORIENTED_EDGE('',*,*,#19404,.T.);
#25580=ORIENTED_EDGE('',*,*,#19405,.F.);
#25581=ORIENTED_EDGE('',*,*,#19406,.T.);
#25582=ORIENTED_EDGE('',*,*,#19407,.F.);
#25583=ORIENTED_EDGE('',*,*,#19408,.F.);
#25584=ORIENTED_EDGE('',*,*,#19409,.T.);
#25585=ORIENTED_EDGE('',*,*,#19410,.F.);
#25586=ORIENTED_EDGE('',*,*,#19411,.T.);
#25587=ORIENTED_EDGE('',*,*,#19412,.F.);
#25588=ORIENTED_EDGE('',*,*,#19413,.T.);
#25589=ORIENTED_EDGE('',*,*,#19414,.F.);
#25590=ORIENTED_EDGE('',*,*,#19415,.F.);
#25591=ORIENTED_EDGE('',*,*,#19384,.T.);
#25592=ORIENTED_EDGE('',*,*,#19416,.F.);
#25593=ORIENTED_EDGE('',*,*,#19417,.F.);
#25594=ORIENTED_EDGE('',*,*,#19418,.F.);
#25595=ORIENTED_EDGE('',*,*,#19419,.T.);
#25596=ORIENTED_EDGE('',*,*,#19394,.F.);
#25597=ORIENTED_EDGE('',*,*,#19417,.T.);
#25598=ORIENTED_EDGE('',*,*,#19420,.T.);
#25599=ORIENTED_EDGE('',*,*,#19421,.T.);
#25600=ORIENTED_EDGE('',*,*,#19422,.T.);
#25601=ORIENTED_EDGE('',*,*,#19423,.T.);
#25602=ORIENTED_EDGE('',*,*,#19424,.T.);
#25603=ORIENTED_EDGE('',*,*,#19375,.F.);
#25604=ORIENTED_EDGE('',*,*,#19425,.T.);
#25605=ORIENTED_EDGE('',*,*,#19426,.T.);
#25606=ORIENTED_EDGE('',*,*,#19427,.T.);
#25607=ORIENTED_EDGE('',*,*,#19376,.F.);
#25608=ORIENTED_EDGE('',*,*,#19428,.T.);
#25609=ORIENTED_EDGE('',*,*,#19429,.T.);
#25610=ORIENTED_EDGE('',*,*,#19383,.T.);
#25611=ORIENTED_EDGE('',*,*,#19416,.T.);
#25612=ORIENTED_EDGE('',*,*,#19429,.F.);
#25613=ORIENTED_EDGE('',*,*,#19430,.T.);
#25614=ORIENTED_EDGE('',*,*,#19431,.F.);
#25615=ORIENTED_EDGE('',*,*,#19420,.F.);
#25616=ORIENTED_EDGE('',*,*,#19432,.T.);
#25617=ORIENTED_EDGE('',*,*,#19433,.T.);
#25618=ORIENTED_EDGE('',*,*,#19418,.T.);
#25619=ORIENTED_EDGE('',*,*,#19424,.F.);
#25620=ORIENTED_EDGE('',*,*,#19434,.F.);
#25621=ORIENTED_EDGE('',*,*,#19433,.F.);
#25622=ORIENTED_EDGE('',*,*,#19435,.T.);
#25623=ORIENTED_EDGE('',*,*,#19436,.T.);
#25624=ORIENTED_EDGE('',*,*,#19437,.T.);
#25625=ORIENTED_EDGE('',*,*,#19438,.T.);
#25626=ORIENTED_EDGE('',*,*,#19426,.F.);
#25627=ORIENTED_EDGE('',*,*,#19439,.T.);
#25628=ORIENTED_EDGE('',*,*,#19437,.F.);
#25629=ORIENTED_EDGE('',*,*,#19440,.T.);
#25630=ORIENTED_EDGE('',*,*,#19440,.F.);
#25631=ORIENTED_EDGE('',*,*,#19436,.F.);
#25632=ORIENTED_EDGE('',*,*,#19386,.F.);
#25633=ORIENTED_EDGE('',*,*,#19395,.F.);
#25634=ORIENTED_EDGE('',*,*,#19419,.F.);
#25635=ORIENTED_EDGE('',*,*,#19438,.F.);
#25636=ORIENTED_EDGE('',*,*,#19441,.F.);
#25637=ORIENTED_EDGE('',*,*,#19391,.F.);
#25638=ORIENTED_EDGE('',*,*,#19441,.T.);
#25639=ORIENTED_EDGE('',*,*,#19439,.F.);
#25640=ORIENTED_EDGE('',*,*,#19442,.T.);
#25641=ORIENTED_EDGE('',*,*,#19443,.F.);
#25642=ORIENTED_EDGE('',*,*,#19372,.F.);
#25643=ORIENTED_EDGE('',*,*,#19379,.F.);
#25644=ORIENTED_EDGE('',*,*,#19444,.F.);
#25645=ORIENTED_EDGE('',*,*,#19445,.F.);
#25646=ORIENTED_EDGE('',*,*,#19446,.F.);
#25647=ORIENTED_EDGE('',*,*,#19447,.F.);
#25648=ORIENTED_EDGE('',*,*,#19448,.F.);
#25649=ORIENTED_EDGE('',*,*,#19449,.F.);
#25650=ORIENTED_EDGE('',*,*,#19450,.F.);
#25651=ORIENTED_EDGE('',*,*,#19451,.F.);
#25652=ORIENTED_EDGE('',*,*,#19442,.F.);
#25653=ORIENTED_EDGE('',*,*,#19425,.F.);
#25654=ORIENTED_EDGE('',*,*,#19430,.F.);
#25655=ORIENTED_EDGE('',*,*,#19428,.F.);
#25656=ORIENTED_EDGE('',*,*,#19427,.F.);
#25657=ORIENTED_EDGE('',*,*,#19435,.F.);
#25658=ORIENTED_EDGE('',*,*,#19432,.F.);
#25659=ORIENTED_EDGE('',*,*,#19434,.T.);
#25660=ORIENTED_EDGE('',*,*,#19423,.F.);
#25661=ORIENTED_EDGE('',*,*,#19452,.T.);
#25662=ORIENTED_EDGE('',*,*,#19421,.F.);
#25663=ORIENTED_EDGE('',*,*,#19431,.T.);
#25664=ORIENTED_EDGE('',*,*,#19414,.T.);
#25665=ORIENTED_EDGE('',*,*,#19453,.T.);
#25666=ORIENTED_EDGE('',*,*,#19454,.T.);
#25667=ORIENTED_EDGE('',*,*,#19455,.T.);
#25668=ORIENTED_EDGE('',*,*,#19456,.T.);
#25669=ORIENTED_EDGE('',*,*,#19457,.T.);
#25670=ORIENTED_EDGE('',*,*,#19458,.T.);
#25671=ORIENTED_EDGE('',*,*,#19381,.T.);
#25672=ORIENTED_EDGE('',*,*,#19415,.T.);
#25673=ORIENTED_EDGE('',*,*,#19457,.F.);
#25674=ORIENTED_EDGE('',*,*,#19459,.F.);
#25675=ORIENTED_EDGE('',*,*,#19378,.F.);
#25676=ORIENTED_EDGE('',*,*,#19460,.T.);
#25677=ORIENTED_EDGE('',*,*,#19461,.T.);
#25678=ORIENTED_EDGE('',*,*,#19461,.F.);
#25679=ORIENTED_EDGE('',*,*,#19462,.T.);
#25680=ORIENTED_EDGE('',*,*,#19463,.T.);
#25681=ORIENTED_EDGE('',*,*,#19444,.T.);
#25682=ORIENTED_EDGE('',*,*,#19460,.F.);
#25683=ORIENTED_EDGE('',*,*,#19464,.T.);
#25684=ORIENTED_EDGE('',*,*,#19465,.T.);
#25685=ORIENTED_EDGE('',*,*,#19466,.T.);
#25686=ORIENTED_EDGE('',*,*,#19412,.T.);
#25687=ORIENTED_EDGE('',*,*,#19465,.F.);
#25688=ORIENTED_EDGE('',*,*,#19467,.T.);
#25689=ORIENTED_EDGE('',*,*,#19468,.F.);
#25690=ORIENTED_EDGE('',*,*,#19453,.F.);
#25691=ORIENTED_EDGE('',*,*,#19413,.F.);
#25692=ORIENTED_EDGE('',*,*,#19469,.T.);
#25693=ORIENTED_EDGE('',*,*,#19470,.T.);
#25694=ORIENTED_EDGE('',*,*,#19471,.T.);
#25695=ORIENTED_EDGE('',*,*,#19472,.T.);
#25696=ORIENTED_EDGE('',*,*,#19473,.T.);
#25697=ORIENTED_EDGE('',*,*,#19474,.T.);
#25698=ORIENTED_EDGE('',*,*,#19471,.F.);
#25699=ORIENTED_EDGE('',*,*,#19410,.T.);
#25700=ORIENTED_EDGE('',*,*,#19469,.F.);
#25701=ORIENTED_EDGE('',*,*,#19475,.T.);
#25702=ORIENTED_EDGE('',*,*,#19463,.F.);
#25703=ORIENTED_EDGE('',*,*,#19458,.F.);
#25704=ORIENTED_EDGE('',*,*,#19459,.T.);
#25705=ORIENTED_EDGE('',*,*,#19456,.F.);
#25706=ORIENTED_EDGE('',*,*,#19476,.T.);
#25707=ORIENTED_EDGE('',*,*,#19454,.F.);
#25708=ORIENTED_EDGE('',*,*,#19468,.T.);
#25709=ORIENTED_EDGE('',*,*,#19467,.F.);
#25710=ORIENTED_EDGE('',*,*,#19464,.F.);
#25711=ORIENTED_EDGE('',*,*,#19377,.F.);
#25712=ORIENTED_EDGE('',*,*,#19382,.F.);
#25713=ORIENTED_EDGE('',*,*,#19475,.F.);
#25714=ORIENTED_EDGE('',*,*,#19477,.T.);
#25715=ORIENTED_EDGE('',*,*,#19478,.F.);
#25716=ORIENTED_EDGE('',*,*,#19445,.T.);
#25717=ORIENTED_EDGE('',*,*,#19479,.T.);
#25718=ORIENTED_EDGE('',*,*,#19480,.T.);
#25719=ORIENTED_EDGE('',*,*,#19481,.T.);
#25720=ORIENTED_EDGE('',*,*,#19482,.T.);
#25721=ORIENTED_EDGE('',*,*,#19483,.T.);
#25722=ORIENTED_EDGE('',*,*,#19479,.F.);
#25723=ORIENTED_EDGE('',*,*,#19484,.T.);
#25724=ORIENTED_EDGE('',*,*,#19485,.T.);
#25725=ORIENTED_EDGE('',*,*,#19480,.F.);
#25726=ORIENTED_EDGE('',*,*,#19486,.F.);
#25727=ORIENTED_EDGE('',*,*,#19486,.T.);
#25728=ORIENTED_EDGE('',*,*,#19487,.T.);
#25729=ORIENTED_EDGE('',*,*,#19482,.F.);
#25730=ORIENTED_EDGE('',*,*,#19405,.T.);
#25731=ORIENTED_EDGE('',*,*,#19404,.F.);
#25732=ORIENTED_EDGE('',*,*,#19342,.T.);
#25733=ORIENTED_EDGE('',*,*,#19488,.T.);
#25734=ORIENTED_EDGE('',*,*,#19481,.F.);
#25735=ORIENTED_EDGE('',*,*,#19489,.F.);
#25736=ORIENTED_EDGE('',*,*,#19490,.F.);
#25737=ORIENTED_EDGE('',*,*,#19406,.F.);
#25738=ORIENTED_EDGE('',*,*,#19491,.T.);
#25739=ORIENTED_EDGE('',*,*,#19492,.T.);
#25740=ORIENTED_EDGE('',*,*,#19493,.T.);
#25741=ORIENTED_EDGE('',*,*,#19494,.T.);
#25742=ORIENTED_EDGE('',*,*,#19495,.T.);
#25743=ORIENTED_EDGE('',*,*,#19491,.F.);
#25744=ORIENTED_EDGE('',*,*,#19496,.T.);
#25745=ORIENTED_EDGE('',*,*,#19402,.T.);
#25746=ORIENTED_EDGE('',*,*,#19494,.F.);
#25747=ORIENTED_EDGE('',*,*,#19497,.T.);
#25748=ORIENTED_EDGE('',*,*,#19498,.F.);
#25749=ORIENTED_EDGE('',*,*,#19344,.F.);
#25750=ORIENTED_EDGE('',*,*,#19403,.F.);
#25751=ORIENTED_EDGE('',*,*,#19487,.F.);
#25752=ORIENTED_EDGE('',*,*,#19488,.F.);
#25753=ORIENTED_EDGE('',*,*,#19347,.T.);
#25754=ORIENTED_EDGE('',*,*,#19348,.T.);
#25755=ORIENTED_EDGE('',*,*,#19345,.F.);
#25756=ORIENTED_EDGE('',*,*,#19498,.T.);
#25757=ORIENTED_EDGE('',*,*,#19497,.F.);
#25758=ORIENTED_EDGE('',*,*,#19496,.F.);
#25759=ORIENTED_EDGE('',*,*,#19499,.F.);
#25760=ORIENTED_EDGE('',*,*,#19483,.F.);
#25761=ORIENTED_EDGE('',*,*,#19484,.F.);
#25762=ORIENTED_EDGE('',*,*,#19499,.T.);
#25763=ORIENTED_EDGE('',*,*,#19493,.F.);
#25764=ORIENTED_EDGE('',*,*,#19447,.T.);
#25765=ORIENTED_EDGE('',*,*,#19492,.F.);
#25766=ORIENTED_EDGE('',*,*,#19500,.T.);
#25767=ORIENTED_EDGE('',*,*,#19501,.F.);
#25768=ORIENTED_EDGE('',*,*,#19448,.T.);
#25769=ORIENTED_EDGE('',*,*,#19399,.T.);
#25770=ORIENTED_EDGE('',*,*,#19502,.T.);
#25771=ORIENTED_EDGE('',*,*,#19503,.T.);
#25772=ORIENTED_EDGE('',*,*,#19504,.T.);
#25773=ORIENTED_EDGE('',*,*,#19505,.T.);
#25774=ORIENTED_EDGE('',*,*,#19506,.T.);
#25775=ORIENTED_EDGE('',*,*,#19507,.T.);
#25776=ORIENTED_EDGE('',*,*,#19508,.T.);
#25777=ORIENTED_EDGE('',*,*,#19400,.T.);
#25778=ORIENTED_EDGE('',*,*,#19506,.F.);
#25779=ORIENTED_EDGE('',*,*,#19509,.F.);
#25780=ORIENTED_EDGE('',*,*,#19508,.F.);
#25781=ORIENTED_EDGE('',*,*,#19510,.T.);
#25782=ORIENTED_EDGE('',*,*,#19511,.T.);
#25783=ORIENTED_EDGE('',*,*,#19512,.T.);
#25784=ORIENTED_EDGE('',*,*,#19511,.F.);
#25785=ORIENTED_EDGE('',*,*,#19513,.T.);
#25786=ORIENTED_EDGE('',*,*,#19501,.T.);
#25787=ORIENTED_EDGE('',*,*,#19510,.F.);
#25788=ORIENTED_EDGE('',*,*,#19507,.F.);
#25789=ORIENTED_EDGE('',*,*,#19509,.T.);
#25790=ORIENTED_EDGE('',*,*,#19505,.F.);
#25791=ORIENTED_EDGE('',*,*,#19514,.T.);
#25792=ORIENTED_EDGE('',*,*,#19503,.F.);
#25793=ORIENTED_EDGE('',*,*,#19515,.T.);
#25794=ORIENTED_EDGE('',*,*,#19516,.F.);
#25795=ORIENTED_EDGE('',*,*,#19517,.F.);
#25796=ORIENTED_EDGE('',*,*,#19518,.F.);
#25797=ORIENTED_EDGE('',*,*,#19504,.F.);
#25798=ORIENTED_EDGE('',*,*,#19514,.F.);
#25799=ORIENTED_EDGE('',*,*,#19519,.T.);
#25800=ORIENTED_EDGE('',*,*,#19520,.T.);
#25801=ORIENTED_EDGE('',*,*,#19521,.T.);
#25802=ORIENTED_EDGE('',*,*,#19517,.T.);
#25803=ORIENTED_EDGE('',*,*,#19397,.T.);
#25804=ORIENTED_EDGE('',*,*,#19519,.F.);
#25805=ORIENTED_EDGE('',*,*,#19516,.T.);
#25806=ORIENTED_EDGE('',*,*,#19515,.F.);
#25807=ORIENTED_EDGE('',*,*,#19502,.F.);
#25808=ORIENTED_EDGE('',*,*,#19398,.F.);
#25809=ORIENTED_EDGE('',*,*,#19521,.F.);
#25810=ORIENTED_EDGE('',*,*,#19522,.T.);
#25811=ORIENTED_EDGE('',*,*,#19523,.T.);
#25812=ORIENTED_EDGE('',*,*,#19362,.F.);
#25813=ORIENTED_EDGE('',*,*,#19368,.T.);
#25814=ORIENTED_EDGE('',*,*,#19392,.F.);
#25815=ORIENTED_EDGE('',*,*,#19451,.T.);
#25816=ORIENTED_EDGE('',*,*,#19363,.F.);
#25817=ORIENTED_EDGE('',*,*,#19450,.T.);
#25818=ORIENTED_EDGE('',*,*,#19522,.F.);
#25819=ORIENTED_EDGE('',*,*,#19524,.T.);
#25820=ORIENTED_EDGE('',*,*,#19513,.F.);
#25821=ORIENTED_EDGE('',*,*,#19518,.T.);
#25822=ORIENTED_EDGE('',*,*,#19523,.F.);
#25823=ORIENTED_EDGE('',*,*,#19449,.T.);
#25824=ORIENTED_EDGE('',*,*,#19525,.T.);
#25825=ORIENTED_EDGE('',*,*,#19478,.T.);
#25826=ORIENTED_EDGE('',*,*,#19526,.T.);
#25827=ORIENTED_EDGE('',*,*,#19527,.F.);
#25828=ORIENTED_EDGE('',*,*,#19527,.T.);
#25829=ORIENTED_EDGE('',*,*,#19528,.T.);
#25830=ORIENTED_EDGE('',*,*,#19485,.F.);
#25831=ORIENTED_EDGE('',*,*,#19446,.T.);
#25832=ORIENTED_EDGE('',*,*,#19525,.F.);
#25833=ORIENTED_EDGE('',*,*,#19489,.T.);
#25834=ORIENTED_EDGE('',*,*,#19361,.F.);
#25835=ORIENTED_EDGE('',*,*,#19524,.F.);
#25836=ORIENTED_EDGE('',*,*,#19520,.F.);
#25837=ORIENTED_EDGE('',*,*,#19396,.F.);
#25838=ORIENTED_EDGE('',*,*,#19495,.F.);
#25839=ORIENTED_EDGE('',*,*,#19401,.F.);
#25840=ORIENTED_EDGE('',*,*,#19512,.F.);
#25841=ORIENTED_EDGE('',*,*,#19500,.F.);
#25842=ORIENTED_EDGE('',*,*,#19526,.F.);
#25843=ORIENTED_EDGE('',*,*,#19529,.T.);
#25844=ORIENTED_EDGE('',*,*,#19530,.T.);
#25845=ORIENTED_EDGE('',*,*,#19490,.T.);
#25846=ORIENTED_EDGE('',*,*,#19528,.F.);
#25847=ORIENTED_EDGE('',*,*,#19443,.T.);
#25848=ORIENTED_EDGE('',*,*,#19531,.T.);
#25849=ORIENTED_EDGE('',*,*,#19532,.T.);
#25850=ORIENTED_EDGE('',*,*,#19533,.T.);
#25851=ORIENTED_EDGE('',*,*,#19531,.F.);
#25852=ORIENTED_EDGE('',*,*,#19533,.F.);
#25853=ORIENTED_EDGE('',*,*,#19534,.T.);
#25854=ORIENTED_EDGE('',*,*,#19253,.T.);
#25855=ORIENTED_EDGE('',*,*,#19534,.F.);
#25856=ORIENTED_EDGE('',*,*,#19532,.F.);
#25857=ORIENTED_EDGE('',*,*,#19535,.T.);
#25858=ORIENTED_EDGE('',*,*,#19536,.T.);
#25859=ORIENTED_EDGE('',*,*,#19473,.F.);
#25860=ORIENTED_EDGE('',*,*,#19409,.F.);
#25861=ORIENTED_EDGE('',*,*,#19408,.T.);
#25862=ORIENTED_EDGE('',*,*,#19537,.T.);
#25863=ORIENTED_EDGE('',*,*,#19538,.T.);
#25864=ORIENTED_EDGE('',*,*,#19407,.T.);
#25865=ORIENTED_EDGE('',*,*,#19530,.F.);
#25866=ORIENTED_EDGE('',*,*,#19539,.T.);
#25867=ORIENTED_EDGE('',*,*,#19540,.F.);
#25868=ORIENTED_EDGE('',*,*,#19537,.F.);
#25869=ORIENTED_EDGE('',*,*,#19288,.F.);
#25870=ORIENTED_EDGE('',*,*,#19541,.F.);
#25871=ORIENTED_EDGE('',*,*,#19542,.T.);
#25872=ORIENTED_EDGE('',*,*,#19543,.T.);
#25873=ORIENTED_EDGE('',*,*,#19542,.F.);
#25874=ORIENTED_EDGE('',*,*,#19544,.T.);
#25875=ORIENTED_EDGE('',*,*,#19545,.F.);
#25876=ORIENTED_EDGE('',*,*,#19546,.T.);
#25877=ORIENTED_EDGE('',*,*,#19547,.F.);
#25878=ORIENTED_EDGE('',*,*,#19548,.T.);
#25879=ORIENTED_EDGE('',*,*,#19549,.F.);
#25880=ORIENTED_EDGE('',*,*,#19550,.T.);
#25881=ORIENTED_EDGE('',*,*,#19551,.F.);
#25882=ORIENTED_EDGE('',*,*,#19552,.T.);
#25883=ORIENTED_EDGE('',*,*,#19553,.F.);
#25884=ORIENTED_EDGE('',*,*,#19554,.T.);
#25885=ORIENTED_EDGE('',*,*,#19555,.F.);
#25886=ORIENTED_EDGE('',*,*,#19556,.T.);
#25887=ORIENTED_EDGE('',*,*,#19557,.F.);
#25888=ORIENTED_EDGE('',*,*,#19558,.T.);
#25889=ORIENTED_EDGE('',*,*,#19559,.F.);
#25890=ORIENTED_EDGE('',*,*,#19560,.T.);
#25891=ORIENTED_EDGE('',*,*,#19561,.F.);
#25892=ORIENTED_EDGE('',*,*,#19562,.T.);
#25893=ORIENTED_EDGE('',*,*,#19563,.F.);
#25894=ORIENTED_EDGE('',*,*,#19564,.T.);
#25895=ORIENTED_EDGE('',*,*,#19565,.F.);
#25896=ORIENTED_EDGE('',*,*,#19566,.T.);
#25897=ORIENTED_EDGE('',*,*,#19567,.F.);
#25898=ORIENTED_EDGE('',*,*,#19568,.T.);
#25899=ORIENTED_EDGE('',*,*,#19569,.F.);
#25900=ORIENTED_EDGE('',*,*,#19570,.T.);
#25901=ORIENTED_EDGE('',*,*,#19571,.F.);
#25902=ORIENTED_EDGE('',*,*,#19572,.T.);
#25903=ORIENTED_EDGE('',*,*,#19573,.F.);
#25904=ORIENTED_EDGE('',*,*,#19574,.T.);
#25905=ORIENTED_EDGE('',*,*,#19575,.F.);
#25906=ORIENTED_EDGE('',*,*,#19576,.T.);
#25907=ORIENTED_EDGE('',*,*,#19577,.F.);
#25908=ORIENTED_EDGE('',*,*,#19578,.T.);
#25909=ORIENTED_EDGE('',*,*,#19579,.F.);
#25910=ORIENTED_EDGE('',*,*,#19580,.T.);
#25911=ORIENTED_EDGE('',*,*,#19581,.F.);
#25912=ORIENTED_EDGE('',*,*,#19582,.T.);
#25913=ORIENTED_EDGE('',*,*,#19583,.F.);
#25914=ORIENTED_EDGE('',*,*,#19584,.T.);
#25915=ORIENTED_EDGE('',*,*,#19585,.F.);
#25916=ORIENTED_EDGE('',*,*,#19586,.T.);
#25917=ORIENTED_EDGE('',*,*,#19587,.F.);
#25918=ORIENTED_EDGE('',*,*,#19588,.T.);
#25919=ORIENTED_EDGE('',*,*,#19589,.F.);
#25920=ORIENTED_EDGE('',*,*,#19590,.T.);
#25921=ORIENTED_EDGE('',*,*,#19591,.F.);
#25922=ORIENTED_EDGE('',*,*,#19592,.T.);
#25923=ORIENTED_EDGE('',*,*,#19593,.F.);
#25924=ORIENTED_EDGE('',*,*,#19594,.T.);
#25925=ORIENTED_EDGE('',*,*,#19595,.F.);
#25926=ORIENTED_EDGE('',*,*,#19596,.T.);
#25927=ORIENTED_EDGE('',*,*,#19160,.T.);
#25928=ORIENTED_EDGE('',*,*,#19597,.T.);
#25929=ORIENTED_EDGE('',*,*,#19598,.T.);
#25930=ORIENTED_EDGE('',*,*,#19165,.T.);
#25931=ORIENTED_EDGE('',*,*,#19599,.T.);
#25932=ORIENTED_EDGE('',*,*,#19290,.F.);
#25933=ORIENTED_EDGE('',*,*,#19600,.F.);
#25934=ORIENTED_EDGE('',*,*,#19595,.T.);
#25935=ORIENTED_EDGE('',*,*,#19601,.T.);
#25936=ORIENTED_EDGE('',*,*,#19292,.F.);
#25937=ORIENTED_EDGE('',*,*,#19602,.F.);
#25938=ORIENTED_EDGE('',*,*,#19593,.T.);
#25939=ORIENTED_EDGE('',*,*,#19603,.T.);
#25940=ORIENTED_EDGE('',*,*,#19294,.F.);
#25941=ORIENTED_EDGE('',*,*,#19604,.F.);
#25942=ORIENTED_EDGE('',*,*,#19591,.T.);
#25943=ORIENTED_EDGE('',*,*,#19605,.T.);
#25944=ORIENTED_EDGE('',*,*,#19296,.F.);
#25945=ORIENTED_EDGE('',*,*,#19606,.F.);
#25946=ORIENTED_EDGE('',*,*,#19589,.T.);
#25947=ORIENTED_EDGE('',*,*,#19607,.T.);
#25948=ORIENTED_EDGE('',*,*,#19298,.F.);
#25949=ORIENTED_EDGE('',*,*,#19608,.F.);
#25950=ORIENTED_EDGE('',*,*,#19587,.T.);
#25951=ORIENTED_EDGE('',*,*,#19609,.T.);
#25952=ORIENTED_EDGE('',*,*,#19300,.F.);
#25953=ORIENTED_EDGE('',*,*,#19610,.F.);
#25954=ORIENTED_EDGE('',*,*,#19585,.T.);
#25955=ORIENTED_EDGE('',*,*,#19611,.T.);
#25956=ORIENTED_EDGE('',*,*,#19302,.F.);
#25957=ORIENTED_EDGE('',*,*,#19612,.F.);
#25958=ORIENTED_EDGE('',*,*,#19583,.T.);
#25959=ORIENTED_EDGE('',*,*,#19613,.T.);
#25960=ORIENTED_EDGE('',*,*,#19304,.F.);
#25961=ORIENTED_EDGE('',*,*,#19614,.F.);
#25962=ORIENTED_EDGE('',*,*,#19581,.T.);
#25963=ORIENTED_EDGE('',*,*,#19615,.T.);
#25964=ORIENTED_EDGE('',*,*,#19306,.F.);
#25965=ORIENTED_EDGE('',*,*,#19616,.F.);
#25966=ORIENTED_EDGE('',*,*,#19579,.T.);
#25967=ORIENTED_EDGE('',*,*,#19617,.T.);
#25968=ORIENTED_EDGE('',*,*,#19308,.F.);
#25969=ORIENTED_EDGE('',*,*,#19618,.F.);
#25970=ORIENTED_EDGE('',*,*,#19577,.T.);
#25971=ORIENTED_EDGE('',*,*,#19619,.T.);
#25972=ORIENTED_EDGE('',*,*,#19310,.F.);
#25973=ORIENTED_EDGE('',*,*,#19620,.F.);
#25974=ORIENTED_EDGE('',*,*,#19575,.T.);
#25975=ORIENTED_EDGE('',*,*,#19621,.T.);
#25976=ORIENTED_EDGE('',*,*,#19312,.F.);
#25977=ORIENTED_EDGE('',*,*,#19622,.F.);
#25978=ORIENTED_EDGE('',*,*,#19573,.T.);
#25979=ORIENTED_EDGE('',*,*,#19623,.T.);
#25980=ORIENTED_EDGE('',*,*,#19314,.F.);
#25981=ORIENTED_EDGE('',*,*,#19624,.F.);
#25982=ORIENTED_EDGE('',*,*,#19571,.T.);
#25983=ORIENTED_EDGE('',*,*,#19625,.T.);
#25984=ORIENTED_EDGE('',*,*,#19316,.F.);
#25985=ORIENTED_EDGE('',*,*,#19626,.F.);
#25986=ORIENTED_EDGE('',*,*,#19569,.T.);
#25987=ORIENTED_EDGE('',*,*,#19627,.T.);
#25988=ORIENTED_EDGE('',*,*,#19318,.F.);
#25989=ORIENTED_EDGE('',*,*,#19628,.F.);
#25990=ORIENTED_EDGE('',*,*,#19567,.T.);
#25991=ORIENTED_EDGE('',*,*,#19629,.T.);
#25992=ORIENTED_EDGE('',*,*,#19320,.F.);
#25993=ORIENTED_EDGE('',*,*,#19630,.F.);
#25994=ORIENTED_EDGE('',*,*,#19565,.T.);
#25995=ORIENTED_EDGE('',*,*,#19631,.T.);
#25996=ORIENTED_EDGE('',*,*,#19322,.F.);
#25997=ORIENTED_EDGE('',*,*,#19632,.F.);
#25998=ORIENTED_EDGE('',*,*,#19563,.T.);
#25999=ORIENTED_EDGE('',*,*,#19633,.T.);
#26000=ORIENTED_EDGE('',*,*,#19324,.F.);
#26001=ORIENTED_EDGE('',*,*,#19634,.F.);
#26002=ORIENTED_EDGE('',*,*,#19561,.T.);
#26003=ORIENTED_EDGE('',*,*,#19635,.T.);
#26004=ORIENTED_EDGE('',*,*,#19326,.F.);
#26005=ORIENTED_EDGE('',*,*,#19636,.F.);
#26006=ORIENTED_EDGE('',*,*,#19559,.T.);
#26007=ORIENTED_EDGE('',*,*,#19637,.T.);
#26008=ORIENTED_EDGE('',*,*,#19328,.F.);
#26009=ORIENTED_EDGE('',*,*,#19638,.F.);
#26010=ORIENTED_EDGE('',*,*,#19557,.T.);
#26011=ORIENTED_EDGE('',*,*,#19639,.T.);
#26012=ORIENTED_EDGE('',*,*,#19330,.F.);
#26013=ORIENTED_EDGE('',*,*,#19640,.F.);
#26014=ORIENTED_EDGE('',*,*,#19555,.T.);
#26015=ORIENTED_EDGE('',*,*,#19641,.T.);
#26016=ORIENTED_EDGE('',*,*,#19332,.F.);
#26017=ORIENTED_EDGE('',*,*,#19642,.F.);
#26018=ORIENTED_EDGE('',*,*,#19553,.T.);
#26019=ORIENTED_EDGE('',*,*,#19643,.T.);
#26020=ORIENTED_EDGE('',*,*,#19644,.T.);
#26021=ORIENTED_EDGE('',*,*,#19079,.T.);
#26022=ORIENTED_EDGE('',*,*,#19076,.T.);
#26023=ORIENTED_EDGE('',*,*,#19645,.T.);
#26024=ORIENTED_EDGE('',*,*,#19646,.T.);
#26025=ORIENTED_EDGE('',*,*,#19647,.T.);
#26026=ORIENTED_EDGE('',*,*,#19644,.F.);
#26027=ORIENTED_EDGE('',*,*,#19648,.F.);
#26028=ORIENTED_EDGE('',*,*,#19649,.T.);
#26029=ORIENTED_EDGE('',*,*,#19247,.T.);
#26030=ORIENTED_EDGE('',*,*,#19244,.T.);
#26031=ORIENTED_EDGE('',*,*,#19241,.T.);
#26032=ORIENTED_EDGE('',*,*,#19238,.T.);
#26033=ORIENTED_EDGE('',*,*,#19235,.T.);
#26034=ORIENTED_EDGE('',*,*,#19232,.T.);
#26035=ORIENTED_EDGE('',*,*,#19229,.T.);
#26036=ORIENTED_EDGE('',*,*,#19226,.T.);
#26037=ORIENTED_EDGE('',*,*,#19223,.T.);
#26038=ORIENTED_EDGE('',*,*,#19220,.T.);
#26039=ORIENTED_EDGE('',*,*,#19217,.T.);
#26040=ORIENTED_EDGE('',*,*,#19214,.T.);
#26041=ORIENTED_EDGE('',*,*,#19211,.T.);
#26042=ORIENTED_EDGE('',*,*,#19208,.T.);
#26043=ORIENTED_EDGE('',*,*,#19205,.T.);
#26044=ORIENTED_EDGE('',*,*,#19202,.T.);
#26045=ORIENTED_EDGE('',*,*,#19199,.T.);
#26046=ORIENTED_EDGE('',*,*,#19196,.T.);
#26047=ORIENTED_EDGE('',*,*,#19193,.T.);
#26048=ORIENTED_EDGE('',*,*,#19190,.T.);
#26049=ORIENTED_EDGE('',*,*,#19187,.T.);
#26050=ORIENTED_EDGE('',*,*,#19184,.T.);
#26051=ORIENTED_EDGE('',*,*,#19181,.T.);
#26052=ORIENTED_EDGE('',*,*,#19178,.T.);
#26053=ORIENTED_EDGE('',*,*,#19175,.T.);
#26054=ORIENTED_EDGE('',*,*,#19172,.T.);
#26055=ORIENTED_EDGE('',*,*,#19169,.T.);
#26056=ORIENTED_EDGE('',*,*,#19166,.T.);
#26057=ORIENTED_EDGE('',*,*,#19598,.F.);
#26058=ORIENTED_EDGE('',*,*,#19650,.F.);
#26059=ORIENTED_EDGE('',*,*,#19162,.F.);
#26060=ORIENTED_EDGE('',*,*,#19158,.F.);
#26061=ORIENTED_EDGE('',*,*,#19155,.F.);
#26062=ORIENTED_EDGE('',*,*,#19152,.F.);
#26063=ORIENTED_EDGE('',*,*,#19149,.F.);
#26064=ORIENTED_EDGE('',*,*,#19146,.F.);
#26065=ORIENTED_EDGE('',*,*,#19143,.F.);
#26066=ORIENTED_EDGE('',*,*,#19140,.F.);
#26067=ORIENTED_EDGE('',*,*,#19137,.F.);
#26068=ORIENTED_EDGE('',*,*,#19134,.F.);
#26069=ORIENTED_EDGE('',*,*,#19131,.F.);
#26070=ORIENTED_EDGE('',*,*,#19128,.F.);
#26071=ORIENTED_EDGE('',*,*,#19125,.F.);
#26072=ORIENTED_EDGE('',*,*,#19122,.F.);
#26073=ORIENTED_EDGE('',*,*,#19119,.F.);
#26074=ORIENTED_EDGE('',*,*,#19116,.F.);
#26075=ORIENTED_EDGE('',*,*,#19113,.F.);
#26076=ORIENTED_EDGE('',*,*,#19110,.F.);
#26077=ORIENTED_EDGE('',*,*,#19107,.F.);
#26078=ORIENTED_EDGE('',*,*,#19104,.F.);
#26079=ORIENTED_EDGE('',*,*,#19101,.F.);
#26080=ORIENTED_EDGE('',*,*,#19098,.F.);
#26081=ORIENTED_EDGE('',*,*,#19095,.F.);
#26082=ORIENTED_EDGE('',*,*,#19092,.F.);
#26083=ORIENTED_EDGE('',*,*,#19089,.F.);
#26084=ORIENTED_EDGE('',*,*,#19086,.F.);
#26085=ORIENTED_EDGE('',*,*,#19083,.F.);
#26086=ORIENTED_EDGE('',*,*,#19080,.F.);
#26087=ORIENTED_EDGE('',*,*,#19647,.F.);
#26088=ORIENTED_EDGE('',*,*,#19651,.T.);
#26089=ORIENTED_EDGE('',*,*,#19652,.F.);
#26090=ORIENTED_EDGE('',*,*,#19653,.T.);
#26091=ORIENTED_EDGE('',*,*,#19654,.F.);
#26092=ORIENTED_EDGE('',*,*,#19648,.T.);
#26093=ORIENTED_EDGE('',*,*,#19646,.F.);
#26094=ORIENTED_EDGE('',*,*,#19655,.F.);
#26095=ORIENTED_EDGE('',*,*,#19656,.F.);
#26096=ORIENTED_EDGE('',*,*,#19657,.F.);
#26097=ORIENTED_EDGE('',*,*,#19651,.F.);
#26098=ORIENTED_EDGE('',*,*,#19334,.F.);
#26099=ORIENTED_EDGE('',*,*,#19658,.F.);
#26100=ORIENTED_EDGE('',*,*,#19551,.T.);
#26101=ORIENTED_EDGE('',*,*,#19659,.T.);
#26102=ORIENTED_EDGE('',*,*,#19545,.T.);
#26103=ORIENTED_EDGE('',*,*,#19660,.T.);
#26104=ORIENTED_EDGE('',*,*,#19340,.T.);
#26105=ORIENTED_EDGE('',*,*,#19661,.F.);
#26106=ORIENTED_EDGE('',*,*,#19336,.F.);
#26107=ORIENTED_EDGE('',*,*,#19662,.F.);
#26108=ORIENTED_EDGE('',*,*,#19549,.T.);
#26109=ORIENTED_EDGE('',*,*,#19663,.T.);
#26110=ORIENTED_EDGE('',*,*,#19652,.T.);
#26111=ORIENTED_EDGE('',*,*,#19657,.T.);
#26112=ORIENTED_EDGE('',*,*,#19664,.T.);
#26113=ORIENTED_EDGE('',*,*,#19665,.T.);
#26114=ORIENTED_EDGE('',*,*,#19664,.F.);
#26115=ORIENTED_EDGE('',*,*,#19656,.T.);
#26116=ORIENTED_EDGE('',*,*,#19666,.T.);
#26117=ORIENTED_EDGE('',*,*,#19665,.F.);
#26118=ORIENTED_EDGE('',*,*,#19667,.F.);
#26119=ORIENTED_EDGE('',*,*,#19338,.F.);
#26120=ORIENTED_EDGE('',*,*,#19668,.F.);
#26121=ORIENTED_EDGE('',*,*,#19547,.T.);
#26122=ORIENTED_EDGE('',*,*,#19669,.T.);
#26123=ORIENTED_EDGE('',*,*,#19670,.T.);
#26124=ORIENTED_EDGE('',*,*,#19671,.T.);
#26125=ORIENTED_EDGE('',*,*,#19667,.T.);
#26126=ORIENTED_EDGE('',*,*,#19671,.F.);
#26127=ORIENTED_EDGE('',*,*,#19670,.F.);
#26128=ORIENTED_EDGE('',*,*,#19672,.T.);
#26129=ORIENTED_EDGE('',*,*,#19673,.T.);
#26130=ORIENTED_EDGE('',*,*,#19672,.F.);
#26131=ORIENTED_EDGE('',*,*,#19245,.T.);
#26132=ORIENTED_EDGE('',*,*,#19649,.F.);
#26133=ORIENTED_EDGE('',*,*,#19654,.T.);
#26134=ORIENTED_EDGE('',*,*,#19674,.T.);
#26135=ORIENTED_EDGE('',*,*,#19675,.T.);
#26136=ORIENTED_EDGE('',*,*,#19645,.F.);
#26137=ORIENTED_EDGE('',*,*,#19075,.F.);
#26138=ORIENTED_EDGE('',*,*,#19078,.F.);
#26139=ORIENTED_EDGE('',*,*,#19082,.F.);
#26140=ORIENTED_EDGE('',*,*,#19085,.F.);
#26141=ORIENTED_EDGE('',*,*,#19088,.F.);
#26142=ORIENTED_EDGE('',*,*,#19091,.F.);
#26143=ORIENTED_EDGE('',*,*,#19094,.F.);
#26144=ORIENTED_EDGE('',*,*,#19097,.F.);
#26145=ORIENTED_EDGE('',*,*,#19100,.F.);
#26146=ORIENTED_EDGE('',*,*,#19103,.F.);
#26147=ORIENTED_EDGE('',*,*,#19106,.F.);
#26148=ORIENTED_EDGE('',*,*,#19109,.F.);
#26149=ORIENTED_EDGE('',*,*,#19112,.F.);
#26150=ORIENTED_EDGE('',*,*,#19115,.F.);
#26151=ORIENTED_EDGE('',*,*,#19118,.F.);
#26152=ORIENTED_EDGE('',*,*,#19121,.F.);
#26153=ORIENTED_EDGE('',*,*,#19124,.F.);
#26154=ORIENTED_EDGE('',*,*,#19127,.F.);
#26155=ORIENTED_EDGE('',*,*,#19130,.F.);
#26156=ORIENTED_EDGE('',*,*,#19133,.F.);
#26157=ORIENTED_EDGE('',*,*,#19136,.F.);
#26158=ORIENTED_EDGE('',*,*,#19139,.F.);
#26159=ORIENTED_EDGE('',*,*,#19142,.F.);
#26160=ORIENTED_EDGE('',*,*,#19145,.F.);
#26161=ORIENTED_EDGE('',*,*,#19148,.F.);
#26162=ORIENTED_EDGE('',*,*,#19151,.F.);
#26163=ORIENTED_EDGE('',*,*,#19154,.F.);
#26164=ORIENTED_EDGE('',*,*,#19157,.F.);
#26165=ORIENTED_EDGE('',*,*,#19161,.F.);
#26166=ORIENTED_EDGE('',*,*,#19599,.F.);
#26167=ORIENTED_EDGE('',*,*,#19164,.F.);
#26168=ORIENTED_EDGE('',*,*,#19168,.F.);
#26169=ORIENTED_EDGE('',*,*,#19171,.F.);
#26170=ORIENTED_EDGE('',*,*,#19174,.F.);
#26171=ORIENTED_EDGE('',*,*,#19177,.F.);
#26172=ORIENTED_EDGE('',*,*,#19180,.F.);
#26173=ORIENTED_EDGE('',*,*,#19183,.F.);
#26174=ORIENTED_EDGE('',*,*,#19186,.F.);
#26175=ORIENTED_EDGE('',*,*,#19189,.F.);
#26176=ORIENTED_EDGE('',*,*,#19192,.F.);
#26177=ORIENTED_EDGE('',*,*,#19195,.F.);
#26178=ORIENTED_EDGE('',*,*,#19198,.F.);
#26179=ORIENTED_EDGE('',*,*,#19201,.F.);
#26180=ORIENTED_EDGE('',*,*,#19204,.F.);
#26181=ORIENTED_EDGE('',*,*,#19207,.F.);
#26182=ORIENTED_EDGE('',*,*,#19210,.F.);
#26183=ORIENTED_EDGE('',*,*,#19213,.F.);
#26184=ORIENTED_EDGE('',*,*,#19216,.F.);
#26185=ORIENTED_EDGE('',*,*,#19219,.F.);
#26186=ORIENTED_EDGE('',*,*,#19222,.F.);
#26187=ORIENTED_EDGE('',*,*,#19225,.F.);
#26188=ORIENTED_EDGE('',*,*,#19228,.F.);
#26189=ORIENTED_EDGE('',*,*,#19231,.F.);
#26190=ORIENTED_EDGE('',*,*,#19234,.F.);
#26191=ORIENTED_EDGE('',*,*,#19237,.F.);
#26192=ORIENTED_EDGE('',*,*,#19240,.F.);
#26193=ORIENTED_EDGE('',*,*,#19243,.F.);
#26194=ORIENTED_EDGE('',*,*,#19246,.F.);
#26195=ORIENTED_EDGE('',*,*,#19675,.F.);
#26196=ORIENTED_EDGE('',*,*,#19674,.F.);
#26197=ORIENTED_EDGE('',*,*,#19653,.F.);
#26198=ORIENTED_EDGE('',*,*,#19666,.F.);
#26199=ORIENTED_EDGE('',*,*,#19655,.T.);
#26200=ORIENTED_EDGE('',*,*,#19673,.F.);
#26201=ORIENTED_EDGE('',*,*,#19676,.T.);
#26202=ORIENTED_EDGE('',*,*,#19676,.F.);
#26203=ORIENTED_EDGE('',*,*,#19546,.F.);
#26204=ORIENTED_EDGE('',*,*,#19661,.T.);
#26205=ORIENTED_EDGE('',*,*,#19339,.T.);
#26206=ORIENTED_EDGE('',*,*,#19669,.F.);
#26207=ORIENTED_EDGE('',*,*,#19548,.F.);
#26208=ORIENTED_EDGE('',*,*,#19668,.T.);
#26209=ORIENTED_EDGE('',*,*,#19337,.T.);
#26210=ORIENTED_EDGE('',*,*,#19663,.F.);
#26211=ORIENTED_EDGE('',*,*,#19550,.F.);
#26212=ORIENTED_EDGE('',*,*,#19662,.T.);
#26213=ORIENTED_EDGE('',*,*,#19335,.T.);
#26214=ORIENTED_EDGE('',*,*,#19659,.F.);
#26215=ORIENTED_EDGE('',*,*,#19552,.F.);
#26216=ORIENTED_EDGE('',*,*,#19658,.T.);
#26217=ORIENTED_EDGE('',*,*,#19333,.T.);
#26218=ORIENTED_EDGE('',*,*,#19643,.F.);
#26219=ORIENTED_EDGE('',*,*,#19554,.F.);
#26220=ORIENTED_EDGE('',*,*,#19642,.T.);
#26221=ORIENTED_EDGE('',*,*,#19331,.T.);
#26222=ORIENTED_EDGE('',*,*,#19641,.F.);
#26223=ORIENTED_EDGE('',*,*,#19556,.F.);
#26224=ORIENTED_EDGE('',*,*,#19640,.T.);
#26225=ORIENTED_EDGE('',*,*,#19329,.T.);
#26226=ORIENTED_EDGE('',*,*,#19639,.F.);
#26227=ORIENTED_EDGE('',*,*,#19558,.F.);
#26228=ORIENTED_EDGE('',*,*,#19638,.T.);
#26229=ORIENTED_EDGE('',*,*,#19327,.T.);
#26230=ORIENTED_EDGE('',*,*,#19637,.F.);
#26231=ORIENTED_EDGE('',*,*,#19560,.F.);
#26232=ORIENTED_EDGE('',*,*,#19636,.T.);
#26233=ORIENTED_EDGE('',*,*,#19325,.T.);
#26234=ORIENTED_EDGE('',*,*,#19635,.F.);
#26235=ORIENTED_EDGE('',*,*,#19562,.F.);
#26236=ORIENTED_EDGE('',*,*,#19634,.T.);
#26237=ORIENTED_EDGE('',*,*,#19323,.T.);
#26238=ORIENTED_EDGE('',*,*,#19633,.F.);
#26239=ORIENTED_EDGE('',*,*,#19564,.F.);
#26240=ORIENTED_EDGE('',*,*,#19632,.T.);
#26241=ORIENTED_EDGE('',*,*,#19321,.T.);
#26242=ORIENTED_EDGE('',*,*,#19631,.F.);
#26243=ORIENTED_EDGE('',*,*,#19566,.F.);
#26244=ORIENTED_EDGE('',*,*,#19630,.T.);
#26245=ORIENTED_EDGE('',*,*,#19319,.T.);
#26246=ORIENTED_EDGE('',*,*,#19629,.F.);
#26247=ORIENTED_EDGE('',*,*,#19568,.F.);
#26248=ORIENTED_EDGE('',*,*,#19628,.T.);
#26249=ORIENTED_EDGE('',*,*,#19317,.T.);
#26250=ORIENTED_EDGE('',*,*,#19627,.F.);
#26251=ORIENTED_EDGE('',*,*,#19570,.F.);
#26252=ORIENTED_EDGE('',*,*,#19626,.T.);
#26253=ORIENTED_EDGE('',*,*,#19315,.T.);
#26254=ORIENTED_EDGE('',*,*,#19625,.F.);
#26255=ORIENTED_EDGE('',*,*,#19572,.F.);
#26256=ORIENTED_EDGE('',*,*,#19624,.T.);
#26257=ORIENTED_EDGE('',*,*,#19313,.T.);
#26258=ORIENTED_EDGE('',*,*,#19623,.F.);
#26259=ORIENTED_EDGE('',*,*,#19574,.F.);
#26260=ORIENTED_EDGE('',*,*,#19622,.T.);
#26261=ORIENTED_EDGE('',*,*,#19311,.T.);
#26262=ORIENTED_EDGE('',*,*,#19621,.F.);
#26263=ORIENTED_EDGE('',*,*,#19576,.F.);
#26264=ORIENTED_EDGE('',*,*,#19620,.T.);
#26265=ORIENTED_EDGE('',*,*,#19309,.T.);
#26266=ORIENTED_EDGE('',*,*,#19619,.F.);
#26267=ORIENTED_EDGE('',*,*,#19578,.F.);
#26268=ORIENTED_EDGE('',*,*,#19618,.T.);
#26269=ORIENTED_EDGE('',*,*,#19307,.T.);
#26270=ORIENTED_EDGE('',*,*,#19617,.F.);
#26271=ORIENTED_EDGE('',*,*,#19580,.F.);
#26272=ORIENTED_EDGE('',*,*,#19616,.T.);
#26273=ORIENTED_EDGE('',*,*,#19305,.T.);
#26274=ORIENTED_EDGE('',*,*,#19615,.F.);
#26275=ORIENTED_EDGE('',*,*,#19582,.F.);
#26276=ORIENTED_EDGE('',*,*,#19614,.T.);
#26277=ORIENTED_EDGE('',*,*,#19303,.T.);
#26278=ORIENTED_EDGE('',*,*,#19613,.F.);
#26279=ORIENTED_EDGE('',*,*,#19584,.F.);
#26280=ORIENTED_EDGE('',*,*,#19612,.T.);
#26281=ORIENTED_EDGE('',*,*,#19301,.T.);
#26282=ORIENTED_EDGE('',*,*,#19611,.F.);
#26283=ORIENTED_EDGE('',*,*,#19586,.F.);
#26284=ORIENTED_EDGE('',*,*,#19610,.T.);
#26285=ORIENTED_EDGE('',*,*,#19299,.T.);
#26286=ORIENTED_EDGE('',*,*,#19609,.F.);
#26287=ORIENTED_EDGE('',*,*,#19588,.F.);
#26288=ORIENTED_EDGE('',*,*,#19608,.T.);
#26289=ORIENTED_EDGE('',*,*,#19297,.T.);
#26290=ORIENTED_EDGE('',*,*,#19607,.F.);
#26291=ORIENTED_EDGE('',*,*,#19590,.F.);
#26292=ORIENTED_EDGE('',*,*,#19606,.T.);
#26293=ORIENTED_EDGE('',*,*,#19295,.T.);
#26294=ORIENTED_EDGE('',*,*,#19605,.F.);
#26295=ORIENTED_EDGE('',*,*,#19592,.F.);
#26296=ORIENTED_EDGE('',*,*,#19604,.T.);
#26297=ORIENTED_EDGE('',*,*,#19293,.T.);
#26298=ORIENTED_EDGE('',*,*,#19603,.F.);
#26299=ORIENTED_EDGE('',*,*,#19594,.F.);
#26300=ORIENTED_EDGE('',*,*,#19602,.T.);
#26301=ORIENTED_EDGE('',*,*,#19291,.T.);
#26302=ORIENTED_EDGE('',*,*,#19601,.F.);
#26303=ORIENTED_EDGE('',*,*,#19596,.F.);
#26304=ORIENTED_EDGE('',*,*,#19600,.T.);
#26305=ORIENTED_EDGE('',*,*,#19289,.T.);
#26306=ORIENTED_EDGE('',*,*,#19543,.F.);
#26307=ORIENTED_EDGE('',*,*,#19544,.F.);
#26308=ORIENTED_EDGE('',*,*,#19541,.T.);
#26309=ORIENTED_EDGE('',*,*,#19287,.T.);
#26310=ORIENTED_EDGE('',*,*,#19660,.F.);
#26311=ORIENTED_EDGE('',*,*,#19535,.F.);
#26312=ORIENTED_EDGE('',*,*,#19677,.F.);
#26313=ORIENTED_EDGE('',*,*,#19474,.F.);
#26314=ORIENTED_EDGE('',*,*,#19536,.F.);
#26315=ORIENTED_EDGE('',*,*,#19677,.T.);
#26316=ORIENTED_EDGE('',*,*,#19538,.F.);
#26317=ORIENTED_EDGE('',*,*,#19540,.T.);
#26318=ORIENTED_EDGE('',*,*,#19539,.F.);
#26319=ORIENTED_EDGE('',*,*,#19529,.F.);
#26320=ORIENTED_EDGE('',*,*,#19477,.F.);
#26321=ORIENTED_EDGE('',*,*,#19472,.F.);
#26322=ORIENTED_EDGE('',*,*,#19466,.F.);
#26323=ORIENTED_EDGE('',*,*,#19411,.F.);
#26324=ORIENTED_EDGE('',*,*,#19470,.F.);
#26325=ORIENTED_EDGE('',*,*,#19462,.F.);
#26326=ORIENTED_EDGE('',*,*,#19422,.F.);
#26327=ORIENTED_EDGE('',*,*,#19452,.F.);
#26328=ORIENTED_EDGE('',*,*,#19455,.F.);
#26329=ORIENTED_EDGE('',*,*,#19476,.F.);
#26330=ORIENTED_EDGE('',*,*,#19159,.T.);
#26331=ORIENTED_EDGE('',*,*,#19650,.T.);
#26332=ORIENTED_EDGE('',*,*,#19597,.F.);
#37227=CYLINDRICAL_SURFACE('',#40552,10.925);
#37228=CYLINDRICAL_SURFACE('',#40554,10.925);
#37229=CYLINDRICAL_SURFACE('',#40556,10.925);
#37230=CYLINDRICAL_SURFACE('',#40557,10.925);
#37231=CYLINDRICAL_SURFACE('',#40558,10.925);
#37232=CYLINDRICAL_SURFACE('',#40559,10.925);
#37233=CYLINDRICAL_SURFACE('',#40560,10.925);
#37234=CYLINDRICAL_SURFACE('',#40561,10.925);
#37235=CYLINDRICAL_SURFACE('',#40562,10.925);
#37236=CYLINDRICAL_SURFACE('',#40563,10.925);
#37237=CYLINDRICAL_SURFACE('',#40564,10.925);
#37238=CYLINDRICAL_SURFACE('',#40565,10.925);
#37239=CYLINDRICAL_SURFACE('',#40566,10.925);
#37240=CYLINDRICAL_SURFACE('',#40567,10.925);
#37241=CYLINDRICAL_SURFACE('',#40568,10.925);
#37242=CYLINDRICAL_SURFACE('',#40569,10.925);
#37243=CYLINDRICAL_SURFACE('',#40570,10.925);
#37244=CYLINDRICAL_SURFACE('',#40571,10.925);
#37245=CYLINDRICAL_SURFACE('',#40572,10.925);
#37246=CYLINDRICAL_SURFACE('',#40573,10.925);
#37247=CYLINDRICAL_SURFACE('',#40574,10.925);
#37248=CYLINDRICAL_SURFACE('',#40575,10.925);
#37249=CYLINDRICAL_SURFACE('',#40576,10.925);
#37250=CYLINDRICAL_SURFACE('',#40577,10.925);
#37251=CYLINDRICAL_SURFACE('',#40578,10.925);
#37252=CYLINDRICAL_SURFACE('',#40579,10.925);
#37253=CYLINDRICAL_SURFACE('',#40580,10.925);
#37254=CYLINDRICAL_SURFACE('',#40581,10.925);
#37255=CYLINDRICAL_SURFACE('',#40582,10.925);
#37256=CYLINDRICAL_SURFACE('',#40584,10.0685);
#37257=CYLINDRICAL_SURFACE('',#40586,10.0685);
#37258=CYLINDRICAL_SURFACE('',#40587,10.0685);
#37259=CYLINDRICAL_SURFACE('',#40588,10.0685);
#37260=CYLINDRICAL_SURFACE('',#40589,10.0685);
#37261=CYLINDRICAL_SURFACE('',#40590,10.0685);
#37262=CYLINDRICAL_SURFACE('',#40591,10.0685);
#37263=CYLINDRICAL_SURFACE('',#40592,10.0685);
#37264=CYLINDRICAL_SURFACE('',#40593,10.0685);
#37265=CYLINDRICAL_SURFACE('',#40594,10.0685);
#37266=CYLINDRICAL_SURFACE('',#40595,10.0685);
#37267=CYLINDRICAL_SURFACE('',#40596,10.0685);
#37268=CYLINDRICAL_SURFACE('',#40597,10.0685);
#37269=CYLINDRICAL_SURFACE('',#40598,10.0685);
#37270=CYLINDRICAL_SURFACE('',#40599,10.0685);
#37271=CYLINDRICAL_SURFACE('',#40600,10.0685);
#37272=CYLINDRICAL_SURFACE('',#40601,10.0685);
#37273=CYLINDRICAL_SURFACE('',#40602,10.0685);
#37274=CYLINDRICAL_SURFACE('',#40603,10.0685);
#37275=CYLINDRICAL_SURFACE('',#40604,10.0685);
#37276=CYLINDRICAL_SURFACE('',#40605,10.0685);
#37277=CYLINDRICAL_SURFACE('',#40606,10.0685);
#37278=CYLINDRICAL_SURFACE('',#40607,10.0685);
#37279=CYLINDRICAL_SURFACE('',#40608,10.0685);
#37280=CYLINDRICAL_SURFACE('',#40609,10.0685);
#37281=CYLINDRICAL_SURFACE('',#40610,10.0685);
#37282=CYLINDRICAL_SURFACE('',#40611,10.0685);
#37283=CYLINDRICAL_SURFACE('',#40612,10.0685);
#37284=CYLINDRICAL_SURFACE('',#40617,45.25);
#37285=CYLINDRICAL_SURFACE('',#40630,33.);
#37286=CYLINDRICAL_SURFACE('',#40643,17.);
#37287=CYLINDRICAL_SURFACE('',#40677,14.);
#37288=CYLINDRICAL_SURFACE('',#40701,29.1);
#37289=CYLINDRICAL_SURFACE('',#40725,29.1);
#37290=CYLINDRICAL_SURFACE('',#40758,29.1);
#37291=CYLINDRICAL_SURFACE('',#40789,29.1);
#37292=CYLINDRICAL_SURFACE('',#40790,29.1);
#37293=CYLINDRICAL_SURFACE('',#40796,40.);
#37294=CYLINDRICAL_SURFACE('',#40797,0.999999999999999);
#37295=CYLINDRICAL_SURFACE('',#40827,1.);
#37296=CYLINDRICAL_SURFACE('',#40828,1.);
#37297=CYLINDRICAL_SURFACE('',#40829,0.999999999999999);
#37298=CYLINDRICAL_SURFACE('',#40830,0.999999999999999);
#37299=CYLINDRICAL_SURFACE('',#40831,1.);
#37300=CYLINDRICAL_SURFACE('',#40832,1.);
#37301=CYLINDRICAL_SURFACE('',#40833,1.);
#37302=CYLINDRICAL_SURFACE('',#40834,1.);
#37303=CYLINDRICAL_SURFACE('',#40835,1.);
#37304=CYLINDRICAL_SURFACE('',#40836,1.);
#37305=CYLINDRICAL_SURFACE('',#40837,0.999999999999999);
#37306=CYLINDRICAL_SURFACE('',#40838,1.);
#37307=CYLINDRICAL_SURFACE('',#40839,1.);
#37308=CYLINDRICAL_SURFACE('',#40840,1.);
#37309=CYLINDRICAL_SURFACE('',#40841,1.);
#37310=CYLINDRICAL_SURFACE('',#40842,0.999999999999999);
#37311=CYLINDRICAL_SURFACE('',#40843,1.);
#37312=CYLINDRICAL_SURFACE('',#40844,1.);
#37313=CYLINDRICAL_SURFACE('',#40845,1.);
#37314=CYLINDRICAL_SURFACE('',#40846,1.);
#37315=CYLINDRICAL_SURFACE('',#40847,1.);
#37316=CYLINDRICAL_SURFACE('',#40848,1.);
#37317=CYLINDRICAL_SURFACE('',#40854,1.);
#37318=CYLINDRICAL_SURFACE('',#40855,0.999999999999999);
#37319=CYLINDRICAL_SURFACE('',#40856,0.999999999999999);
#37320=CYLINDRICAL_SURFACE('',#40862,1.);
#37321=CYLINDRICAL_SURFACE('',#40866,2.5);
#37322=CYLINDRICAL_SURFACE('',#40868,10.0685);
#37323=CYLINDRICAL_SURFACE('',#40900,29.1);
#37324=CYLINDRICAL_SURFACE('',#40903,10.925);
#37948=ADVANCED_FACE('',(#2145),#37227,.T.);
#37949=ADVANCED_FACE('',(#2146),#37228,.T.);
#37950=ADVANCED_FACE('',(#2147),#37229,.T.);
#37951=ADVANCED_FACE('',(#2148),#37230,.T.);
#37952=ADVANCED_FACE('',(#2149),#37231,.T.);
#37953=ADVANCED_FACE('',(#2150),#37232,.T.);
#37954=ADVANCED_FACE('',(#2151),#37233,.T.);
#37955=ADVANCED_FACE('',(#2152),#37234,.T.);
#37956=ADVANCED_FACE('',(#2153),#37235,.T.);
#37957=ADVANCED_FACE('',(#2154),#37236,.T.);
#37958=ADVANCED_FACE('',(#2155),#37237,.T.);
#37959=ADVANCED_FACE('',(#2156),#37238,.T.);
#37960=ADVANCED_FACE('',(#2157),#37239,.T.);
#37961=ADVANCED_FACE('',(#2158),#37240,.T.);
#37962=ADVANCED_FACE('',(#2159),#37241,.T.);
#37963=ADVANCED_FACE('',(#2160),#37242,.T.);
#37964=ADVANCED_FACE('',(#2161),#37243,.T.);
#37965=ADVANCED_FACE('',(#2162),#37244,.T.);
#37966=ADVANCED_FACE('',(#2163),#37245,.T.);
#37967=ADVANCED_FACE('',(#2164),#37246,.T.);
#37968=ADVANCED_FACE('',(#2165),#37247,.T.);
#37969=ADVANCED_FACE('',(#2166),#37248,.T.);
#37970=ADVANCED_FACE('',(#2167),#37249,.T.);
#37971=ADVANCED_FACE('',(#2168),#37250,.T.);
#37972=ADVANCED_FACE('',(#2169),#37251,.T.);
#37973=ADVANCED_FACE('',(#2170),#37252,.T.);
#37974=ADVANCED_FACE('',(#2171),#37253,.T.);
#37975=ADVANCED_FACE('',(#2172),#37254,.T.);
#37976=ADVANCED_FACE('',(#2173),#37255,.T.);
#37977=ADVANCED_FACE('',(#2174),#37256,.T.);
#37978=ADVANCED_FACE('',(#2175),#37257,.T.);
#37979=ADVANCED_FACE('',(#2176),#37258,.T.);
#37980=ADVANCED_FACE('',(#2177),#37259,.T.);
#37981=ADVANCED_FACE('',(#2178),#37260,.T.);
#37982=ADVANCED_FACE('',(#2179),#37261,.T.);
#37983=ADVANCED_FACE('',(#2180),#37262,.T.);
#37984=ADVANCED_FACE('',(#2181),#37263,.T.);
#37985=ADVANCED_FACE('',(#2182),#37264,.T.);
#37986=ADVANCED_FACE('',(#2183),#37265,.T.);
#37987=ADVANCED_FACE('',(#2184),#37266,.T.);
#37988=ADVANCED_FACE('',(#2185),#37267,.T.);
#37989=ADVANCED_FACE('',(#2186),#37268,.T.);
#37990=ADVANCED_FACE('',(#2187),#37269,.T.);
#37991=ADVANCED_FACE('',(#2188),#37270,.T.);
#37992=ADVANCED_FACE('',(#2189),#37271,.T.);
#37993=ADVANCED_FACE('',(#2190),#37272,.T.);
#37994=ADVANCED_FACE('',(#2191),#37273,.T.);
#37995=ADVANCED_FACE('',(#2192),#37274,.T.);
#37996=ADVANCED_FACE('',(#2193),#37275,.T.);
#37997=ADVANCED_FACE('',(#2194),#37276,.T.);
#37998=ADVANCED_FACE('',(#2195),#37277,.T.);
#37999=ADVANCED_FACE('',(#2196),#37278,.T.);
#38000=ADVANCED_FACE('',(#2197),#37279,.T.);
#38001=ADVANCED_FACE('',(#2198),#37280,.T.);
#38002=ADVANCED_FACE('',(#2199),#37281,.T.);
#38003=ADVANCED_FACE('',(#2200),#37282,.T.);
#38004=ADVANCED_FACE('',(#2201),#37283,.T.);
#38005=ADVANCED_FACE('',(#2202),#1938,.F.);
#38006=ADVANCED_FACE('',(#2203),#1931,.T.);
#38007=ADVANCED_FACE('',(#2204,#1040),#1116,.T.);
#38008=ADVANCED_FACE('',(#2205),#1939,.F.);
#38009=ADVANCED_FACE('',(#2206),#37284,.T.);
#38010=ADVANCED_FACE('',(#2207),#1940,.F.);
#38011=ADVANCED_FACE('',(#2208),#1932,.T.);
#38012=ADVANCED_FACE('',(#2209),#781,.T.);
#38013=ADVANCED_FACE('',(#2210),#574,.T.);
#38014=ADVANCED_FACE('',(#2211),#37285,.T.);
#38015=ADVANCED_FACE('',(#2212),#782,.T.);
#38016=ADVANCED_FACE('',(#2213,#1041),#1117,.T.);
#38017=ADVANCED_FACE('',(#2214),#783,.T.);
#38018=ADVANCED_FACE('',(#2215,#1042),#1118,.T.);
#38019=ADVANCED_FACE('',(#2216),#37286,.T.);
#38020=ADVANCED_FACE('',(#2217),#784,.T.);
#38021=ADVANCED_FACE('',(#2218,#1043),#1119,.T.);
#38022=ADVANCED_FACE('',(#2219),#37287,.T.);
#38023=ADVANCED_FACE('',(#2220),#1941,.F.);
#38024=ADVANCED_FACE('',(#2221),#1120,.T.);
#38025=ADVANCED_FACE('',(#2222),#1942,.F.);
#38026=ADVANCED_FACE('',(#2223),#1943,.F.);
#38027=ADVANCED_FACE('',(#2224),#1944,.F.);
#38028=ADVANCED_FACE('',(#2225),#290,.T.);
#38029=ADVANCED_FACE('',(#2226),#785,.F.);
#38030=ADVANCED_FACE('',(#2227),#1121,.T.);
#38031=ADVANCED_FACE('',(#2228),#786,.T.);
#38032=ADVANCED_FACE('',(#2229),#291,.T.);
#38033=ADVANCED_FACE('',(#2230),#292,.T.);
#38034=ADVANCED_FACE('',(#2231),#1945,.F.);
#38035=ADVANCED_FACE('',(#2232),#1946,.F.);
#38036=ADVANCED_FACE('',(#2233),#37288,.F.);
#38037=ADVANCED_FACE('',(#2234),#1947,.F.);
#38038=ADVANCED_FACE('',(#2235),#1948,.F.);
#38039=ADVANCED_FACE('',(#2236),#293,.T.);
#38040=ADVANCED_FACE('',(#2237),#1933,.T.);
#38041=ADVANCED_FACE('',(#2238),#1949,.F.);
#38042=ADVANCED_FACE('',(#2239),#1950,.F.);
#38043=ADVANCED_FACE('',(#2240),#1951,.F.);
#38044=ADVANCED_FACE('',(#2241),#1952,.F.);
#38045=ADVANCED_FACE('',(#2242),#1953,.F.);
#38046=ADVANCED_FACE('',(#2243),#1954,.F.);
#38047=ADVANCED_FACE('',(#2244),#294,.T.);
#38048=ADVANCED_FACE('',(#2245),#37289,.F.);
#38049=ADVANCED_FACE('',(#2246),#787,.T.);
#38050=ADVANCED_FACE('',(#2247,#1044),#1122,.T.);
#38051=ADVANCED_FACE('',(#2248),#788,.F.);
#38052=ADVANCED_FACE('',(#2249),#1955,.F.);
#38053=ADVANCED_FACE('',(#2250),#1956,.F.);
#38054=ADVANCED_FACE('',(#2251),#295,.T.);
#38055=ADVANCED_FACE('',(#2252),#789,.T.);
#38056=ADVANCED_FACE('',(#2253),#1957,.F.);
#38057=ADVANCED_FACE('',(#2254),#1958,.F.);
#38058=ADVANCED_FACE('',(#2255),#1959,.F.);
#38059=ADVANCED_FACE('',(#2256),#1960,.F.);
#38060=ADVANCED_FACE('',(#2257),#296,.T.);
#38061=ADVANCED_FACE('',(#2258),#790,.F.);
#38062=ADVANCED_FACE('',(#2259),#1961,.F.);
#38063=ADVANCED_FACE('',(#2260),#1962,.F.);
#38064=ADVANCED_FACE('',(#2261),#297,.T.);
#38065=ADVANCED_FACE('',(#2262),#1963,.F.);
#38066=ADVANCED_FACE('',(#2263),#37290,.F.);
#38067=ADVANCED_FACE('',(#2264),#298,.T.);
#38068=ADVANCED_FACE('',(#2265),#1964,.F.);
#38069=ADVANCED_FACE('',(#2266),#1965,.F.);
#38070=ADVANCED_FACE('',(#2267),#791,.F.);
#38071=ADVANCED_FACE('',(#2268),#1966,.F.);
#38072=ADVANCED_FACE('',(#2269),#792,.T.);
#38073=ADVANCED_FACE('',(#2270),#1967,.F.);
#38074=ADVANCED_FACE('',(#2271),#1968,.F.);
#38075=ADVANCED_FACE('',(#2272),#1969,.F.);
#38076=ADVANCED_FACE('',(#2273),#299,.T.);
#38077=ADVANCED_FACE('',(#2274),#793,.F.);
#38078=ADVANCED_FACE('',(#2275),#1123,.T.);
#38079=ADVANCED_FACE('',(#2276),#1970,.F.);
#38080=ADVANCED_FACE('',(#2277),#1971,.F.);
#38081=ADVANCED_FACE('',(#2278),#300,.T.);
#38082=ADVANCED_FACE('',(#2279),#1972,.F.);
#38083=ADVANCED_FACE('',(#2280),#794,.T.);
#38084=ADVANCED_FACE('',(#2281),#1973,.F.);
#38085=ADVANCED_FACE('',(#2282),#301,.T.);
#38086=ADVANCED_FACE('',(#2283),#795,.T.);
#38087=ADVANCED_FACE('',(#2284),#37291,.F.);
#38088=ADVANCED_FACE('',(#2285),#37292,.F.);
#38089=ADVANCED_FACE('',(#2286),#1974,.F.);
#38090=ADVANCED_FACE('',(#2287),#796,.T.);
#38091=ADVANCED_FACE('',(#2288),#37293,.T.);
#38092=ADVANCED_FACE('',(#2289),#1975,.F.);
#38093=ADVANCED_FACE('',(#2290),#1976,.F.);
#38094=ADVANCED_FACE('',(#2291),#37294,.T.);
#38095=ADVANCED_FACE('',(#2292,#1045),#1124,.T.);
#38096=ADVANCED_FACE('',(#2293),#37295,.T.);
#38097=ADVANCED_FACE('',(#2294),#37296,.T.);
#38098=ADVANCED_FACE('',(#2295),#37297,.T.);
#38099=ADVANCED_FACE('',(#2296),#37298,.T.);
#38100=ADVANCED_FACE('',(#2297),#37299,.T.);
#38101=ADVANCED_FACE('',(#2298),#37300,.T.);
#38102=ADVANCED_FACE('',(#2299),#37301,.T.);
#38103=ADVANCED_FACE('',(#2300),#37302,.T.);
#38104=ADVANCED_FACE('',(#2301),#37303,.T.);
#38105=ADVANCED_FACE('',(#2302),#37304,.T.);
#38106=ADVANCED_FACE('',(#2303),#37305,.T.);
#38107=ADVANCED_FACE('',(#2304),#37306,.T.);
#38108=ADVANCED_FACE('',(#2305),#37307,.T.);
#38109=ADVANCED_FACE('',(#2306),#37308,.T.);
#38110=ADVANCED_FACE('',(#2307),#37309,.T.);
#38111=ADVANCED_FACE('',(#2308),#37310,.T.);
#38112=ADVANCED_FACE('',(#2309),#37311,.T.);
#38113=ADVANCED_FACE('',(#2310),#37312,.T.);
#38114=ADVANCED_FACE('',(#2311),#37313,.T.);
#38115=ADVANCED_FACE('',(#2312),#37314,.T.);
#38116=ADVANCED_FACE('',(#2313),#37315,.T.);
#38117=ADVANCED_FACE('',(#2314),#37316,.T.);
#38118=ADVANCED_FACE('',(#2315),#797,.T.);
#38119=ADVANCED_FACE('',(#2316),#1977,.F.);
#38120=ADVANCED_FACE('',(#2317),#1978,.F.);
#38121=ADVANCED_FACE('',(#2318),#575,.T.);
#38122=ADVANCED_FACE('',(#2319),#37317,.T.);
#38123=ADVANCED_FACE('',(#2320),#37318,.T.);
#38124=ADVANCED_FACE('',(#2321),#37319,.T.);
#38125=ADVANCED_FACE('',(#2322),#798,.T.);
#38126=ADVANCED_FACE('',(#2323,#1046),#1125,.T.);
#38127=ADVANCED_FACE('',(#2324),#37320,.T.);
#38128=ADVANCED_FACE('',(#2325),#799,.T.);
#38129=ADVANCED_FACE('',(#2326),#37321,.F.);
#38130=ADVANCED_FACE('',(#2327),#37322,.T.);
#38131=ADVANCED_FACE('',(#2328),#1979,.F.);
#38132=ADVANCED_FACE('',(#2329),#576,.F.);
#38133=ADVANCED_FACE('',(#2330),#1126,.F.);
#38134=ADVANCED_FACE('',(#2331),#1127,.F.);
#38135=ADVANCED_FACE('',(#2332),#1128,.F.);
#38136=ADVANCED_FACE('',(#2333),#1129,.F.);
#38137=ADVANCED_FACE('',(#2334),#1130,.F.);
#38138=ADVANCED_FACE('',(#2335),#1131,.F.);
#38139=ADVANCED_FACE('',(#2336),#1132,.F.);
#38140=ADVANCED_FACE('',(#2337),#1133,.F.);
#38141=ADVANCED_FACE('',(#2338),#1134,.F.);
#38142=ADVANCED_FACE('',(#2339),#1135,.F.);
#38143=ADVANCED_FACE('',(#2340),#1136,.F.);
#38144=ADVANCED_FACE('',(#2341),#1137,.F.);
#38145=ADVANCED_FACE('',(#2342),#1138,.F.);
#38146=ADVANCED_FACE('',(#2343),#1139,.F.);
#38147=ADVANCED_FACE('',(#2344),#1140,.F.);
#38148=ADVANCED_FACE('',(#2345),#1141,.F.);
#38149=ADVANCED_FACE('',(#2346),#1142,.F.);
#38150=ADVANCED_FACE('',(#2347),#1143,.F.);
#38151=ADVANCED_FACE('',(#2348),#1144,.F.);
#38152=ADVANCED_FACE('',(#2349),#1145,.F.);
#38153=ADVANCED_FACE('',(#2350),#1146,.F.);
#38154=ADVANCED_FACE('',(#2351),#1147,.F.);
#38155=ADVANCED_FACE('',(#2352),#1148,.F.);
#38156=ADVANCED_FACE('',(#2353),#1149,.F.);
#38157=ADVANCED_FACE('',(#2354),#1150,.F.);
#38158=ADVANCED_FACE('',(#2355),#1151,.F.);
#38159=ADVANCED_FACE('',(#2356),#1152,.F.);
#38160=ADVANCED_FACE('',(#2357),#1153,.T.);
#38161=ADVANCED_FACE('',(#2358),#800,.F.);
#38162=ADVANCED_FACE('',(#2359),#37323,.F.);
#38163=ADVANCED_FACE('',(#2360),#1154,.T.);
#38164=ADVANCED_FACE('',(#2361),#1155,.T.);
#38165=ADVANCED_FACE('',(#2362),#37324,.T.);
#40345=CLOSED_SHELL('',(#37948,#37949,#37950,#37951,#37952,#37953,#37954,
#37955,#37956,#37957,#37958,#37959,#37960,#37961,#37962,#37963,#37964,#37965,
#37966,#37967,#37968,#37969,#37970,#37971,#37972,#37973,#37974,#37975,#37976,
#37977,#37978,#37979,#37980,#37981,#37982,#37983,#37984,#37985,#37986,#37987,
#37988,#37989,#37990,#37991,#37992,#37993,#37994,#37995,#37996,#37997,#37998,
#37999,#38000,#38001,#38002,#38003,#38004,#38005,#38006,#38007,#38008,#38009,
#38010,#38011,#38012,#38013,#38014,#38015,#38016,#38017,#38018,#38019,#38020,
#38021,#38022,#38023,#38024,#38025,#38026,#38027,#38028,#38029,#38030,#38031,
#38032,#38033,#38034,#38035,#38036,#38037,#38038,#38039,#38040,#38041,#38042,
#38043,#38044,#38045,#38046,#38047,#38048,#38049,#38050,#38051,#38052,#38053,
#38054,#38055,#38056,#38057,#38058,#38059,#38060,#38061,#38062,#38063,#38064,
#38065,#38066,#38067,#38068,#38069,#38070,#38071,#38072,#38073,#38074,#38075,
#38076,#38077,#38078,#38079,#38080,#38081,#38082,#38083,#38084,#38085,#38086,
#38087,#38088,#38089,#38090,#38091,#38092,#38093,#38094,#38095,#38096,#38097,
#38098,#38099,#38100,#38101,#38102,#38103,#38104,#38105,#38106,#38107,#38108,
#38109,#38110,#38111,#38112,#38113,#38114,#38115,#38116,#38117,#38118,#38119,
#38120,#38121,#38122,#38123,#38124,#38125,#38126,#38127,#38128,#38129,#38130,
#38131,#38132,#38133,#38134,#38135,#38136,#38137,#38138,#38139,#38140,#38141,
#38142,#38143,#38144,#38145,#38146,#38147,#38148,#38149,#38150,#38151,#38152,
#38153,#38154,#38155,#38156,#38157,#38158,#38159,#38160,#38161,#38162,#38163,
#38164,#38165));
#40551=AXIS2_PLACEMENT_3D('',#57283,#45298,#45299);
#40552=AXIS2_PLACEMENT_3D('',#57284,#45300,#45301);
#40553=AXIS2_PLACEMENT_3D('',#57293,#45303,#45304);
#40554=AXIS2_PLACEMENT_3D('',#57294,#45305,#45306);
#40555=AXIS2_PLACEMENT_3D('',#57342,#45308,#45309);
#40556=AXIS2_PLACEMENT_3D('',#57380,#45310,#45311);
#40557=AXIS2_PLACEMENT_3D('',#57470,#45313,#45314);
#40558=AXIS2_PLACEMENT_3D('',#57557,#45316,#45317);
#40559=AXIS2_PLACEMENT_3D('',#57644,#45319,#45320);
#40560=AXIS2_PLACEMENT_3D('',#57731,#45322,#45323);
#40561=AXIS2_PLACEMENT_3D('',#57821,#45325,#45326);
#40562=AXIS2_PLACEMENT_3D('',#57908,#45328,#45329);
#40563=AXIS2_PLACEMENT_3D('',#57995,#45331,#45332);
#40564=AXIS2_PLACEMENT_3D('',#58082,#45334,#45335);
#40565=AXIS2_PLACEMENT_3D('',#58169,#45337,#45338);
#40566=AXIS2_PLACEMENT_3D('',#58259,#45340,#45341);
#40567=AXIS2_PLACEMENT_3D('',#58346,#45343,#45344);
#40568=AXIS2_PLACEMENT_3D('',#58433,#45346,#45347);
#40569=AXIS2_PLACEMENT_3D('',#58523,#45349,#45350);
#40570=AXIS2_PLACEMENT_3D('',#58607,#45352,#45353);
#40571=AXIS2_PLACEMENT_3D('',#58697,#45355,#45356);
#40572=AXIS2_PLACEMENT_3D('',#58784,#45358,#45359);
#40573=AXIS2_PLACEMENT_3D('',#58871,#45361,#45362);
#40574=AXIS2_PLACEMENT_3D('',#58961,#45364,#45365);
#40575=AXIS2_PLACEMENT_3D('',#59045,#45367,#45368);
#40576=AXIS2_PLACEMENT_3D('',#59135,#45370,#45371);
#40577=AXIS2_PLACEMENT_3D('',#59225,#45373,#45374);
#40578=AXIS2_PLACEMENT_3D('',#59309,#45376,#45377);
#40579=AXIS2_PLACEMENT_3D('',#59399,#45379,#45380);
#40580=AXIS2_PLACEMENT_3D('',#59483,#45382,#45383);
#40581=AXIS2_PLACEMENT_3D('',#59573,#45385,#45386);
#40582=AXIS2_PLACEMENT_3D('',#59663,#45388,#45389);
#40583=AXIS2_PLACEMENT_3D('',#59668,#45391,#45392);
#40584=AXIS2_PLACEMENT_3D('',#59743,#45393,#45394);
#40585=AXIS2_PLACEMENT_3D('',#59759,#45396,#45397);
#40586=AXIS2_PLACEMENT_3D('',#59768,#45398,#45399);
#40587=AXIS2_PLACEMENT_3D('',#59805,#45401,#45402);
#40588=AXIS2_PLACEMENT_3D('',#59843,#45404,#45405);
#40589=AXIS2_PLACEMENT_3D('',#59880,#45407,#45408);
#40590=AXIS2_PLACEMENT_3D('',#59917,#45410,#45411);
#40591=AXIS2_PLACEMENT_3D('',#59954,#45413,#45414);
#40592=AXIS2_PLACEMENT_3D('',#59991,#45416,#45417);
#40593=AXIS2_PLACEMENT_3D('',#60029,#45419,#45420);
#40594=AXIS2_PLACEMENT_3D('',#60066,#45422,#45423);
#40595=AXIS2_PLACEMENT_3D('',#60103,#45425,#45426);
#40596=AXIS2_PLACEMENT_3D('',#60140,#45428,#45429);
#40597=AXIS2_PLACEMENT_3D('',#60178,#45431,#45432);
#40598=AXIS2_PLACEMENT_3D('',#60215,#45434,#45435);
#40599=AXIS2_PLACEMENT_3D('',#60252,#45437,#45438);
#40600=AXIS2_PLACEMENT_3D('',#60289,#45440,#45441);
#40601=AXIS2_PLACEMENT_3D('',#60326,#45443,#45444);
#40602=AXIS2_PLACEMENT_3D('',#60364,#45446,#45447);
#40603=AXIS2_PLACEMENT_3D('',#60401,#45449,#45450);
#40604=AXIS2_PLACEMENT_3D('',#60438,#45452,#45453);
#40605=AXIS2_PLACEMENT_3D('',#60476,#45455,#45456);
#40606=AXIS2_PLACEMENT_3D('',#60512,#45458,#45459);
#40607=AXIS2_PLACEMENT_3D('',#60550,#45461,#45462);
#40608=AXIS2_PLACEMENT_3D('',#60587,#45464,#45465);
#40609=AXIS2_PLACEMENT_3D('',#60624,#45467,#45468);
#40610=AXIS2_PLACEMENT_3D('',#60662,#45470,#45471);
#40611=AXIS2_PLACEMENT_3D('',#60698,#45473,#45474);
#40612=AXIS2_PLACEMENT_3D('',#60736,#45476,#45477);
#40613=AXIS2_PLACEMENT_3D('',#60864,#45479,#45480);
#40614=AXIS2_PLACEMENT_3D('',#61121,#45481,#45482);
#40615=AXIS2_PLACEMENT_3D('',#61123,#45483,#45484);
#40616=AXIS2_PLACEMENT_3D('',#61217,#45485,#45486);
#40617=AXIS2_PLACEMENT_3D('',#61246,#45487,#45488);
#40618=AXIS2_PLACEMENT_3D('',#61370,#45490,#45491);
#40619=AXIS2_PLACEMENT_3D('',#61596,#45492,#45493);
#40620=AXIS2_PLACEMENT_3D('',#61597,#45494,#45495);
#40621=AXIS2_PLACEMENT_3D('',#61598,#45496,#45497);
#40622=AXIS2_PLACEMENT_3D('',#61601,#45498,#45499);
#40623=AXIS2_PLACEMENT_3D('',#61602,#45500,#45501);
#40624=AXIS2_PLACEMENT_3D('',#61604,#45502,#45503);
#40625=AXIS2_PLACEMENT_3D('',#61606,#45504,#45505);
#40626=AXIS2_PLACEMENT_3D('',#61607,#45506,#45507);
#40627=AXIS2_PLACEMENT_3D('',#61608,#45508,#45509);
#40628=AXIS2_PLACEMENT_3D('',#61612,#45511,#45512);
#40629=AXIS2_PLACEMENT_3D('',#61613,#45513,#45514);
#40630=AXIS2_PLACEMENT_3D('',#61614,#45515,#45516);
#40631=AXIS2_PLACEMENT_3D('',#61616,#45518,#45519);
#40632=AXIS2_PLACEMENT_3D('',#61618,#45520,#45521);
#40633=AXIS2_PLACEMENT_3D('',#61619,#45522,#45523);
#40634=AXIS2_PLACEMENT_3D('',#61620,#45524,#45525);
#40635=AXIS2_PLACEMENT_3D('',#61622,#45526,#45527);
#40636=AXIS2_PLACEMENT_3D('',#61623,#45528,#45529);
#40637=AXIS2_PLACEMENT_3D('',#61626,#45530,#45531);
#40638=AXIS2_PLACEMENT_3D('',#61627,#45532,#45533);
#40639=AXIS2_PLACEMENT_3D('',#61629,#45534,#45535);
#40640=AXIS2_PLACEMENT_3D('',#61630,#45536,#45537);
#40641=AXIS2_PLACEMENT_3D('',#61631,#45538,#45539);
#40642=AXIS2_PLACEMENT_3D('',#61633,#45540,#45541);
#40643=AXIS2_PLACEMENT_3D('',#61634,#45542,#45543);
#40644=AXIS2_PLACEMENT_3D('',#61636,#45545,#45546);
#40645=AXIS2_PLACEMENT_3D('',#61639,#45547,#45548);
#40646=AXIS2_PLACEMENT_3D('',#61640,#45549,#45550);
#40647=AXIS2_PLACEMENT_3D('',#61642,#45551,#45552);
#40648=AXIS2_PLACEMENT_3D('',#61643,#45553,#45554);
#40649=AXIS2_PLACEMENT_3D('',#61644,#45555,#45556);
#40650=AXIS2_PLACEMENT_3D('',#61649,#45558,#45559);
#40651=AXIS2_PLACEMENT_3D('',#61653,#45561,#45562);
#40652=AXIS2_PLACEMENT_3D('',#61657,#45564,#45565);
#40653=AXIS2_PLACEMENT_3D('',#61661,#45567,#45568);
#40654=AXIS2_PLACEMENT_3D('',#61665,#45570,#45571);
#40655=AXIS2_PLACEMENT_3D('',#61669,#45573,#45574);
#40656=AXIS2_PLACEMENT_3D('',#61673,#45576,#45577);
#40657=AXIS2_PLACEMENT_3D('',#61677,#45579,#45580);
#40658=AXIS2_PLACEMENT_3D('',#61681,#45582,#45583);
#40659=AXIS2_PLACEMENT_3D('',#61685,#45585,#45586);
#40660=AXIS2_PLACEMENT_3D('',#61689,#45588,#45589);
#40661=AXIS2_PLACEMENT_3D('',#61693,#45591,#45592);
#40662=AXIS2_PLACEMENT_3D('',#61697,#45594,#45595);
#40663=AXIS2_PLACEMENT_3D('',#61701,#45597,#45598);
#40664=AXIS2_PLACEMENT_3D('',#61705,#45600,#45601);
#40665=AXIS2_PLACEMENT_3D('',#61709,#45603,#45604);
#40666=AXIS2_PLACEMENT_3D('',#61713,#45606,#45607);
#40667=AXIS2_PLACEMENT_3D('',#61717,#45609,#45610);
#40668=AXIS2_PLACEMENT_3D('',#61721,#45612,#45613);
#40669=AXIS2_PLACEMENT_3D('',#61725,#45615,#45616);
#40670=AXIS2_PLACEMENT_3D('',#61729,#45618,#45619);
#40671=AXIS2_PLACEMENT_3D('',#61733,#45621,#45622);
#40672=AXIS2_PLACEMENT_3D('',#61737,#45624,#45625);
#40673=AXIS2_PLACEMENT_3D('',#61741,#45627,#45628);
#40674=AXIS2_PLACEMENT_3D('',#61745,#45630,#45631);
#40675=AXIS2_PLACEMENT_3D('',#61749,#45633,#45634);
#40676=AXIS2_PLACEMENT_3D('',#61752,#45636,#45637);
#40677=AXIS2_PLACEMENT_3D('',#61753,#45638,#45639);
#40678=AXIS2_PLACEMENT_3D('',#61819,#45641,#45642);
#40679=AXIS2_PLACEMENT_3D('',#61820,#45643,#45644);
#40680=AXIS2_PLACEMENT_3D('',#61913,#45645,#45646);
#40681=AXIS2_PLACEMENT_3D('',#61955,#45647,#45648);
#40682=AXIS2_PLACEMENT_3D('',#61962,#45649,#45650);
#40683=AXIS2_PLACEMENT_3D('',#61964,#45651,#45652);
#40684=AXIS2_PLACEMENT_3D('',#61965,#45653,#45654);
#40685=AXIS2_PLACEMENT_3D('',#61966,#45655,#45656);
#40686=AXIS2_PLACEMENT_3D('',#61967,#45657,#45658);
#40687=AXIS2_PLACEMENT_3D('',#61992,#45659,#45660);
#40688=AXIS2_PLACEMENT_3D('',#61993,#45661,#45662);
#40689=AXIS2_PLACEMENT_3D('',#61996,#45663,#45664);
#40690=AXIS2_PLACEMENT_3D('',#61998,#45665,#45666);
#40691=AXIS2_PLACEMENT_3D('',#62000,#45667,#45668);
#40692=AXIS2_PLACEMENT_3D('',#62001,#45669,#45670);
#40693=AXIS2_PLACEMENT_3D('',#62002,#45671,#45672);
#40694=AXIS2_PLACEMENT_3D('',#62004,#45673,#45674);
#40695=AXIS2_PLACEMENT_3D('',#62005,#45675,#45676);
#40696=AXIS2_PLACEMENT_3D('',#62006,#45677,#45678);
#40697=AXIS2_PLACEMENT_3D('',#62008,#45679,#45680);
#40698=AXIS2_PLACEMENT_3D('',#62009,#45681,#45682);
#40699=AXIS2_PLACEMENT_3D('',#62061,#45683,#45684);
#40700=AXIS2_PLACEMENT_3D('',#62167,#45685,#45686);
#40701=AXIS2_PLACEMENT_3D('',#62174,#45687,#45688);
#40702=AXIS2_PLACEMENT_3D('',#62181,#45689,#45690);
#40703=AXIS2_PLACEMENT_3D('',#62203,#45691,#45692);
#40704=AXIS2_PLACEMENT_3D('',#62211,#45693,#45694);
#40705=AXIS2_PLACEMENT_3D('',#62212,#45695,#45696);
#40706=AXIS2_PLACEMENT_3D('',#62243,#45697,#45698);
#40707=AXIS2_PLACEMENT_3D('',#62245,#45699,#45700);
#40708=AXIS2_PLACEMENT_3D('',#62246,#45701,#45702);
#40709=AXIS2_PLACEMENT_3D('',#62248,#45703,#45704);
#40710=AXIS2_PLACEMENT_3D('',#62278,#45705,#45706);
#40711=AXIS2_PLACEMENT_3D('',#62279,#45707,#45708);
#40712=AXIS2_PLACEMENT_3D('',#62281,#45709,#45710);
#40713=AXIS2_PLACEMENT_3D('',#62305,#45711,#45712);
#40714=AXIS2_PLACEMENT_3D('',#62328,#45713,#45714);
#40715=AXIS2_PLACEMENT_3D('',#62352,#45715,#45716);
#40716=AXIS2_PLACEMENT_3D('',#62391,#45717,#45718);
#40717=AXIS2_PLACEMENT_3D('',#62569,#45719,#45720);
#40718=AXIS2_PLACEMENT_3D('',#62603,#45721,#45722);
#40719=AXIS2_PLACEMENT_3D('',#62661,#45723,#45724);
#40720=AXIS2_PLACEMENT_3D('',#62692,#45725,#45726);
#40721=AXIS2_PLACEMENT_3D('',#62694,#45727,#45728);
#40722=AXIS2_PLACEMENT_3D('',#62700,#45729,#45730);
#40723=AXIS2_PLACEMENT_3D('',#62701,#45731,#45732);
#40724=AXIS2_PLACEMENT_3D('',#62703,#45733,#45734);
#40725=AXIS2_PLACEMENT_3D('',#62704,#45735,#45736);
#40726=AXIS2_PLACEMENT_3D('',#62705,#45737,#45738);
#40727=AXIS2_PLACEMENT_3D('',#62706,#45739,#45740);
#40728=AXIS2_PLACEMENT_3D('',#62707,#45741,#45742);
#40729=AXIS2_PLACEMENT_3D('',#62708,#45743,#45744);
#40730=AXIS2_PLACEMENT_3D('',#62710,#45745,#45746);
#40731=AXIS2_PLACEMENT_3D('',#62712,#45747,#45748);
#40732=AXIS2_PLACEMENT_3D('',#62800,#45749,#45750);
#40733=AXIS2_PLACEMENT_3D('',#62882,#45751,#45752);
#40734=AXIS2_PLACEMENT_3D('',#62969,#45753,#45754);
#40735=AXIS2_PLACEMENT_3D('',#63055,#45755,#45756);
#40736=AXIS2_PLACEMENT_3D('',#63056,#45757,#45758);
#40737=AXIS2_PLACEMENT_3D('',#63145,#45759,#45760);
#40738=AXIS2_PLACEMENT_3D('',#63147,#45761,#45762);
#40739=AXIS2_PLACEMENT_3D('',#63148,#45763,#45764);
#40740=AXIS2_PLACEMENT_3D('',#63149,#45765,#45766);
#40741=AXIS2_PLACEMENT_3D('',#63151,#45767,#45768);
#40742=AXIS2_PLACEMENT_3D('',#63152,#45769,#45770);
#40743=AXIS2_PLACEMENT_3D('',#63184,#45771,#45772);
#40744=AXIS2_PLACEMENT_3D('',#63246,#45773,#45774);
#40745=AXIS2_PLACEMENT_3D('',#63254,#45775,#45776);
#40746=AXIS2_PLACEMENT_3D('',#63293,#45777,#45778);
#40747=AXIS2_PLACEMENT_3D('',#63294,#45779,#45780);
#40748=AXIS2_PLACEMENT_3D('',#63295,#45781,#45782);
#40749=AXIS2_PLACEMENT_3D('',#63296,#45783,#45784);
#40750=AXIS2_PLACEMENT_3D('',#63347,#45785,#45786);
#40751=AXIS2_PLACEMENT_3D('',#63370,#45787,#45788);
#40752=AXIS2_PLACEMENT_3D('',#63372,#45789,#45790);
#40753=AXIS2_PLACEMENT_3D('',#63379,#45791,#45792);
#40754=AXIS2_PLACEMENT_3D('',#63385,#45793,#45794);
#40755=AXIS2_PLACEMENT_3D('',#63386,#45795,#45796);
#40756=AXIS2_PLACEMENT_3D('',#63387,#45797,#45798);
#40757=AXIS2_PLACEMENT_3D('',#63389,#45799,#45800);
#40758=AXIS2_PLACEMENT_3D('',#63420,#45801,#45802);
#40759=AXIS2_PLACEMENT_3D('',#63422,#45803,#45804);
#40760=AXIS2_PLACEMENT_3D('',#63428,#45805,#45806);
#40761=AXIS2_PLACEMENT_3D('',#63431,#45807,#45808);
#40762=AXIS2_PLACEMENT_3D('',#63432,#45809,#45810);
#40763=AXIS2_PLACEMENT_3D('',#63433,#45811,#45812);
#40764=AXIS2_PLACEMENT_3D('',#63455,#45813,#45814);
#40765=AXIS2_PLACEMENT_3D('',#63496,#45815,#45816);
#40766=AXIS2_PLACEMENT_3D('',#63546,#45817,#45818);
#40767=AXIS2_PLACEMENT_3D('',#63548,#45819,#45820);
#40768=AXIS2_PLACEMENT_3D('',#63549,#45821,#45822);
#40769=AXIS2_PLACEMENT_3D('',#63635,#45823,#45824);
#40770=AXIS2_PLACEMENT_3D('',#63671,#45825,#45826);
#40771=AXIS2_PLACEMENT_3D('',#63678,#45827,#45828);
#40772=AXIS2_PLACEMENT_3D('',#63679,#45829,#45830);
#40773=AXIS2_PLACEMENT_3D('',#63680,#45831,#45832);
#40774=AXIS2_PLACEMENT_3D('',#63681,#45833,#45834);
#40775=AXIS2_PLACEMENT_3D('',#63707,#45835,#45836);
#40776=AXIS2_PLACEMENT_3D('',#63732,#45837,#45838);
#40777=AXIS2_PLACEMENT_3D('',#63740,#45839,#45840);
#40778=AXIS2_PLACEMENT_3D('',#63761,#45841,#45842);
#40779=AXIS2_PLACEMENT_3D('',#63762,#45843,#45844);
#40780=AXIS2_PLACEMENT_3D('',#63763,#45845,#45846);
#40781=AXIS2_PLACEMENT_3D('',#63806,#45847,#45848);
#40782=AXIS2_PLACEMENT_3D('',#63807,#45849,#45850);
#40783=AXIS2_PLACEMENT_3D('',#63850,#45851,#45852);
#40784=AXIS2_PLACEMENT_3D('',#63851,#45853,#45854);
#40785=AXIS2_PLACEMENT_3D('',#63853,#45855,#45856);
#40786=AXIS2_PLACEMENT_3D('',#63855,#45857,#45858);
#40787=AXIS2_PLACEMENT_3D('',#63856,#45859,#45860);
#40788=AXIS2_PLACEMENT_3D('',#63857,#45861,#45862);
#40789=AXIS2_PLACEMENT_3D('',#63858,#45863,#45864);
#40790=AXIS2_PLACEMENT_3D('',#63859,#45865,#45866);
#40791=AXIS2_PLACEMENT_3D('',#63886,#45867,#45868);
#40792=AXIS2_PLACEMENT_3D('',#63887,#45869,#45870);
#40793=AXIS2_PLACEMENT_3D('',#63889,#45871,#45872);
#40794=AXIS2_PLACEMENT_3D('',#63891,#45873,#45874);
#40795=AXIS2_PLACEMENT_3D('',#63892,#45875,#45876);
#40796=AXIS2_PLACEMENT_3D('',#63893,#45877,#45878);
#40797=AXIS2_PLACEMENT_3D('',#63978,#45880,#45881);
#40798=AXIS2_PLACEMENT_3D('',#63982,#45883,#45884);
#40799=AXIS2_PLACEMENT_3D('',#63984,#45886,#45887);
#40800=AXIS2_PLACEMENT_3D('',#63988,#45889,#45890);
#40801=AXIS2_PLACEMENT_3D('',#63992,#45892,#45893);
#40802=AXIS2_PLACEMENT_3D('',#63996,#45895,#45896);
#40803=AXIS2_PLACEMENT_3D('',#64000,#45898,#45899);
#40804=AXIS2_PLACEMENT_3D('',#64004,#45901,#45902);
#40805=AXIS2_PLACEMENT_3D('',#64008,#45904,#45905);
#40806=AXIS2_PLACEMENT_3D('',#64012,#45907,#45908);
#40807=AXIS2_PLACEMENT_3D('',#64016,#45910,#45911);
#40808=AXIS2_PLACEMENT_3D('',#64020,#45913,#45914);
#40809=AXIS2_PLACEMENT_3D('',#64024,#45916,#45917);
#40810=AXIS2_PLACEMENT_3D('',#64028,#45919,#45920);
#40811=AXIS2_PLACEMENT_3D('',#64032,#45922,#45923);
#40812=AXIS2_PLACEMENT_3D('',#64036,#45925,#45926);
#40813=AXIS2_PLACEMENT_3D('',#64040,#45928,#45929);
#40814=AXIS2_PLACEMENT_3D('',#64044,#45931,#45932);
#40815=AXIS2_PLACEMENT_3D('',#64048,#45934,#45935);
#40816=AXIS2_PLACEMENT_3D('',#64052,#45937,#45938);
#40817=AXIS2_PLACEMENT_3D('',#64056,#45940,#45941);
#40818=AXIS2_PLACEMENT_3D('',#64060,#45943,#45944);
#40819=AXIS2_PLACEMENT_3D('',#64064,#45946,#45947);
#40820=AXIS2_PLACEMENT_3D('',#64068,#45949,#45950);
#40821=AXIS2_PLACEMENT_3D('',#64072,#45952,#45953);
#40822=AXIS2_PLACEMENT_3D('',#64076,#45955,#45956);
#40823=AXIS2_PLACEMENT_3D('',#64080,#45958,#45959);
#40824=AXIS2_PLACEMENT_3D('',#64084,#45961,#45962);
#40825=AXIS2_PLACEMENT_3D('',#64088,#45964,#45965);
#40826=AXIS2_PLACEMENT_3D('',#64091,#45967,#45968);
#40827=AXIS2_PLACEMENT_3D('',#64346,#45969,#45970);
#40828=AXIS2_PLACEMENT_3D('',#64349,#45973,#45974);
#40829=AXIS2_PLACEMENT_3D('',#64352,#45977,#45978);
#40830=AXIS2_PLACEMENT_3D('',#64355,#45981,#45982);
#40831=AXIS2_PLACEMENT_3D('',#64358,#45985,#45986);
#40832=AXIS2_PLACEMENT_3D('',#64361,#45989,#45990);
#40833=AXIS2_PLACEMENT_3D('',#64364,#45993,#45994);
#40834=AXIS2_PLACEMENT_3D('',#64367,#45997,#45998);
#40835=AXIS2_PLACEMENT_3D('',#64370,#46001,#46002);
#40836=AXIS2_PLACEMENT_3D('',#64373,#46005,#46006);
#40837=AXIS2_PLACEMENT_3D('',#64376,#46009,#46010);
#40838=AXIS2_PLACEMENT_3D('',#64379,#46013,#46014);
#40839=AXIS2_PLACEMENT_3D('',#64382,#46017,#46018);
#40840=AXIS2_PLACEMENT_3D('',#64385,#46021,#46022);
#40841=AXIS2_PLACEMENT_3D('',#64388,#46025,#46026);
#40842=AXIS2_PLACEMENT_3D('',#64391,#46029,#46030);
#40843=AXIS2_PLACEMENT_3D('',#64394,#46033,#46034);
#40844=AXIS2_PLACEMENT_3D('',#64397,#46037,#46038);
#40845=AXIS2_PLACEMENT_3D('',#64400,#46041,#46042);
#40846=AXIS2_PLACEMENT_3D('',#64403,#46045,#46046);
#40847=AXIS2_PLACEMENT_3D('',#64406,#46049,#46050);
#40848=AXIS2_PLACEMENT_3D('',#64409,#46053,#46054);
#40849=AXIS2_PLACEMENT_3D('',#64412,#46057,#46058);
#40850=AXIS2_PLACEMENT_3D('',#64670,#46059,#46060);
#40851=AXIS2_PLACEMENT_3D('',#66340,#46061,#46062);
#40852=AXIS2_PLACEMENT_3D('',#66401,#46063,#46064);
#40853=AXIS2_PLACEMENT_3D('',#66402,#46065,#46066);
#40854=AXIS2_PLACEMENT_3D('',#66403,#46067,#46068);
#40855=AXIS2_PLACEMENT_3D('',#66406,#46071,#46072);
#40856=AXIS2_PLACEMENT_3D('',#66409,#46075,#46076);
#40857=AXIS2_PLACEMENT_3D('',#66412,#46079,#46080);
#40858=AXIS2_PLACEMENT_3D('',#66414,#46081,#46082);
#40859=AXIS2_PLACEMENT_3D('',#66415,#46083,#46084);
#40860=AXIS2_PLACEMENT_3D('',#66477,#46085,#46086);
#40861=AXIS2_PLACEMENT_3D('',#66479,#46087,#46088);
#40862=AXIS2_PLACEMENT_3D('',#66480,#46089,#46090);
#40863=AXIS2_PLACEMENT_3D('',#66483,#46093,#46094);
#40864=AXIS2_PLACEMENT_3D('',#66485,#46095,#46096);
#40865=AXIS2_PLACEMENT_3D('',#66486,#46097,#46098);
#40866=AXIS2_PLACEMENT_3D('',#66487,#46099,#46100);
#40867=AXIS2_PLACEMENT_3D('',#66490,#46102,#46103);
#40868=AXIS2_PLACEMENT_3D('',#66491,#46104,#46105);
#40869=AXIS2_PLACEMENT_3D('',#67979,#46106,#46107);
#40870=AXIS2_PLACEMENT_3D('',#67982,#46109,#46110);
#40871=AXIS2_PLACEMENT_3D('',#67983,#46111,#46112);
#40872=AXIS2_PLACEMENT_3D('',#67984,#46113,#46114);
#40873=AXIS2_PLACEMENT_3D('',#67985,#46115,#46116);
#40874=AXIS2_PLACEMENT_3D('',#67986,#46117,#46118);
#40875=AXIS2_PLACEMENT_3D('',#67987,#46119,#46120);
#40876=AXIS2_PLACEMENT_3D('',#67988,#46121,#46122);
#40877=AXIS2_PLACEMENT_3D('',#67989,#46123,#46124);
#40878=AXIS2_PLACEMENT_3D('',#67990,#46125,#46126);
#40879=AXIS2_PLACEMENT_3D('',#67991,#46127,#46128);
#40880=AXIS2_PLACEMENT_3D('',#67992,#46129,#46130);
#40881=AXIS2_PLACEMENT_3D('',#67993,#46131,#46132);
#40882=AXIS2_PLACEMENT_3D('',#67994,#46133,#46134);
#40883=AXIS2_PLACEMENT_3D('',#67995,#46135,#46136);
#40884=AXIS2_PLACEMENT_3D('',#67996,#46137,#46138);
#40885=AXIS2_PLACEMENT_3D('',#67997,#46139,#46140);
#40886=AXIS2_PLACEMENT_3D('',#67998,#46141,#46142);
#40887=AXIS2_PLACEMENT_3D('',#67999,#46143,#46144);
#40888=AXIS2_PLACEMENT_3D('',#68000,#46145,#46146);
#40889=AXIS2_PLACEMENT_3D('',#68001,#46147,#46148);
#40890=AXIS2_PLACEMENT_3D('',#68002,#46149,#46150);
#40891=AXIS2_PLACEMENT_3D('',#68003,#46151,#46152);
#40892=AXIS2_PLACEMENT_3D('',#68004,#46153,#46154);
#40893=AXIS2_PLACEMENT_3D('',#68005,#46155,#46156);
#40894=AXIS2_PLACEMENT_3D('',#68006,#46157,#46158);
#40895=AXIS2_PLACEMENT_3D('',#68007,#46159,#46160);
#40896=AXIS2_PLACEMENT_3D('',#68008,#46161,#46162);
#40897=AXIS2_PLACEMENT_3D('',#68009,#46163,#46164);
#40898=AXIS2_PLACEMENT_3D('',#68010,#46165,#46166);
#40899=AXIS2_PLACEMENT_3D('',#68011,#46167,#46168);
#40900=AXIS2_PLACEMENT_3D('',#68012,#46169,#46170);
#40901=AXIS2_PLACEMENT_3D('',#68013,#46171,#46172);
#40902=AXIS2_PLACEMENT_3D('',#68014,#46173,#46174);
#40903=AXIS2_PLACEMENT_3D('',#68015,#46175,#46176);
#45298=DIRECTION('axis',(0.,0.,1.));
#45299=DIRECTION('refdir',(1.,0.,0.));
#45300=DIRECTION('center_axis',(1.,0.,0.));
#45301=DIRECTION('ref_axis',(0.,-0.989733601576773,0.142924448258054));
#45302=DIRECTION('',(-1.,0.,0.));
#45303=DIRECTION('center_axis',(-1.,0.,0.));
#45304=DIRECTION('ref_axis',(0.,4.50212443845799E-15,1.));
#45305=DIRECTION('center_axis',(1.,0.,0.));
#45306=DIRECTION('ref_axis',(0.,1.,0.));
#45307=DIRECTION('',(-1.,0.,0.));
#45308=DIRECTION('center_axis',(-1.,0.,0.));
#45309=DIRECTION('ref_axis',(0.,4.50212443845799E-15,1.));
#45310=DIRECTION('center_axis',(1.,0.,0.));
#45311=DIRECTION('ref_axis',(0.,1.,0.));
#45312=DIRECTION('',(-1.,0.,0.));
#45313=DIRECTION('center_axis',(1.,0.,0.));
#45314=DIRECTION('ref_axis',(0.,1.,0.));
#45315=DIRECTION('',(-1.,0.,0.));
#45316=DIRECTION('center_axis',(1.,0.,0.));
#45317=DIRECTION('ref_axis',(0.,1.,0.));
#45318=DIRECTION('',(-1.,0.,0.));
#45319=DIRECTION('center_axis',(1.,0.,0.));
#45320=DIRECTION('ref_axis',(0.,1.,0.));
#45321=DIRECTION('',(-1.,0.,0.));
#45322=DIRECTION('center_axis',(1.,0.,0.));
#45323=DIRECTION('ref_axis',(0.,1.,0.));
#45324=DIRECTION('',(-1.,0.,0.));
#45325=DIRECTION('center_axis',(1.,0.,0.));
#45326=DIRECTION('ref_axis',(0.,1.,0.));
#45327=DIRECTION('',(-1.,0.,0.));
#45328=DIRECTION('center_axis',(1.,0.,0.));
#45329=DIRECTION('ref_axis',(0.,1.,0.));
#45330=DIRECTION('',(-1.,0.,0.));
#45331=DIRECTION('center_axis',(1.,0.,0.));
#45332=DIRECTION('ref_axis',(0.,1.,0.));
#45333=DIRECTION('',(-1.,0.,0.));
#45334=DIRECTION('center_axis',(1.,0.,0.));
#45335=DIRECTION('ref_axis',(0.,1.,0.));
#45336=DIRECTION('',(-1.,0.,0.));
#45337=DIRECTION('center_axis',(1.,0.,0.));
#45338=DIRECTION('ref_axis',(0.,1.,0.));
#45339=DIRECTION('',(-1.,0.,0.));
#45340=DIRECTION('center_axis',(1.,0.,0.));
#45341=DIRECTION('ref_axis',(0.,1.,0.));
#45342=DIRECTION('',(-1.,0.,0.));
#45343=DIRECTION('center_axis',(1.,0.,0.));
#45344=DIRECTION('ref_axis',(0.,1.,0.));
#45345=DIRECTION('',(-1.,0.,0.));
#45346=DIRECTION('center_axis',(1.,0.,0.));
#45347=DIRECTION('ref_axis',(0.,1.,0.));
#45348=DIRECTION('',(-1.,0.,0.));
#45349=DIRECTION('center_axis',(1.,0.,0.));
#45350=DIRECTION('ref_axis',(0.,1.,0.));
#45351=DIRECTION('',(-1.,0.,0.));
#45352=DIRECTION('center_axis',(1.,0.,0.));
#45353=DIRECTION('ref_axis',(0.,1.,0.));
#45354=DIRECTION('',(-1.,0.,0.));
#45355=DIRECTION('center_axis',(1.,0.,0.));
#45356=DIRECTION('ref_axis',(0.,1.,0.));
#45357=DIRECTION('',(-1.,0.,0.));
#45358=DIRECTION('center_axis',(1.,0.,0.));
#45359=DIRECTION('ref_axis',(0.,1.,0.));
#45360=DIRECTION('',(-1.,0.,0.));
#45361=DIRECTION('center_axis',(1.,0.,0.));
#45362=DIRECTION('ref_axis',(0.,1.,0.));
#45363=DIRECTION('',(-1.,0.,0.));
#45364=DIRECTION('center_axis',(1.,0.,0.));
#45365=DIRECTION('ref_axis',(0.,1.,0.));
#45366=DIRECTION('',(-1.,0.,0.));
#45367=DIRECTION('center_axis',(1.,0.,0.));
#45368=DIRECTION('ref_axis',(0.,1.,0.));
#45369=DIRECTION('',(-1.,0.,0.));
#45370=DIRECTION('center_axis',(1.,0.,0.));
#45371=DIRECTION('ref_axis',(0.,1.,0.));
#45372=DIRECTION('',(-1.,0.,0.));
#45373=DIRECTION('center_axis',(1.,0.,0.));
#45374=DIRECTION('ref_axis',(0.,1.,0.));
#45375=DIRECTION('',(-1.,0.,0.));
#45376=DIRECTION('center_axis',(1.,0.,0.));
#45377=DIRECTION('ref_axis',(0.,1.,0.));
#45378=DIRECTION('',(-1.,0.,0.));
#45379=DIRECTION('center_axis',(1.,0.,0.));
#45380=DIRECTION('ref_axis',(0.,1.,0.));
#45381=DIRECTION('',(-1.,0.,0.));
#45382=DIRECTION('center_axis',(1.,0.,0.));
#45383=DIRECTION('ref_axis',(0.,1.,0.));
#45384=DIRECTION('',(-1.,0.,0.));
#45385=DIRECTION('center_axis',(1.,0.,0.));
#45386=DIRECTION('ref_axis',(0.,1.,0.));
#45387=DIRECTION('',(-1.,0.,0.));
#45388=DIRECTION('center_axis',(1.,0.,0.));
#45389=DIRECTION('ref_axis',(0.,1.,0.));
#45390=DIRECTION('',(-1.,0.,0.));
#45391=DIRECTION('center_axis',(1.,0.,0.));
#45392=DIRECTION('ref_axis',(0.,1.,0.));
#45393=DIRECTION('center_axis',(1.,0.,0.));
#45394=DIRECTION('ref_axis',(-2.75667434231801E-17,0.0999709782219109,-0.994990353477537));
#45395=DIRECTION('',(1.,0.,0.));
#45396=DIRECTION('center_axis',(1.,0.,0.));
#45397=DIRECTION('ref_axis',(-2.75667434231801E-17,1.,-8.83977033703589E-14));
#45398=DIRECTION('center_axis',(1.,0.,0.));
#45399=DIRECTION('ref_axis',(-2.75667434231801E-17,1.,-8.83977033703589E-14));
#45400=DIRECTION('',(1.,0.,0.));
#45401=DIRECTION('center_axis',(1.,0.,0.));
#45402=DIRECTION('ref_axis',(-2.75667434231801E-17,1.,-8.83977033703589E-14));
#45403=DIRECTION('',(1.,0.,0.));
#45404=DIRECTION('center_axis',(1.,0.,0.));
#45405=DIRECTION('ref_axis',(-2.75667434231801E-17,1.,-8.83977033703589E-14));
#45406=DIRECTION('',(1.,0.,0.));
#45407=DIRECTION('center_axis',(1.,0.,0.));
#45408=DIRECTION('ref_axis',(-2.75667434231801E-17,1.,-8.83977033703589E-14));
#45409=DIRECTION('',(1.,0.,0.));
#45410=DIRECTION('center_axis',(1.,0.,0.));
#45411=DIRECTION('ref_axis',(-2.75667434231801E-17,1.,-8.83977033703589E-14));
#45412=DIRECTION('',(1.,0.,0.));
#45413=DIRECTION('center_axis',(1.,0.,0.));
#45414=DIRECTION('ref_axis',(-2.75667434231801E-17,1.,-8.83977033703589E-14));
#45415=DIRECTION('',(1.,0.,0.));
#45416=DIRECTION('center_axis',(1.,0.,0.));
#45417=DIRECTION('ref_axis',(-2.75667434231801E-17,1.,-8.83977033703589E-14));
#45418=DIRECTION('',(1.,0.,0.));
#45419=DIRECTION('center_axis',(1.,0.,0.));
#45420=DIRECTION('ref_axis',(-2.75667434231801E-17,1.,-8.83977033703589E-14));
#45421=DIRECTION('',(1.,0.,0.));
#45422=DIRECTION('center_axis',(1.,0.,0.));
#45423=DIRECTION('ref_axis',(-2.75667434231801E-17,1.,-8.83977033703589E-14));
#45424=DIRECTION('',(1.,0.,0.));
#45425=DIRECTION('center_axis',(1.,0.,0.));
#45426=DIRECTION('ref_axis',(-2.75667434231801E-17,1.,-8.83977033703589E-14));
#45427=DIRECTION('',(1.,0.,0.));
#45428=DIRECTION('center_axis',(1.,0.,0.));
#45429=DIRECTION('ref_axis',(-2.75667434231801E-17,1.,-8.83977033703589E-14));
#45430=DIRECTION('',(1.,0.,0.));
#45431=DIRECTION('center_axis',(1.,0.,0.));
#45432=DIRECTION('ref_axis',(-2.75667434231801E-17,1.,-8.83977033703589E-14));
#45433=DIRECTION('',(1.,0.,0.));
#45434=DIRECTION('center_axis',(1.,0.,0.));
#45435=DIRECTION('ref_axis',(-2.75667434231801E-17,1.,-8.83977033703589E-14));
#45436=DIRECTION('',(1.,0.,0.));
#45437=DIRECTION('center_axis',(1.,0.,0.));
#45438=DIRECTION('ref_axis',(-2.75667434231801E-17,1.,-8.83977033703589E-14));
#45439=DIRECTION('',(1.,0.,0.));
#45440=DIRECTION('center_axis',(1.,0.,0.));
#45441=DIRECTION('ref_axis',(-2.75667434231801E-17,1.,-8.83977033703589E-14));
#45442=DIRECTION('',(1.,0.,0.));
#45443=DIRECTION('center_axis',(1.,0.,0.));
#45444=DIRECTION('ref_axis',(-2.75667434231801E-17,1.,-8.83977033703589E-14));
#45445=DIRECTION('',(1.,0.,0.));
#45446=DIRECTION('center_axis',(1.,0.,0.));
#45447=DIRECTION('ref_axis',(-2.75667434231801E-17,1.,-8.83977033703589E-14));
#45448=DIRECTION('',(1.,0.,0.));
#45449=DIRECTION('center_axis',(1.,0.,0.));
#45450=DIRECTION('ref_axis',(-2.75667434231801E-17,1.,-8.83977033703589E-14));
#45451=DIRECTION('',(1.,0.,0.));
#45452=DIRECTION('center_axis',(1.,0.,0.));
#45453=DIRECTION('ref_axis',(-2.75667434231801E-17,1.,-8.83977033703589E-14));
#45454=DIRECTION('',(1.,0.,0.));
#45455=DIRECTION('center_axis',(1.,0.,0.));
#45456=DIRECTION('ref_axis',(-2.75667434231801E-17,1.,-8.83977033703589E-14));
#45457=DIRECTION('',(1.,0.,0.));
#45458=DIRECTION('center_axis',(1.,0.,0.));
#45459=DIRECTION('ref_axis',(-2.75667434231801E-17,1.,-8.83977033703589E-14));
#45460=DIRECTION('',(1.,0.,0.));
#45461=DIRECTION('center_axis',(1.,0.,0.));
#45462=DIRECTION('ref_axis',(-2.75667434231801E-17,1.,-8.83977033703589E-14));
#45463=DIRECTION('',(1.,0.,0.));
#45464=DIRECTION('center_axis',(1.,0.,0.));
#45465=DIRECTION('ref_axis',(-2.75667434231801E-17,1.,-8.83977033703589E-14));
#45466=DIRECTION('',(1.,0.,0.));
#45467=DIRECTION('center_axis',(1.,0.,0.));
#45468=DIRECTION('ref_axis',(-2.75667434231801E-17,1.,-8.83977033703589E-14));
#45469=DIRECTION('',(1.,0.,0.));
#45470=DIRECTION('center_axis',(1.,0.,0.));
#45471=DIRECTION('ref_axis',(-2.75667434231801E-17,1.,-8.83977033703589E-14));
#45472=DIRECTION('',(1.,0.,0.));
#45473=DIRECTION('center_axis',(1.,0.,0.));
#45474=DIRECTION('ref_axis',(-2.75667434231801E-17,1.,-8.83977033703589E-14));
#45475=DIRECTION('',(1.,0.,0.));
#45476=DIRECTION('center_axis',(1.,0.,0.));
#45477=DIRECTION('ref_axis',(-2.75667434231801E-17,1.,-8.83977033703589E-14));
#45478=DIRECTION('',(1.,0.,0.));
#45479=DIRECTION('center_axis',(0.,-9.2713066947687E-16,1.));
#45480=DIRECTION('ref_axis',(1.,0.,0.));
#45481=DIRECTION('center_axis',(1.,0.,0.));
#45482=DIRECTION('ref_axis',(0.,0.,-1.));
#45483=DIRECTION('center_axis',(1.,0.,0.));
#45484=DIRECTION('ref_axis',(0.,0.,-1.));
#45485=DIRECTION('center_axis',(-9.99587409342698E-14,2.22044604925032E-15,
1.));
#45486=DIRECTION('ref_axis',(0.102620742916192,0.99472055529346,8.04911692853245E-15));
#45487=DIRECTION('center_axis',(1.,0.,0.));
#45488=DIRECTION('ref_axis',(0.,1.,0.));
#45489=DIRECTION('',(-1.,0.,0.));
#45490=DIRECTION('center_axis',(2.22242551277839E-15,-2.22044604925032E-15,
1.));
#45491=DIRECTION('ref_axis',(0.,1.,2.22044604925032E-15));
#45492=DIRECTION('center_axis',(1.,0.,0.));
#45493=DIRECTION('ref_axis',(0.,0.,-1.));
#45494=DIRECTION('center_axis',(1.,0.,0.));
#45495=DIRECTION('ref_axis',(0.,0.,-1.));
#45496=DIRECTION('center_axis',(1.,0.,0.));
#45497=DIRECTION('ref_axis',(0.,0.,-1.));
#45498=DIRECTION('center_axis',(-1.,0.,0.));
#45499=DIRECTION('ref_axis',(0.,-1.,1.83697019872103E-16));
#45500=DIRECTION('center_axis',(-1.,0.,0.));
#45501=DIRECTION('ref_axis',(0.,-1.,1.83697019872103E-16));
#45502=DIRECTION('center_axis',(0.,-1.,-1.22464679914735E-16));
#45503=DIRECTION('ref_axis',(0.,-1.22464679914735E-16,1.));
#45504=DIRECTION('center_axis',(1.,0.,0.));
#45505=DIRECTION('ref_axis',(0.,-1.,3.06161699786838E-17));
#45506=DIRECTION('center_axis',(1.,0.,0.));
#45507=DIRECTION('ref_axis',(0.,-1.,3.06161699786838E-17));
#45508=DIRECTION('center_axis',(1.,0.,0.));
#45509=DIRECTION('ref_axis',(0.,1.,0.));
#45510=DIRECTION('',(-0.707106781186548,0.707106781186547,8.65956056235493E-17));
#45511=DIRECTION('center_axis',(-1.,0.,0.));
#45512=DIRECTION('ref_axis',(0.,-1.,3.06161699786838E-17));
#45513=DIRECTION('center_axis',(-1.,0.,0.));
#45514=DIRECTION('ref_axis',(0.,-1.,3.06161699786838E-17));
#45515=DIRECTION('center_axis',(1.,0.,0.));
#45516=DIRECTION('ref_axis',(0.,1.,0.));
#45517=DIRECTION('',(-1.,0.,0.));
#45518=DIRECTION('center_axis',(1.,0.,0.));
#45519=DIRECTION('ref_axis',(0.,0.,-1.));
#45520=DIRECTION('center_axis',(0.,-1.,-1.22464679914735E-16));
#45521=DIRECTION('ref_axis',(0.,-1.22464679914735E-16,1.));
#45522=DIRECTION('center_axis',(1.,0.,0.));
#45523=DIRECTION('ref_axis',(0.,-1.,1.83697019872103E-16));
#45524=DIRECTION('center_axis',(-1.,0.,0.));
#45525=DIRECTION('ref_axis',(0.,0.,1.));
#45526=DIRECTION('center_axis',(1.,0.,0.));
#45527=DIRECTION('ref_axis',(0.,0.,-1.));
#45528=DIRECTION('center_axis',(1.,0.,0.));
#45529=DIRECTION('ref_axis',(0.,0.,-1.));
#45530=DIRECTION('center_axis',(-1.,0.,0.));
#45531=DIRECTION('ref_axis',(0.,-1.,1.83697019872103E-16));
#45532=DIRECTION('center_axis',(-1.,0.,0.));
#45533=DIRECTION('ref_axis',(0.,-1.,1.83697019872103E-16));
#45534=DIRECTION('center_axis',(0.,-1.,-1.22464679914735E-16));
#45535=DIRECTION('ref_axis',(0.,-1.22464679914735E-16,1.));
#45536=DIRECTION('center_axis',(1.,0.,0.));
#45537=DIRECTION('ref_axis',(0.,-1.,1.83697019872103E-16));
#45538=DIRECTION('center_axis',(-1.,0.,0.));
#45539=DIRECTION('ref_axis',(0.,0.,1.));
#45540=DIRECTION('center_axis',(1.,0.,0.));
#45541=DIRECTION('ref_axis',(0.,0.,-1.));
#45542=DIRECTION('center_axis',(1.,0.,0.));
#45543=DIRECTION('ref_axis',(0.,1.,0.));
#45544=DIRECTION('',(-1.,0.,0.));
#45545=DIRECTION('center_axis',(1.,0.,0.));
#45546=DIRECTION('ref_axis',(0.,0.,-1.));
#45547=DIRECTION('center_axis',(-1.,0.,0.));
#45548=DIRECTION('ref_axis',(0.,-1.,1.83697019872103E-16));
#45549=DIRECTION('center_axis',(-1.,0.,0.));
#45550=DIRECTION('ref_axis',(0.,-1.,1.83697019872103E-16));
#45551=DIRECTION('center_axis',(0.,-1.,-1.22464679914735E-16));
#45552=DIRECTION('ref_axis',(0.,-1.22464679914735E-16,1.));
#45553=DIRECTION('center_axis',(1.,0.,0.));
#45554=DIRECTION('ref_axis',(0.,-1.,1.83697019872103E-16));
#45555=DIRECTION('center_axis',(-1.,0.,0.));
#45556=DIRECTION('ref_axis',(0.,0.,1.));
#45557=DIRECTION('',(0.,0.,-1.));
#45558=DIRECTION('center_axis',(1.,0.,0.));
#45559=DIRECTION('ref_axis',(0.,0.689067033753994,0.724697607967262));
#45560=DIRECTION('',(0.,0.23061587074244,-0.973044870579824));
#45561=DIRECTION('center_axis',(1.,0.,0.));
#45562=DIRECTION('ref_axis',(0.,0.503366372793645,0.8640730841431));
#45563=DIRECTION('',(0.,0.448799180200462,-0.893632640323412));
#45564=DIRECTION('center_axis',(1.,0.,0.));
#45565=DIRECTION('ref_axis',(0.,0.290529100384464,0.956866156695802));
#45566=DIRECTION('',(0.,0.642787609686539,-0.766044443118978));
#45567=DIRECTION('center_axis',(1.,0.,0.));
#45568=DIRECTION('ref_axis',(0.,0.0620293289728968,0.998074327065461));
#45569=DIRECTION('',(0.,0.802123192755044,-0.597158591702786));
#45570=DIRECTION('center_axis',(1.,0.,0.));
#45571=DIRECTION('ref_axis',(0.,-0.169814459619289,0.98547605212111));
#45572=DIRECTION('',(0.,0.918216106880274,-0.396079766039157));
#45573=DIRECTION('center_axis',(1.,0.,0.));
#45574=DIRECTION('ref_axis',(0.,-0.392503506738569,0.919750508125941));
#45575=DIRECTION('',(0.,0.984807753012208,-0.17364817766693));
#45576=DIRECTION('center_axis',(1.,0.,0.));
#45577=DIRECTION('ref_axis',(0.,-0.594032588213822,0.804440976169158));
#45578=DIRECTION('',(0.,0.998308158271268,0.0581448289104758));
#45579=DIRECTION('center_axis',(1.,0.,0.));
#45580=DIRECTION('ref_axis',(0.,-0.763537219098866,0.645763822965308));
#45581=DIRECTION('',(0.,0.957989512315489,0.28680323271109));
#45582=DIRECTION('center_axis',(1.,0.,0.));
#45583=DIRECTION('ref_axis',(0.,-0.891879360868045,0.452273374915667));
#45584=DIRECTION('',(0.,0.866025403784439,0.5));
#45585=DIRECTION('center_axis',(1.,0.,0.));
#45586=DIRECTION('ref_axis',(0.,-0.972140055438462,0.234400752157718));
#45587=DIRECTION('',(0.,0.727373641573049,0.686241637868733));
#45588=DIRECTION('center_axis',(1.,0.,0.));
#45589=DIRECTION('ref_axis',(0.,-0.999992427991116,0.00389152417857752));
#45590=DIRECTION('',(0.,0.549508978070806,0.835487811412936));
#45591=DIRECTION('center_axis',(1.,0.,0.));
#45592=DIRECTION('ref_axis',(0.,-0.973934949912377,-0.226827496876316));
#45593=DIRECTION('',(0.,0.342020143325669,0.939692620785908));
#45594=DIRECTION('center_axis',(1.,0.,0.));
#45595=DIRECTION('ref_axis',(0.,-0.895372386590195,-0.445318188862501));
#45596=DIRECTION('',(0.,0.11609291412523,0.993238357741943));
#45597=DIRECTION('center_axis',(1.,0.,0.));
#45598=DIRECTION('ref_axis',(0.,-0.768540066148433,-0.639801662020788));
#45599=DIRECTION('',(0.,-0.11609291412523,0.993238357741943));
#45600=DIRECTION('center_axis',(1.,0.,0.));
#45601=DIRECTION('ref_axis',(0.,-0.600275551811428,-0.799793261973046));
#45602=DIRECTION('',(0.,-0.342020143325669,0.939692620785909));
#45603=DIRECTION('center_axis',(1.,0.,0.));
#45604=DIRECTION('ref_axis',(0.,-0.399650027100731,-0.91666780015357));
#45605=DIRECTION('',(0.,-0.549508978070806,0.835487811412936));
#45606=DIRECTION('center_axis',(1.,0.,0.));
#45607=DIRECTION('ref_axis',(0.,-0.177479265983482,-0.984124539957197));
#45608=DIRECTION('',(0.,-0.727373641573049,0.686241637868734));
#45609=DIRECTION('center_axis',(1.,0.,0.));
#45610=DIRECTION('ref_axis',(0.,0.0542594483017311,-0.998526871080589));
#45611=DIRECTION('',(0.,-0.866025403784438,0.5));
#45612=DIRECTION('center_axis',(1.,0.,0.));
#45613=DIRECTION('ref_axis',(0.,0.283073021684467,-0.95909836012498));
#45614=DIRECTION('',(0.,-0.957989512315489,0.286803232711091));
#45615=DIRECTION('center_axis',(1.,0.,0.));
#45616=DIRECTION('ref_axis',(0.,0.496626055197469,-0.867964608321676));
#45617=DIRECTION('',(0.,-0.998308158271268,0.0581448289104762));
#45618=DIRECTION('center_axis',(1.,0.,0.));
#45619=DIRECTION('ref_axis',(0.,0.683405849527915,-0.730038659819485));
#45620=DIRECTION('',(0.,-0.984807753012208,-0.17364817766693));
#45621=DIRECTION('center_axis',(1.,0.,0.));
#45622=DIRECTION('ref_axis',(0.,0.833343057617297,-0.552756138202965));
#45623=DIRECTION('',(0.,-0.918216106880274,-0.396079766039157));
#45624=DIRECTION('center_axis',(1.,0.,0.));
#45625=DIRECTION('ref_axis',(0.,0.938354525767724,-0.345674390100322));
#45626=DIRECTION('',(0.,-0.802123192755044,-0.597158591702786));
#45627=DIRECTION('center_axis',(1.,0.,0.));
#45628=DIRECTION('ref_axis',(0.,0.992779058549995,-0.119957246152893));
#45629=DIRECTION('',(0.,-0.64278760968654,-0.766044443118978));
#45630=DIRECTION('center_axis',(1.,0.,0.));
#45631=DIRECTION('ref_axis',(0.,0.993682615314554,0.112226823984413));
#45632=DIRECTION('',(0.,-0.448799180200462,-0.893632640323412));
#45633=DIRECTION('center_axis',(1.,0.,0.));
#45634=DIRECTION('ref_axis',(0.,0.941016485082348,0.338360716991886));
#45635=DIRECTION('',(0.,-0.23061587074244,-0.973044870579824));
#45636=DIRECTION('center_axis',(1.,0.,0.));
#45637=DIRECTION('ref_axis',(0.,0.689067033753993,-0.724697607967264));
#45638=DIRECTION('center_axis',(1.,0.,0.));
#45639=DIRECTION('ref_axis',(0.,1.,0.));
#45640=DIRECTION('',(-1.,0.,0.));
#45641=DIRECTION('center_axis',(0.560848145169515,-0.413959345244166,-0.716998618230841));
#45642=DIRECTION('ref_axis',(-0.827918690488332,-0.280424072584758,-0.485708741382183));
#45643=DIRECTION('center_axis',(-0.560848145169515,0.413959345244166,0.716998618230841));
#45644=DIRECTION('ref_axis',(-0.827918690488332,-0.280424072584758,-0.485708741382183));
#45645=DIRECTION('center_axis',(-0.997956501960528,0.0439071569546112,0.0464217811255753));
#45646=DIRECTION('ref_axis',(0.0527884954132498,0.975885776409967,0.211802564084388));
#45647=DIRECTION('center_axis',(-0.979411682864431,-0.141665783972161,-0.143817805296205));
#45648=DIRECTION('ref_axis',(-0.151699271769559,0.98652249625054,0.0613245084463765));
#45649=DIRECTION('center_axis',(0.,0.,1.));
#45650=DIRECTION('ref_axis',(1.,0.,0.));
#45651=DIRECTION('center_axis',(0.,0.0620425458400614,-0.998073505562433));
#45652=DIRECTION('ref_axis',(-0.15169927177702,0.986522496244812,0.0613245085200643));
#45653=DIRECTION('center_axis',(0.,0.701756558301795,0.712416825236757));
#45654=DIRECTION('ref_axis',(0.,-0.712416825236757,0.701756558301795));
#45655=DIRECTION('center_axis',(6.01305526018457E-17,0.866025403784439,
0.5));
#45656=DIRECTION('ref_axis',(-1.,5.20745860967949E-17,3.00652763009229E-17));
#45657=DIRECTION('center_axis',(-0.560848145169515,0.413959345244166,-0.716998618230841));
#45658=DIRECTION('ref_axis',(-0.827918690488332,-0.280424072584758,0.485708741382183));
#45659=DIRECTION('center_axis',(0.560848145169515,-0.413959345244166,0.716998618230841));
#45660=DIRECTION('ref_axis',(-0.827918690488332,-0.280424072584758,0.485708741382183));
#45661=DIRECTION('center_axis',(-1.,0.,0.));
#45662=DIRECTION('ref_axis',(0.,0.,1.));
#45663=DIRECTION('center_axis',(2.27062463608704E-15,0.701756549530087,
-0.712416833877209));
#45664=DIRECTION('ref_axis',(1.,-4.89251306134968E-9,-4.8193005142138E-9));
#45665=DIRECTION('center_axis',(-1.,0.,0.));
#45666=DIRECTION('ref_axis',(0.,0.866025403787478,0.499999999994735));
#45667=DIRECTION('center_axis',(-1.0022629318711E-9,-0.266092789587595,
0.963947419380067));
#45668=DIRECTION('ref_axis',(-2.84217094304039E-13,-0.963947419380068,-0.266092789587595));
#45669=DIRECTION('center_axis',(1.,0.,0.));
#45670=DIRECTION('ref_axis',(0.,0.866025403787478,0.499999999994735));
#45671=DIRECTION('center_axis',(0.,0.,1.));
#45672=DIRECTION('ref_axis',(1.,0.,0.));
#45673=DIRECTION('center_axis',(0.97941168286599,0.053716980910067,-0.194595070409085));
#45674=DIRECTION('ref_axis',(-0.151699271777055,-0.440152665869436,-0.885015797412871));
#45675=DIRECTION('center_axis',(0.,-0.895378283581286,0.445306331968264));
#45676=DIRECTION('ref_axis',(-0.15169927177702,-0.440152665869432,-0.885015797412879));
#45677=DIRECTION('center_axis',(0.,0.,1.));
#45678=DIRECTION('ref_axis',(1.,0.,0.));
#45679=DIRECTION('center_axis',(0.,-0.0620425458400612,-0.998073505562433));
#45680=DIRECTION('ref_axis',(-0.15169927177702,-0.986522496244811,0.0613245085200734));
#45681=DIRECTION('center_axis',(0.979411682865991,-0.141665783970454,0.143817805287263));
#45682=DIRECTION('ref_axis',(-0.151699271777055,-0.986522496244807,0.0613245085200598));
#45683=DIRECTION('center_axis',(0.,0.895378283581287,0.445306331968262));
#45684=DIRECTION('ref_axis',(-0.15169927177702,-0.440152665869428,0.885015797412881));
#45685=DIRECTION('center_axis',(-0.997956501960529,0.0182488632663922,-0.0612356038934034));
#45686=DIRECTION('ref_axis',(0.0527884954132141,-0.304516487121229,-0.951043155605126));
#45687=DIRECTION('center_axis',(1.,0.,0.));
#45688=DIRECTION('ref_axis',(0.,1.,0.));
#45689=DIRECTION('center_axis',(1.,0.,0.));
#45690=DIRECTION('ref_axis',(0.,0.,-1.));
#45691=DIRECTION('center_axis',(0.997955520283696,0.062176287378806,0.0147948917902786));
#45692=DIRECTION('ref_axis',(0.0527881763466631,-0.671369642739936,-0.739240293304718));
#45693=DIRECTION('center_axis',(-0.979411682865068,0.1953827648856,0.0507772651200749));
#45694=DIRECTION('ref_axis',(3.01980662698042E-12,0.251530594143267,-0.967849347889399));
#45695=DIRECTION('center_axis',(-0.979411682865068,0.1953827648856,0.0507772651200749));
#45696=DIRECTION('ref_axis',(3.01980662698042E-12,0.251530594143267,-0.967849347889399));
#45697=DIRECTION('center_axis',(0.,0.,1.));
#45698=DIRECTION('ref_axis',(1.,0.,0.));
#45699=DIRECTION('center_axis',(0.,-0.967849347889388,-0.251530594143311));
#45700=DIRECTION('ref_axis',(0.,-0.251530594143311,0.967849347889388));
#45701=DIRECTION('center_axis',(0.,0.833335737741225,-0.55276717359417));
#45702=DIRECTION('ref_axis',(-0.151699271777054,-0.546369830375377,-0.823691288892807));
#45703=DIRECTION('center_axis',(0.,-1.,0.));
#45704=DIRECTION('ref_axis',(-1.,0.,0.));
#45705=DIRECTION('center_axis',(0.,1.,1.22464679914735E-16));
#45706=DIRECTION('ref_axis',(0.,-1.22464679914735E-16,1.));
#45707=DIRECTION('center_axis',(1.,0.,0.));
#45708=DIRECTION('ref_axis',(0.,0.,-1.));
#45709=DIRECTION('center_axis',(1.,0.,0.));
#45710=DIRECTION('ref_axis',(0.,0.,-1.));
#45711=DIRECTION('center_axis',(1.,0.,0.));
#45712=DIRECTION('ref_axis',(0.,0.,-1.));
#45713=DIRECTION('center_axis',(1.,0.,0.));
#45714=DIRECTION('ref_axis',(0.,0.,-1.));
#45715=DIRECTION('center_axis',(1.,0.,0.));
#45716=DIRECTION('ref_axis',(0.,0.,-1.));
#45717=DIRECTION('center_axis',(1.,0.,0.));
#45718=DIRECTION('ref_axis',(0.,0.,-1.));
#45719=DIRECTION('center_axis',(0.,0.833335737741225,0.552767173594171));
#45720=DIRECTION('ref_axis',(1.,0.,0.));
#45721=DIRECTION('center_axis',(0.997955520283694,0.0439008958260411,-0.0464487984879237));
#45722=DIRECTION('ref_axis',(0.0527881763466811,-0.975885694872911,0.21180301929011));
#45723=DIRECTION('center_axis',(-0.997956501960528,0.0621560202209746,-0.0148138227678562));
#45724=DIRECTION('ref_axis',(0.0527884954132495,0.671369289288742,-0.739240591520741));
#45725=DIRECTION('center_axis',(-0.9794116829089,-0.195382764611353,0.0507772653298721));
#45726=DIRECTION('ref_axis',(-0.151699271791763,0.54636983035541,-0.823691288903343));
#45727=DIRECTION('center_axis',(-0.9794116829089,-0.195382764611353,0.0507772653298721));
#45728=DIRECTION('ref_axis',(-0.151699271791763,0.54636983035541,-0.823691288903343));
#45729=DIRECTION('center_axis',(0.,0.,1.));
#45730=DIRECTION('ref_axis',(1.,0.,0.));
#45731=DIRECTION('center_axis',(0.,0.967849347888444,-0.251530594146943));
#45732=DIRECTION('ref_axis',(0.,0.251530594146943,0.967849347888444));
#45733=DIRECTION('center_axis',(0.,-1.,0.));
#45734=DIRECTION('ref_axis',(-1.,0.,0.));
#45735=DIRECTION('center_axis',(1.,0.,0.));
#45736=DIRECTION('ref_axis',(0.,1.,0.));
#45737=DIRECTION('center_axis',(-1.,0.,0.));
#45738=DIRECTION('ref_axis',(0.,6.12323399573677E-17,1.));
#45739=DIRECTION('center_axis',(-1.,0.,0.));
#45740=DIRECTION('ref_axis',(0.,0.,1.));
#45741=DIRECTION('center_axis',(1.,0.,0.));
#45742=DIRECTION('ref_axis',(0.,6.12323399573677E-17,1.));
#45743=DIRECTION('center_axis',(1.,0.,0.));
#45744=DIRECTION('ref_axis',(0.,0.,-1.));
#45745=DIRECTION('center_axis',(-1.,0.,0.));
#45746=DIRECTION('ref_axis',(0.,-1.,1.83697019872103E-16));
#45747=DIRECTION('center_axis',(1.,0.,0.));
#45748=DIRECTION('ref_axis',(0.,0.878371943987857,-0.477977748451738));
#45749=DIRECTION('center_axis',(1.,0.,0.));
#45750=DIRECTION('ref_axis',(0.,-0.0252450992899237,-0.999681291693429));
#45751=DIRECTION('center_axis',(1.,0.,0.));
#45752=DIRECTION('ref_axis',(0.,-0.866025403784439,-0.499999999999999));
#45753=DIRECTION('center_axis',(1.,0.,0.));
#45754=DIRECTION('ref_axis',(0.,-0.866025403784438,0.5));
#45755=DIRECTION('center_axis',(6.01305526018457E-17,0.866025403784439,
-0.5));
#45756=DIRECTION('ref_axis',(-1.,5.20745860967949E-17,-3.00652763009229E-17));
#45757=DIRECTION('center_axis',(-0.560848145169515,-0.413959345244166,-0.716998618230841));
#45758=DIRECTION('ref_axis',(-0.827918690488332,0.280424072584758,0.485708741382183));
#45759=DIRECTION('center_axis',(0.,0.,1.));
#45760=DIRECTION('ref_axis',(1.,0.,0.));
#45761=DIRECTION('center_axis',(0.97941168286599,0.0537169809100669,0.194595070409084));
#45762=DIRECTION('ref_axis',(-0.151699271777019,-0.440152665869421,0.885015797412885));
#45763=DIRECTION('center_axis',(0.,0.266092789587593,0.963947419380068));
#45764=DIRECTION('ref_axis',(0.,0.963947419380068,-0.266092789587593));
#45765=DIRECTION('center_axis',(-1.,0.,0.));
#45766=DIRECTION('ref_axis',(0.,0.,1.));
#45767=DIRECTION('center_axis',(-1.,0.,0.));
#45768=DIRECTION('ref_axis',(0.,0.878371943987857,-0.477977748451738));
#45769=DIRECTION('center_axis',(-2.05302302574653E-15,0.701756558301643,
0.712416825236906));
#45770=DIRECTION('ref_axis',(0.,-0.712416825236906,0.701756558301643));
#45771=DIRECTION('center_axis',(0.997955520283697,-0.0182753915527593,-0.0612436902781804));
#45772=DIRECTION('ref_axis',(0.0527881763466631,-0.304516052132975,0.951043312594827));
#45773=DIRECTION('center_axis',(-0.979411682865291,0.141665783972824,0.14381780528969));
#45774=DIRECTION('ref_axis',(-0.151699271769167,-0.986522496250837,-0.0613245084425527));
#45775=DIRECTION('center_axis',(0.997955520283697,0.0439008958260354,0.0464487984878664));
#45776=DIRECTION('ref_axis',(1.77635683940025E-14,-0.726758589821175,0.686892969916811));
#45777=DIRECTION('center_axis',(0.,0.,1.));
#45778=DIRECTION('ref_axis',(1.,0.,0.));
#45779=DIRECTION('center_axis',(0.,-0.0620425458402145,0.998073505562424));
#45780=DIRECTION('ref_axis',(-0.151699271776983,-0.986522496244807,-0.0613245085202239));
#45781=DIRECTION('center_axis',(6.01305526018457E-17,1.15635678080473E-17,
-1.));
#45782=DIRECTION('ref_axis',(-1.,0.,-6.01305526018457E-17));
#45783=DIRECTION('center_axis',(-0.560848145169515,-0.827918690488332,-4.32978028117747E-17));
#45784=DIRECTION('ref_axis',(-0.827918690488332,0.560848145169516,-4.91959218075756E-17));
#45785=DIRECTION('center_axis',(0.,-0.833335737741225,0.552767173594171));
#45786=DIRECTION('ref_axis',(-0.151699271777055,0.546369830375374,0.823691288892809));
#45787=DIRECTION('center_axis',(-0.979411682930197,0.195382764526521,-0.050777265245526));
#45788=DIRECTION('ref_axis',(-0.151699272085678,-0.5463698328889,0.823691287168701));
#45789=DIRECTION('center_axis',(-0.979411682930197,0.195382764526521,-0.050777265245526));
#45790=DIRECTION('ref_axis',(-0.151699272085678,-0.5463698328889,0.823691287168701));
#45791=DIRECTION('center_axis',(0.997955520283696,0.062176287378806,-0.0147948917902787));
#45792=DIRECTION('ref_axis',(-1.77635683940025E-14,0.23148746671831,0.972837886162098));
#45793=DIRECTION('center_axis',(0.,0.,1.));
#45794=DIRECTION('ref_axis',(1.,0.,0.));
#45795=DIRECTION('center_axis',(0.,0.833335737741226,0.55276717359417));
#45796=DIRECTION('ref_axis',(-0.15169927177702,-0.546369830375385,0.823691288892808));
#45797=DIRECTION('center_axis',(0.,-0.967849347889388,0.251530594143311));
#45798=DIRECTION('ref_axis',(0.,-0.251530594143311,-0.967849347889388));
#45799=DIRECTION('center_axis',(0.,-1.,0.));
#45800=DIRECTION('ref_axis',(-1.,0.,0.));
#45801=DIRECTION('center_axis',(1.,0.,0.));
#45802=DIRECTION('ref_axis',(0.,1.,0.));
#45803=DIRECTION('center_axis',(-1.,0.,0.));
#45804=DIRECTION('ref_axis',(0.,-0.0252450992899237,-0.999681291693429));
#45805=DIRECTION('center_axis',(0.,0.,1.));
#45806=DIRECTION('ref_axis',(1.,0.,0.));
#45807=DIRECTION('center_axis',(0.979411682865984,0.141665783970477,-0.143817805287287));
#45808=DIRECTION('ref_axis',(-0.151699271777056,0.986522496244806,-0.0613245085200689));
#45809=DIRECTION('center_axis',(0.,0.701756558301794,-0.712416825236758));
#45810=DIRECTION('ref_axis',(0.,-0.712416825236758,-0.701756558301794));
#45811=DIRECTION('center_axis',(0.,0.062042545840064,0.998073505562433));
#45812=DIRECTION('ref_axis',(-0.151699271777056,0.986522496244806,-0.0613245085200689));
#45813=DIRECTION('center_axis',(0.997955520283696,-0.0439008958260262,0.0464487984879082));
#45814=DIRECTION('ref_axis',(0.0527881763466632,0.975885694872913,-0.211803019290109));
#45815=DIRECTION('center_axis',(6.01305526018457E-17,-0.866025403784438,
0.5));
#45816=DIRECTION('ref_axis',(-1.,-5.20745860967949E-17,3.00652763009229E-17));
#45817=DIRECTION('center_axis',(-1.,0.,0.));
#45818=DIRECTION('ref_axis',(0.,0.,1.));
#45819=DIRECTION('center_axis',(-1.,0.,0.));
#45820=DIRECTION('ref_axis',(0.,-0.866025403784439,-0.499999999999999));
#45821=DIRECTION('center_axis',(0.,-0.266092789587593,0.963947419380068));
#45822=DIRECTION('ref_axis',(0.,-0.963947419380068,-0.266092789587593));
#45823=DIRECTION('center_axis',(-0.997956501960528,-0.0182488632663636,
0.0612356038934314));
#45824=DIRECTION('ref_axis',(0.0527884954132496,0.304516487121225,0.951043155605125));
#45825=DIRECTION('center_axis',(-0.979411682975476,0.0537169804255689,-0.194595069991775));
#45826=DIRECTION('ref_axis',(-0.151699272303354,0.440152661180134,0.88501579965483));
#45827=DIRECTION('center_axis',(0.,0.,1.));
#45828=DIRECTION('ref_axis',(1.,0.,0.));
#45829=DIRECTION('center_axis',(0.,0.895378283581287,-0.445306331968262));
#45830=DIRECTION('ref_axis',(-0.15169927177702,0.440152665869428,0.885015797412881));
#45831=DIRECTION('center_axis',(6.01305526018457E-17,1.10901112106688E-16,
1.));
#45832=DIRECTION('ref_axis',(-1.,0.,6.01305526018457E-17));
#45833=DIRECTION('center_axis',(-0.560848145169515,0.827918690488332,-5.80929946143057E-17));
#45834=DIRECTION('ref_axis',(-0.827918690488332,-0.560848145169516,1.17880010386533E-16));
#45835=DIRECTION('center_axis',(0.560848145169515,-0.827918690488332,5.80929946143057E-17));
#45836=DIRECTION('ref_axis',(-0.827918690488332,-0.560848145169515,1.17880010386533E-16));
#45837=DIRECTION('center_axis',(0.997955520283695,0.0182753915527653,0.0612436902782009));
#45838=DIRECTION('ref_axis',(0.0527881763466808,0.304516052132974,-0.951043312594826));
#45839=DIRECTION('center_axis',(-0.979411682975439,0.0537169804257189,0.194595069991925));
#45840=DIRECTION('ref_axis',(-3.62341268100864E-10,0.963947419381388,-0.266092789582811));
#45841=DIRECTION('center_axis',(0.,0.,1.));
#45842=DIRECTION('ref_axis',(1.,0.,0.));
#45843=DIRECTION('center_axis',(0.,-0.266092789587593,-0.963947419380068));
#45844=DIRECTION('ref_axis',(0.,-0.963947419380068,0.266092789587593));
#45845=DIRECTION('center_axis',(0.,0.895378283581287,0.445306331968264));
#45846=DIRECTION('ref_axis',(-0.151699271777055,0.440152665869426,-0.885015797412876));
#45847=DIRECTION('center_axis',(-1.,0.,0.));
#45848=DIRECTION('ref_axis',(0.,0.,1.));
#45849=DIRECTION('center_axis',(-1.,0.,0.));
#45850=DIRECTION('ref_axis',(0.,-0.866025403784438,0.5));
#45851=DIRECTION('center_axis',(0.,0.,1.));
#45852=DIRECTION('ref_axis',(1.,0.,0.));
#45853=DIRECTION('center_axis',(-3.1810942935187E-15,0.967849347889387,
0.251530594143314));
#45854=DIRECTION('ref_axis',(3.55271367880051E-14,-0.251530594143319,0.967849347889386));
#45855=DIRECTION('center_axis',(0.97941168286599,0.195382764880523,0.0507772651218205));
#45856=DIRECTION('ref_axis',(-0.15169927177702,0.546369830375381,0.82369128889281));
#45857=DIRECTION('center_axis',(0.,-1.,0.));
#45858=DIRECTION('ref_axis',(-1.,0.,0.));
#45859=DIRECTION('center_axis',(0.97941168286599,0.195382764880523,0.0507772651218205));
#45860=DIRECTION('ref_axis',(-0.15169927177702,0.546369830375381,0.82369128889281));
#45861=DIRECTION('center_axis',(-1.,0.,0.));
#45862=DIRECTION('ref_axis',(0.,-1.45584689456842E-12,-1.));
#45863=DIRECTION('center_axis',(1.,0.,0.));
#45864=DIRECTION('ref_axis',(0.,1.,0.));
#45865=DIRECTION('center_axis',(1.,0.,0.));
#45866=DIRECTION('ref_axis',(0.,1.,0.));
#45867=DIRECTION('center_axis',(0.997955520283694,-0.0621762873788267,-0.0147948917902837));
#45868=DIRECTION('ref_axis',(0.0527881763466809,0.671369642739935,0.739240293304717));
#45869=DIRECTION('center_axis',(1.,0.,0.));
#45870=DIRECTION('ref_axis',(0.,0.,-1.));
#45871=DIRECTION('center_axis',(0.,-1.,-1.22464679914735E-16));
#45872=DIRECTION('ref_axis',(0.,-1.22464679914735E-16,1.));
#45873=DIRECTION('center_axis',(1.,0.,0.));
#45874=DIRECTION('ref_axis',(0.,-1.,1.83697019872103E-16));
#45875=DIRECTION('center_axis',(1.,0.,0.));
#45876=DIRECTION('ref_axis',(0.,-1.,1.83697019872103E-16));
#45877=DIRECTION('center_axis',(1.,0.,0.));
#45878=DIRECTION('ref_axis',(0.,1.,0.));
#45879=DIRECTION('',(-1.,0.,0.));
#45880=DIRECTION('center_axis',(-1.,0.,0.));
#45881=DIRECTION('ref_axis',(0.,0.689067033753994,0.724697607967262));
#45882=DIRECTION('',(1.,0.,0.));
#45883=DIRECTION('center_axis',(1.,0.,0.));
#45884=DIRECTION('ref_axis',(0.,0.689067033753994,0.724697607967262));
#45885=DIRECTION('',(1.,0.,0.));
#45886=DIRECTION('center_axis',(-1.,0.,0.));
#45887=DIRECTION('ref_axis',(0.,0.,1.));
#45888=DIRECTION('',(0.,0.,-1.));
#45889=DIRECTION('center_axis',(1.,0.,0.));
#45890=DIRECTION('ref_axis',(0.,0.689067033753993,-0.724697607967264));
#45891=DIRECTION('',(0.,-0.23061587074244,-0.973044870579824));
#45892=DIRECTION('center_axis',(1.,0.,0.));
#45893=DIRECTION('ref_axis',(0.,0.941016485082348,0.338360716991886));
#45894=DIRECTION('',(0.,-0.448799180200462,-0.893632640323412));
#45895=DIRECTION('center_axis',(1.,0.,0.));
#45896=DIRECTION('ref_axis',(0.,0.993682615314554,0.112226823984413));
#45897=DIRECTION('',(0.,-0.64278760968654,-0.766044443118978));
#45898=DIRECTION('center_axis',(1.,0.,0.));
#45899=DIRECTION('ref_axis',(0.,0.992779058549995,-0.119957246152893));
#45900=DIRECTION('',(0.,-0.802123192755044,-0.597158591702786));
#45901=DIRECTION('center_axis',(1.,0.,0.));
#45902=DIRECTION('ref_axis',(0.,0.938354525767724,-0.345674390100322));
#45903=DIRECTION('',(0.,-0.918216106880274,-0.396079766039157));
#45904=DIRECTION('center_axis',(1.,0.,0.));
#45905=DIRECTION('ref_axis',(0.,0.833343057617297,-0.552756138202965));
#45906=DIRECTION('',(0.,-0.984807753012208,-0.17364817766693));
#45907=DIRECTION('center_axis',(1.,0.,0.));
#45908=DIRECTION('ref_axis',(0.,0.683405849527915,-0.730038659819485));
#45909=DIRECTION('',(0.,-0.998308158271268,0.0581448289104762));
#45910=DIRECTION('center_axis',(1.,0.,0.));
#45911=DIRECTION('ref_axis',(0.,0.496626055197469,-0.867964608321676));
#45912=DIRECTION('',(0.,-0.957989512315489,0.286803232711091));
#45913=DIRECTION('center_axis',(1.,0.,0.));
#45914=DIRECTION('ref_axis',(0.,0.283073021684467,-0.95909836012498));
#45915=DIRECTION('',(0.,-0.866025403784438,0.5));
#45916=DIRECTION('center_axis',(1.,0.,0.));
#45917=DIRECTION('ref_axis',(0.,0.0542594483017311,-0.998526871080589));
#45918=DIRECTION('',(0.,-0.727373641573049,0.686241637868734));
#45919=DIRECTION('center_axis',(1.,0.,0.));
#45920=DIRECTION('ref_axis',(0.,-0.177479265983482,-0.984124539957197));
#45921=DIRECTION('',(0.,-0.549508978070806,0.835487811412936));
#45922=DIRECTION('center_axis',(1.,0.,0.));
#45923=DIRECTION('ref_axis',(0.,-0.399650027100731,-0.91666780015357));
#45924=DIRECTION('',(0.,-0.342020143325669,0.939692620785909));
#45925=DIRECTION('center_axis',(1.,0.,0.));
#45926=DIRECTION('ref_axis',(0.,-0.600275551811428,-0.799793261973046));
#45927=DIRECTION('',(0.,-0.11609291412523,0.993238357741943));
#45928=DIRECTION('center_axis',(1.,0.,0.));
#45929=DIRECTION('ref_axis',(0.,-0.768540066148433,-0.639801662020788));
#45930=DIRECTION('',(0.,0.11609291412523,0.993238357741943));
#45931=DIRECTION('center_axis',(1.,0.,0.));
#45932=DIRECTION('ref_axis',(0.,-0.895372386590195,-0.445318188862501));
#45933=DIRECTION('',(0.,0.342020143325669,0.939692620785908));
#45934=DIRECTION('center_axis',(1.,0.,0.));
#45935=DIRECTION('ref_axis',(0.,-0.973934949912377,-0.226827496876316));
#45936=DIRECTION('',(0.,0.549508978070806,0.835487811412936));
#45937=DIRECTION('center_axis',(1.,0.,0.));
#45938=DIRECTION('ref_axis',(0.,-0.999992427991116,0.00389152417857752));
#45939=DIRECTION('',(0.,0.727373641573049,0.686241637868733));
#45940=DIRECTION('center_axis',(1.,0.,0.));
#45941=DIRECTION('ref_axis',(0.,-0.972140055438462,0.234400752157718));
#45942=DIRECTION('',(0.,0.866025403784439,0.5));
#45943=DIRECTION('center_axis',(1.,0.,0.));
#45944=DIRECTION('ref_axis',(0.,-0.891879360868045,0.452273374915667));
#45945=DIRECTION('',(0.,0.957989512315489,0.28680323271109));
#45946=DIRECTION('center_axis',(1.,0.,0.));
#45947=DIRECTION('ref_axis',(0.,-0.763537219098866,0.645763822965308));
#45948=DIRECTION('',(0.,0.998308158271268,0.0581448289104758));
#45949=DIRECTION('center_axis',(1.,0.,0.));
#45950=DIRECTION('ref_axis',(0.,-0.594032588213822,0.804440976169158));
#45951=DIRECTION('',(0.,0.984807753012208,-0.17364817766693));
#45952=DIRECTION('center_axis',(1.,0.,0.));
#45953=DIRECTION('ref_axis',(0.,-0.392503506738569,0.919750508125941));
#45954=DIRECTION('',(0.,0.918216106880274,-0.396079766039157));
#45955=DIRECTION('center_axis',(1.,0.,0.));
#45956=DIRECTION('ref_axis',(0.,-0.169814459619289,0.98547605212111));
#45957=DIRECTION('',(0.,0.802123192755044,-0.597158591702786));
#45958=DIRECTION('center_axis',(1.,0.,0.));
#45959=DIRECTION('ref_axis',(0.,0.0620293289728968,0.998074327065461));
#45960=DIRECTION('',(0.,0.642787609686539,-0.766044443118978));
#45961=DIRECTION('center_axis',(1.,0.,0.));
#45962=DIRECTION('ref_axis',(0.,0.290529100384464,0.956866156695802));
#45963=DIRECTION('',(0.,0.448799180200462,-0.893632640323412));
#45964=DIRECTION('center_axis',(1.,0.,0.));
#45965=DIRECTION('ref_axis',(0.,0.503366372793645,0.8640730841431));
#45966=DIRECTION('',(0.,0.23061587074244,-0.973044870579824));
#45967=DIRECTION('center_axis',(1.,0.,0.));
#45968=DIRECTION('ref_axis',(0.,1.,0.));
#45969=DIRECTION('center_axis',(-1.,0.,0.));
#45970=DIRECTION('ref_axis',(0.,0.503366372793645,0.8640730841431));
#45971=DIRECTION('',(1.,0.,0.));
#45972=DIRECTION('',(1.,0.,0.));
#45973=DIRECTION('center_axis',(-1.,0.,0.));
#45974=DIRECTION('ref_axis',(0.,0.290529100384464,0.956866156695802));
#45975=DIRECTION('',(1.,0.,0.));
#45976=DIRECTION('',(1.,0.,0.));
#45977=DIRECTION('center_axis',(-1.,0.,0.));
#45978=DIRECTION('ref_axis',(0.,0.0620293289728968,0.998074327065461));
#45979=DIRECTION('',(1.,0.,0.));
#45980=DIRECTION('',(1.,0.,0.));
#45981=DIRECTION('center_axis',(-1.,0.,0.));
#45982=DIRECTION('ref_axis',(0.,-0.169814459619289,0.98547605212111));
#45983=DIRECTION('',(1.,0.,0.));
#45984=DIRECTION('',(1.,0.,0.));
#45985=DIRECTION('center_axis',(-1.,0.,0.));
#45986=DIRECTION('ref_axis',(0.,-0.392503506738569,0.919750508125941));
#45987=DIRECTION('',(1.,0.,0.));
#45988=DIRECTION('',(1.,0.,0.));
#45989=DIRECTION('center_axis',(-1.,0.,0.));
#45990=DIRECTION('ref_axis',(0.,-0.594032588213822,0.804440976169158));
#45991=DIRECTION('',(1.,0.,0.));
#45992=DIRECTION('',(1.,0.,0.));
#45993=DIRECTION('center_axis',(-1.,0.,0.));
#45994=DIRECTION('ref_axis',(0.,-0.763537219098866,0.645763822965308));
#45995=DIRECTION('',(1.,0.,0.));
#45996=DIRECTION('',(1.,0.,0.));
#45997=DIRECTION('center_axis',(-1.,0.,0.));
#45998=DIRECTION('ref_axis',(0.,-0.891879360868045,0.452273374915667));
#45999=DIRECTION('',(1.,0.,0.));
#46000=DIRECTION('',(1.,0.,0.));
#46001=DIRECTION('center_axis',(-1.,0.,0.));
#46002=DIRECTION('ref_axis',(0.,-0.972140055438462,0.234400752157718));
#46003=DIRECTION('',(1.,0.,0.));
#46004=DIRECTION('',(1.,0.,0.));
#46005=DIRECTION('center_axis',(-1.,0.,0.));
#46006=DIRECTION('ref_axis',(0.,-0.999992427991116,0.00389152417857752));
#46007=DIRECTION('',(1.,0.,0.));
#46008=DIRECTION('',(1.,0.,0.));
#46009=DIRECTION('center_axis',(-1.,0.,0.));
#46010=DIRECTION('ref_axis',(0.,-0.973934949912377,-0.226827496876316));
#46011=DIRECTION('',(1.,0.,0.));
#46012=DIRECTION('',(1.,0.,0.));
#46013=DIRECTION('center_axis',(-1.,0.,0.));
#46014=DIRECTION('ref_axis',(0.,-0.895372386590195,-0.445318188862501));
#46015=DIRECTION('',(1.,0.,0.));
#46016=DIRECTION('',(1.,0.,0.));
#46017=DIRECTION('center_axis',(-1.,0.,0.));
#46018=DIRECTION('ref_axis',(0.,-0.768540066148433,-0.639801662020788));
#46019=DIRECTION('',(1.,0.,0.));
#46020=DIRECTION('',(1.,0.,0.));
#46021=DIRECTION('center_axis',(-1.,0.,0.));
#46022=DIRECTION('ref_axis',(0.,-0.600275551811428,-0.799793261973046));
#46023=DIRECTION('',(1.,0.,0.));
#46024=DIRECTION('',(1.,0.,0.));
#46025=DIRECTION('center_axis',(-1.,0.,0.));
#46026=DIRECTION('ref_axis',(0.,-0.399650027100731,-0.91666780015357));
#46027=DIRECTION('',(1.,0.,0.));
#46028=DIRECTION('',(1.,0.,0.));
#46029=DIRECTION('center_axis',(-1.,0.,0.));
#46030=DIRECTION('ref_axis',(0.,-0.177479265983482,-0.984124539957197));
#46031=DIRECTION('',(1.,0.,0.));
#46032=DIRECTION('',(1.,0.,0.));
#46033=DIRECTION('center_axis',(-1.,0.,0.));
#46034=DIRECTION('ref_axis',(0.,0.0542594483017311,-0.998526871080589));
#46035=DIRECTION('',(1.,0.,0.));
#46036=DIRECTION('',(1.,0.,0.));
#46037=DIRECTION('center_axis',(-1.,0.,0.));
#46038=DIRECTION('ref_axis',(0.,0.283073021684467,-0.95909836012498));
#46039=DIRECTION('',(1.,0.,0.));
#46040=DIRECTION('',(1.,0.,0.));
#46041=DIRECTION('center_axis',(-1.,0.,0.));
#46042=DIRECTION('ref_axis',(0.,0.496626055197469,-0.867964608321676));
#46043=DIRECTION('',(1.,0.,0.));
#46044=DIRECTION('',(1.,0.,0.));
#46045=DIRECTION('center_axis',(-1.,0.,0.));
#46046=DIRECTION('ref_axis',(0.,0.683405849527915,-0.730038659819485));
#46047=DIRECTION('',(1.,0.,0.));
#46048=DIRECTION('',(1.,0.,0.));
#46049=DIRECTION('center_axis',(-1.,0.,0.));
#46050=DIRECTION('ref_axis',(0.,0.833343057617297,-0.552756138202965));
#46051=DIRECTION('',(1.,0.,0.));
#46052=DIRECTION('',(1.,0.,0.));
#46053=DIRECTION('center_axis',(-1.,0.,0.));
#46054=DIRECTION('ref_axis',(0.,0.938354525767724,-0.345674390100322));
#46055=DIRECTION('',(1.,0.,0.));
#46056=DIRECTION('',(1.,0.,0.));
#46057=DIRECTION('center_axis',(1.,0.,0.));
#46058=DIRECTION('ref_axis',(0.,0.0999066712465393,0.994996812578028));
#46059=DIRECTION('center_axis',(1.,0.,0.));
#46060=DIRECTION('ref_axis',(0.,4.55191440096314E-15,1.));
#46061=DIRECTION('center_axis',(1.,0.,0.));
#46062=DIRECTION('ref_axis',(0.,1.,0.));
#46063=DIRECTION('center_axis',(-1.,0.,0.));
#46064=DIRECTION('ref_axis',(0.,-1.,3.06161699786838E-17));
#46065=DIRECTION('center_axis',(-1.,0.,0.));
#46066=DIRECTION('ref_axis',(0.,-1.,3.06161699786838E-17));
#46067=DIRECTION('center_axis',(-1.,0.,0.));
#46068=DIRECTION('ref_axis',(0.,0.992779058549995,-0.119957246152893));
#46069=DIRECTION('',(1.,0.,0.));
#46070=DIRECTION('',(1.,0.,0.));
#46071=DIRECTION('center_axis',(1.,0.,0.));
#46072=DIRECTION('ref_axis',(0.,0.689067033753993,-0.724697607967264));
#46073=DIRECTION('',(1.,0.,0.));
#46074=DIRECTION('',(1.,0.,0.));
#46075=DIRECTION('center_axis',(-1.,0.,0.));
#46076=DIRECTION('ref_axis',(0.,0.993682615314554,0.112226823984413));
#46077=DIRECTION('',(1.,0.,0.));
#46078=DIRECTION('',(1.,0.,0.));
#46079=DIRECTION('center_axis',(1.,0.,0.));
#46080=DIRECTION('ref_axis',(0.,0.,-1.));
#46081=DIRECTION('center_axis',(0.,-1.,-1.22464679914735E-16));
#46082=DIRECTION('ref_axis',(0.,-1.22464679914735E-16,1.));
#46083=DIRECTION('center_axis',(1.,0.,0.));
#46084=DIRECTION('ref_axis',(0.,-1.,1.83697019872103E-16));
#46085=DIRECTION('center_axis',(-1.,0.,0.));
#46086=DIRECTION('ref_axis',(0.,0.,1.));
#46087=DIRECTION('center_axis',(-1.,0.,0.));
#46088=DIRECTION('ref_axis',(0.,1.,0.));
#46089=DIRECTION('center_axis',(-1.,0.,0.));
#46090=DIRECTION('ref_axis',(0.,0.941016485082348,0.338360716991886));
#46091=DIRECTION('',(1.,0.,0.));
#46092=DIRECTION('',(1.,0.,0.));
#46093=DIRECTION('center_axis',(-1.,0.,0.));
#46094=DIRECTION('ref_axis',(0.,1.,0.));
#46095=DIRECTION('center_axis',(1.,0.,0.));
#46096=DIRECTION('ref_axis',(0.,1.,0.));
#46097=DIRECTION('center_axis',(0.,-1.22464679914735E-16,1.));
#46098=DIRECTION('ref_axis',(0.,-1.,-1.22464679914735E-16));
#46099=DIRECTION('center_axis',(1.,0.,0.));
#46100=DIRECTION('ref_axis',(0.,1.,0.));
#46101=DIRECTION('',(1.,0.,0.));
#46102=DIRECTION('center_axis',(1.,0.,0.));
#46103=DIRECTION('ref_axis',(0.,0.,-1.));
#46104=DIRECTION('center_axis',(1.,0.,0.));
#46105=DIRECTION('ref_axis',(-2.75667434231801E-17,0.888918026944739,0.458066306742455));
#46106=DIRECTION('center_axis',(-1.,0.,0.));
#46107=DIRECTION('ref_axis',(0.,1.,0.));
#46108=DIRECTION('',(0.514495755427526,0.857492925712544,1.05012596676537E-16));
#46109=DIRECTION('center_axis',(0.,-0.973044870579824,0.23061587074244));
#46110=DIRECTION('ref_axis',(0.,-0.23061587074244,-0.973044870579824));
#46111=DIRECTION('center_axis',(0.,-0.893632640323412,0.448799180200462));
#46112=DIRECTION('ref_axis',(0.,-0.448799180200462,-0.893632640323412));
#46113=DIRECTION('center_axis',(0.,-0.766044443118978,0.64278760968654));
#46114=DIRECTION('ref_axis',(0.,-0.64278760968654,-0.766044443118978));
#46115=DIRECTION('center_axis',(0.,-0.597158591702786,0.802123192755044));
#46116=DIRECTION('ref_axis',(0.,-0.802123192755044,-0.597158591702786));
#46117=DIRECTION('center_axis',(0.,-0.396079766039157,0.918216106880274));
#46118=DIRECTION('ref_axis',(0.,-0.918216106880274,-0.396079766039157));
#46119=DIRECTION('center_axis',(0.,-0.17364817766693,0.984807753012208));
#46120=DIRECTION('ref_axis',(0.,-0.984807753012208,-0.17364817766693));
#46121=DIRECTION('center_axis',(0.,0.0581448289104762,0.998308158271268));
#46122=DIRECTION('ref_axis',(0.,-0.998308158271268,0.0581448289104762));
#46123=DIRECTION('center_axis',(0.,0.286803232711091,0.957989512315489));
#46124=DIRECTION('ref_axis',(0.,-0.957989512315489,0.286803232711091));
#46125=DIRECTION('center_axis',(0.,0.5,0.866025403784438));
#46126=DIRECTION('ref_axis',(0.,-0.866025403784438,0.5));
#46127=DIRECTION('center_axis',(0.,0.686241637868734,0.727373641573049));
#46128=DIRECTION('ref_axis',(0.,-0.727373641573049,0.686241637868734));
#46129=DIRECTION('center_axis',(0.,0.835487811412936,0.549508978070806));
#46130=DIRECTION('ref_axis',(0.,-0.549508978070806,0.835487811412936));
#46131=DIRECTION('center_axis',(0.,0.939692620785908,0.342020143325669));
#46132=DIRECTION('ref_axis',(0.,-0.342020143325669,0.939692620785909));
#46133=DIRECTION('center_axis',(0.,0.993238357741943,0.11609291412523));
#46134=DIRECTION('ref_axis',(0.,-0.11609291412523,0.993238357741943));
#46135=DIRECTION('center_axis',(0.,0.993238357741943,-0.11609291412523));
#46136=DIRECTION('ref_axis',(0.,0.11609291412523,0.993238357741943));
#46137=DIRECTION('center_axis',(0.,0.939692620785908,-0.342020143325669));
#46138=DIRECTION('ref_axis',(0.,0.342020143325669,0.939692620785908));
#46139=DIRECTION('center_axis',(0.,0.835487811412936,-0.549508978070806));
#46140=DIRECTION('ref_axis',(0.,0.549508978070806,0.835487811412936));
#46141=DIRECTION('center_axis',(0.,0.686241637868733,-0.727373641573049));
#46142=DIRECTION('ref_axis',(0.,0.727373641573049,0.686241637868733));
#46143=DIRECTION('center_axis',(0.,0.5,-0.866025403784439));
#46144=DIRECTION('ref_axis',(0.,0.866025403784439,0.5));
#46145=DIRECTION('center_axis',(0.,0.28680323271109,-0.957989512315489));
#46146=DIRECTION('ref_axis',(0.,0.957989512315489,0.28680323271109));
#46147=DIRECTION('center_axis',(0.,0.0581448289104758,-0.998308158271268));
#46148=DIRECTION('ref_axis',(0.,0.998308158271268,0.0581448289104758));
#46149=DIRECTION('center_axis',(0.,-0.17364817766693,-0.984807753012208));
#46150=DIRECTION('ref_axis',(0.,0.984807753012208,-0.17364817766693));
#46151=DIRECTION('center_axis',(0.,-0.396079766039157,-0.918216106880274));
#46152=DIRECTION('ref_axis',(0.,0.918216106880274,-0.396079766039157));
#46153=DIRECTION('center_axis',(0.,-0.597158591702786,-0.802123192755044));
#46154=DIRECTION('ref_axis',(0.,0.802123192755044,-0.597158591702786));
#46155=DIRECTION('center_axis',(0.,-0.766044443118978,-0.642787609686539));
#46156=DIRECTION('ref_axis',(0.,0.642787609686539,-0.766044443118978));
#46157=DIRECTION('center_axis',(0.,-0.893632640323412,-0.448799180200462));
#46158=DIRECTION('ref_axis',(0.,0.448799180200462,-0.893632640323412));
#46159=DIRECTION('center_axis',(0.,-0.973044870579824,-0.23061587074244));
#46160=DIRECTION('ref_axis',(0.,0.23061587074244,-0.973044870579824));
#46161=DIRECTION('center_axis',(0.,-1.,0.));
#46162=DIRECTION('ref_axis',(0.,0.,-1.));
#46163=DIRECTION('center_axis',(0.560848145169515,0.413959345244165,-0.716998618230842));
#46164=DIRECTION('ref_axis',(-0.827918690488332,0.280424072584757,-0.485708741382183));
#46165=DIRECTION('center_axis',(-0.560848145169515,-0.413959345244165,0.716998618230842));
#46166=DIRECTION('ref_axis',(-0.827918690488332,0.280424072584757,-0.485708741382183));
#46167=DIRECTION('center_axis',(6.01305526018457E-17,-0.866025403784439,
-0.499999999999999));
#46168=DIRECTION('ref_axis',(-1.,-5.20745860967949E-17,-3.00652763009228E-17));
#46169=DIRECTION('center_axis',(1.,0.,0.));
#46170=DIRECTION('ref_axis',(0.,1.,0.));
#46171=DIRECTION('center_axis',(0.560848145169515,0.413959345244166,0.716998618230841));
#46172=DIRECTION('ref_axis',(-0.827918690488332,0.280424072584758,0.485708741382183));
#46173=DIRECTION('center_axis',(0.560848145169515,0.827918690488332,4.32978028117747E-17));
#46174=DIRECTION('ref_axis',(-0.827918690488332,0.560848145169515,-4.91959218075756E-17));
#46175=DIRECTION('center_axis',(1.,0.,0.));
#46176=DIRECTION('ref_axis',(0.,1.,0.));
#57283=CARTESIAN_POINT('',(0.,0.,0.));
#57284=CARTESIAN_POINT('Origin',(21.9,0.,0.));
#57285=CARTESIAN_POINT('',(1.2076868253652,-10.9259358523014,-1.30115088740845E-5));
#57286=CARTESIAN_POINT('',(1.13921356237308,-10.925,-1.33792662806848E-15));
#57287=CARTESIAN_POINT('',(21.9,-10.925,-1.33792662806848E-15));
#57288=CARTESIAN_POINT('',(1.13921356237309,-10.477856724544,3.0906144932497));
#57289=CARTESIAN_POINT('Ctrl Pts',(1.2076868253652,-10.9259358975192,-1.30121375534478E-5));
#57290=CARTESIAN_POINT('Ctrl Pts',(1.18486240436783,-10.9258624043912,1.04421041974912));
#57291=CARTESIAN_POINT('Ctrl Pts',(1.16203798337046,-10.7729788146462,2.08845452903323));
#57292=CARTESIAN_POINT('Ctrl Pts',(1.13921356237309,-10.477856724544,3.0906144932497));
#57293=CARTESIAN_POINT('Origin',(1.13921356237308,0.,0.));
#57294=CARTESIAN_POINT('Origin',(21.9,0.,0.));
#57295=CARTESIAN_POINT('',(2.7076868253652,-10.924189479016,-0.000147560072731594));
#57296=CARTESIAN_POINT('',(2.4923131746348,-10.9255938614398,-0.000203849024224443));
#57297=CARTESIAN_POINT('',(21.9,-10.925,-1.33792662806848E-15));
#57298=CARTESIAN_POINT('Ctrl Pts',(2.7076868253652,-10.924189479016,-0.000147560072731594));
#57299=CARTESIAN_POINT('Ctrl Pts',(2.68421200161813,-10.9236770875182,1.07432675973471));
#57300=CARTESIAN_POINT('Ctrl Pts',(2.66073717787106,-10.7662229664806,2.14894800679005));
#57301=CARTESIAN_POINT('Ctrl Pts',(2.63726235412399,-10.4539812700227,3.17653566527511));
#57302=CARTESIAN_POINT('Ctrl Pts',(2.59757431317426,-9.92608545411549,4.91384119347891));
#57303=CARTESIAN_POINT('Ctrl Pts',(2.55788627222453,-8.95575334874734,6.51670849981278));
#57304=CARTESIAN_POINT('Ctrl Pts',(2.5181982312748,-7.6611825544693,7.78988992812834));
#57305=CARTESIAN_POINT('Ctrl Pts',(2.47851019032507,-6.36661176019123,9.06307135644392));
#57306=CARTESIAN_POINT('Ctrl Pts',(2.43882214937534,-4.74780227700327,10.0065669067412));
#57307=CARTESIAN_POINT('Ctrl Pts',(2.39913410842561,-3.00194370123965,10.5054479791454));
#57308=CARTESIAN_POINT('Ctrl Pts',(2.35944606747588,-1.25608512547604,11.0043290515496));
#57309=CARTESIAN_POINT('Ctrl Pts',(2.31975802652615,0.616822542863241,11.0585956460607));
#57310=CARTESIAN_POINT('Ctrl Pts',(2.28006998557642,2.38863762787762,10.6616374683763));
#57311=CARTESIAN_POINT('Ctrl Pts',(2.24038194462669,4.16045271289198,10.264679290692));
#57312=CARTESIAN_POINT('Ctrl Pts',(2.20069390367696,5.83117521458145,9.4164963408121));
#57313=CARTESIAN_POINT('Ctrl Pts',(2.16100586272722,7.19729193517843,8.2204070474781));
#57314=CARTESIAN_POINT('Ctrl Pts',(2.12131782177749,8.56340865577541,7.02431775414409));
#57315=CARTESIAN_POINT('Ctrl Pts',(2.08162978082776,9.62491959527989,5.48032211735595));
#57316=CARTESIAN_POINT('Ctrl Pts',(2.04194173987803,10.2525205215885,3.77649654934429));
#57317=CARTESIAN_POINT('Ctrl Pts',(2.0022536989283,10.8801214478971,2.07267098133261));
#57318=CARTESIAN_POINT('Ctrl Pts',(1.96256565797857,11.0738123610098,0.20901548209741));
#57319=CARTESIAN_POINT('Ctrl Pts',(1.92287761702884,10.8099994858353,-1.58745529696239));
#57320=CARTESIAN_POINT('Ctrl Pts',(1.88318957607911,10.5461866106608,-3.38392607602218));
#57321=CARTESIAN_POINT('Ctrl Pts',(1.84350153512938,9.82486994719908,-5.11321213490657));
#57322=CARTESIAN_POINT('Ctrl Pts',(1.80381349417965,8.73391414627591,-6.56466655392927));
#57323=CARTESIAN_POINT('Ctrl Pts',(1.76412545322992,7.64295834535273,-8.01612097295197));
#57324=CARTESIAN_POINT('Ctrl Pts',(1.72443741228019,6.18236340696808,-9.18974375211298));
#57325=CARTESIAN_POINT('Ctrl Pts',(1.68474937133046,4.53004659234707,-9.94257416385729));
#57326=CARTESIAN_POINT('Ctrl Pts',(1.64506133038073,2.87772977772604,-10.6954045756016));
#57327=CARTESIAN_POINT('Ctrl Pts',(1.605373289431,1.03369108686863,-11.0274426199292));
#57328=CARTESIAN_POINT('Ctrl Pts',(1.56568524848127,-0.777444405467683,
-10.8982422226886));
#57329=CARTESIAN_POINT('Ctrl Pts',(1.52599720753154,-2.58857989780399,-10.769041825448));
#57330=CARTESIAN_POINT('Ctrl Pts',(1.48630916658181,-4.36681219161921,-10.1786029866393));
#57331=CARTESIAN_POINT('Ctrl Pts',(1.44662112563208,-5.89553210708439,-9.19884798966945));
#57332=CARTESIAN_POINT('Ctrl Pts',(1.40693308468235,-7.42425202254956,-8.21909299269962));
#57333=CARTESIAN_POINT('Ctrl Pts',(1.36724504373261,-8.7034595596647,-6.85002183756871));
#57334=CARTESIAN_POINT('Ctrl Pts',(1.32755700278288,-9.57733264350962,-5.25840302976058));
#57335=CARTESIAN_POINT('Ctrl Pts',(1.28786896183315,-10.4512057273545,-3.66678422195244));
#57336=CARTESIAN_POINT('Ctrl Pts',(1.24818092088342,-10.9197443579293,-1.85261776146706));
#57337=CARTESIAN_POINT('Ctrl Pts',(1.20849287993369,-10.9258749484534,-0.0368901493056266));
#57338=CARTESIAN_POINT('Ctrl Pts',(1.20822419507753,-10.9259164520598,-0.0245978189050059));
#57339=CARTESIAN_POINT('Ctrl Pts',(1.20795551022136,-10.9259367626667,-0.0123054169539716));
#57340=CARTESIAN_POINT('Ctrl Pts',(1.2076868253652,-10.9259358975192,-1.30121375534478E-5));
#57341=CARTESIAN_POINT('',(1.13921356237308,-8.9203904128527,-6.3056746902777));
#57342=CARTESIAN_POINT('Origin',(1.13921356237308,0.,0.));
#57343=CARTESIAN_POINT('Ctrl Pts',(1.13921356237308,-8.920390421998,-6.30567469743328));
#57344=CARTESIAN_POINT('Ctrl Pts',(1.15944494044868,-8.38580517885053,-7.06185389348771));
#57345=CARTESIAN_POINT('Ctrl Pts',(1.17967631852427,-7.75612190636329,-7.75083412086764));
#57346=CARTESIAN_POINT('Ctrl Pts',(1.19990769659986,-7.04892226234213,-8.34799640854694));
#57347=CARTESIAN_POINT('Ctrl Pts',(1.23950937525994,-5.6646224412225,-9.51690487025583));
#57348=CARTESIAN_POINT('Ctrl Pts',(1.27911105392001,-3.98331356209647,-10.3340068781933));
#57349=CARTESIAN_POINT('Ctrl Pts',(1.31871273258009,-2.20893546975469,-10.7002922971518));
#57350=CARTESIAN_POINT('Ctrl Pts',(1.35831441124016,-0.434557377412914,
-11.0665777161103));
#57351=CARTESIAN_POINT('Ctrl Pts',(1.39791608990024,1.43288992814462,-10.9820465460897));
#57352=CARTESIAN_POINT('Ctrl Pts',(1.43751776856032,3.16690298535677,-10.4569008854534));
#57353=CARTESIAN_POINT('Ctrl Pts',(1.47711944722039,4.90091604256891,-9.93175522481722));
#57354=CARTESIAN_POINT('Ctrl Pts',(1.51672112588047,6.50149485143568,-8.96599507356536));
#57355=CARTESIAN_POINT('Ctrl Pts',(1.55632280454054,7.77449813483008,-7.67678664514963));
#57356=CARTESIAN_POINT('Ctrl Pts',(1.59592448320062,9.04750141822449,-6.38757821673391));
#57357=CARTESIAN_POINT('Ctrl Pts',(1.63552616186069,9.99292917614654,-4.77492151115431));
#57358=CARTESIAN_POINT('Ctrl Pts',(1.67512784052077,10.4961089711804,-3.03440671920132));
#57359=CARTESIAN_POINT('Ctrl Pts',(1.71472951918085,10.9992887662142,-1.29389192724834));
#57360=CARTESIAN_POINT('Ctrl Pts',(1.75433119784092,11.0602205983598,0.574480951078047));
#57361=CARTESIAN_POINT('Ctrl Pts',(1.793932876501,10.671513222116,2.3440844709801));
#57362=CARTESIAN_POINT('Ctrl Pts',(1.83353455516107,10.2828058458723,4.11368799088217));
#57363=CARTESIAN_POINT('Ctrl Pts',(1.87313623382115,9.44445926123903,5.78452215235991));
#57364=CARTESIAN_POINT('Ctrl Pts',(1.91273791248123,8.25815930120191,7.15393026676788));
#57365=CARTESIAN_POINT('Ctrl Pts',(1.9523395911413,7.0718593411648,8.52333838117585));
#57366=CARTESIAN_POINT('Ctrl Pts',(1.99194126980138,5.5376060057238,9.59132044851404));
#57367=CARTESIAN_POINT('Ctrl Pts',(2.03154294846145,3.84149317676308,10.2283359235612));
#57368=CARTESIAN_POINT('Ctrl Pts',(2.07114462712153,2.14538034780235,10.8653513986085));
#57369=CARTESIAN_POINT('Ctrl Pts',(2.11074630578161,0.287408025321914,11.0714002813647));
#57370=CARTESIAN_POINT('Ctrl Pts',(2.15034798444168,-1.50706482753928,10.8214912810367));
#57371=CARTESIAN_POINT('Ctrl Pts',(2.18994966310176,-3.30153768040048,10.5715822807087));
#57372=CARTESIAN_POINT('Ctrl Pts',(2.22955134176183,-5.03251106364243,9.86571539729656));
#57373=CARTESIAN_POINT('Ctrl Pts',(2.26915302042191,-6.49003022120965,8.7895067743812));
#57374=CARTESIAN_POINT('Ctrl Pts',(2.30875469908198,-7.94754937877685,7.71329815146585));
#57375=CARTESIAN_POINT('Ctrl Pts',(2.34835637774206,-9.13161431066935,6.26674778904728));
#57376=CARTESIAN_POINT('Ctrl Pts',(2.38795805640214,-9.89860630920593,4.62531225506919));
#57377=CARTESIAN_POINT('Ctrl Pts',(2.42274309581303,-10.5723112580779,3.18351984445045));
#57378=CARTESIAN_POINT('Ctrl Pts',(2.45752813522391,-10.924228228766,1.59136594949956));
#57379=CARTESIAN_POINT('Ctrl Pts',(2.4923131746348,-10.9255938614398,-0.000203849024224443));
#57380=CARTESIAN_POINT('Origin',(21.9,0.,0.));
#57381=CARTESIAN_POINT('',(4.20768682536519,-10.9252346746171,0.00026931280733642));
#57382=CARTESIAN_POINT('',(3.99231317463481,-10.9240736852168,-6.866552131629E-6));
#57383=CARTESIAN_POINT('',(21.9,-10.925,-1.33792662806848E-15));
#57384=CARTESIAN_POINT('Ctrl Pts',(4.20768682536519,-10.9252346746171,0.00026931280733642));
#57385=CARTESIAN_POINT('Ctrl Pts',(4.20015653396462,-10.9255870687535,0.344846207711655));
#57386=CARTESIAN_POINT('Ctrl Pts',(4.19262624256405,-10.9096073684142,0.689390550044324));
#57387=CARTESIAN_POINT('Ctrl Pts',(4.18509595116348,-10.87705529884,1.03236197733682));
#57388=CARTESIAN_POINT('Ctrl Pts',(4.14540791021375,-10.7054911718317,2.83997649407921));
#57389=CARTESIAN_POINT('Ctrl Pts',(4.10571986926402,-10.0735852992404,4.60389910141565));
#57390=CARTESIAN_POINT('Ctrl Pts',(4.06603182831429,-9.05831107750627,6.10926375673875));
#57391=CARTESIAN_POINT('Ctrl Pts',(4.02634378736457,-8.04303685577212,7.61462841206186));
#57392=CARTESIAN_POINT('Ctrl Pts',(3.98665574641483,-6.64439428489504,8.86143511537164));
#57393=CARTESIAN_POINT('Ctrl Pts',(3.9469677054651,-5.0327541016504,9.69780848329121));
#57394=CARTESIAN_POINT('Ctrl Pts',(3.90727966451537,-3.42111391840574,10.5341818512108));
#57395=CARTESIAN_POINT('Ctrl Pts',(3.86759162356564,-1.59647612279351,10.9601218837401));
#57396=CARTESIAN_POINT('Ctrl Pts',(3.82790358261591,0.218897434975739,10.9237441904887));
#57397=CARTESIAN_POINT('Ctrl Pts',(3.78821554166618,2.03427099274499,10.8873664972373));
#57398=CARTESIAN_POINT('Ctrl Pts',(3.74852750071645,3.84038031267128,10.388671078205));
#57399=CARTESIAN_POINT('Ctrl Pts',(3.70883945976672,5.4172205257909,9.4884047658826));
#57400=CARTESIAN_POINT('Ctrl Pts',(3.66915141881698,6.99406073891051,8.58813845356016));
#57401=CARTESIAN_POINT('Ctrl Pts',(3.62946337786726,8.34163184522347,7.2863012479475));
#57402=CARTESIAN_POINT('Ctrl Pts',(3.58977533691753,9.29578419919515,5.74147187995093));
#57403=CARTESIAN_POINT('Ctrl Pts',(3.5500872959678,10.2499365531668,4.19664251195437));
#57404=CARTESIAN_POINT('Ctrl Pts',(3.51039925501806,10.8106701547972,2.4088209815739));
#57405=CARTESIAN_POINT('Ctrl Pts',(3.47071121406833,10.9096812080811,0.595784494864098));
#57406=CARTESIAN_POINT('Ctrl Pts',(3.4310231731186,11.0086922613649,-1.2172519918457));
#57407=CARTESIAN_POINT('Ctrl Pts',(3.39133513216887,10.6459807663023,-3.05550343488481));
#57408=CARTESIAN_POINT('Ctrl Pts',(3.35164709121914,9.86572915086958,-4.69504968535445));
#57409=CARTESIAN_POINT('Ctrl Pts',(3.31195905026941,9.08547753543687,-6.33459593582411));
#57410=CARTESIAN_POINT('Ctrl Pts',(3.27227100931968,7.88768579963414,-7.77543699372428));
#57411=CARTESIAN_POINT('Ctrl Pts',(3.23258296836995,6.41825874056784,-8.84206186165975));
#57412=CARTESIAN_POINT('Ctrl Pts',(3.19289492742022,4.94883168150154,-9.90868672959523));
#57413=CARTESIAN_POINT('Ctrl Pts',(3.15320688647049,3.20776929917166,-10.601095407566));
#57414=CARTESIAN_POINT('Ctrl Pts',(3.11351884552076,1.40715299810077,-10.8349445622108));
#57415=CARTESIAN_POINT('Ctrl Pts',(3.07383080457103,-0.39346330297011,-11.0687937168556));
#57416=CARTESIAN_POINT('Ctrl Pts',(3.0341427636213,-2.25363352278201,-10.8440833481744));
#57417=CARTESIAN_POINT('Ctrl Pts',(2.99445472267157,-3.94676755356788,-10.1881857611846));
#57418=CARTESIAN_POINT('Ctrl Pts',(2.95476668172184,-5.63990158435378,-9.53228817419476));
#57419=CARTESIAN_POINT('Ctrl Pts',(2.91507864077211,-7.16599942611365,-8.44520336889632));
#57420=CARTESIAN_POINT('Ctrl Pts',(2.87539059982238,-8.33916482548504,-7.05935076616014));
#57421=CARTESIAN_POINT('Ctrl Pts',(2.83570255887265,-9.5123302248564,-5.67349816342398));
#57422=CARTESIAN_POINT('Ctrl Pts',(2.79601451792291,-10.3325631818393,-3.98887776325009));
#57423=CARTESIAN_POINT('Ctrl Pts',(2.75632647697318,-10.6999498971076,-2.21069568812629));
#57424=CARTESIAN_POINT('Ctrl Pts',(2.74011325977052,-10.850033410163,-1.48427907697687));
#57425=CARTESIAN_POINT('Ctrl Pts',(2.72390004256786,-10.9245433694109,-0.742248361911372));
#57426=CARTESIAN_POINT('Ctrl Pts',(2.7076868253652,-10.924189479016,-0.000147560072731594));
#57427=CARTESIAN_POINT('Ctrl Pts',(2.4923131746348,-10.9255938614398,-0.000203849024224443));
#57428=CARTESIAN_POINT('Ctrl Pts',(2.49712981388399,-10.9257829588233,-0.220586452845366));
#57429=CARTESIAN_POINT('Ctrl Pts',(2.50194645313318,-10.9192507316004,-0.440957857446129));
#57430=CARTESIAN_POINT('Ctrl Pts',(2.50676309238236,-10.90592081475,-0.660917311227143));
#57431=CARTESIAN_POINT('Ctrl Pts',(2.54636477104244,-10.7963242565768,-2.46939063800773));
#57432=CARTESIAN_POINT('Ctrl Pts',(2.58596644970252,-10.2272120750497,-4.25001658603124));
#57433=CARTESIAN_POINT('Ctrl Pts',(2.62556812836259,-9.26761353754808,-5.7868177785457));
#57434=CARTESIAN_POINT('Ctrl Pts',(2.66516980702267,-8.30801500004645,-7.32361897106015));
#57435=CARTESIAN_POINT('Ctrl Pts',(2.70477148568274,-6.95793010657029,-8.61659540806554));
#57436=CARTESIAN_POINT('Ctrl Pts',(2.74437316434282,-5.38111458874416,-9.50891824856789));
#57437=CARTESIAN_POINT('Ctrl Pts',(2.7839748430029,-3.80429907091803,-10.4012410890702));
#57438=CARTESIAN_POINT('Ctrl Pts',(2.82357652166298,-2.00075292874194,-10.8929103330696));
#57439=CARTESIAN_POINT('Ctrl Pts',(2.86317820032305,-0.189233524170143,
-10.9242899673815));
#57440=CARTESIAN_POINT('Ctrl Pts',(2.90277987898313,1.62228588040165,-10.9556696016935));
#57441=CARTESIAN_POINT('Ctrl Pts',(2.9423815576432,3.44177854736914,-10.5267596263181));
#57442=CARTESIAN_POINT('Ctrl Pts',(2.98198323630328,5.0485529117372,-9.68958379091988));
#57443=CARTESIAN_POINT('Ctrl Pts',(3.02158491496335,6.65532727610525,-8.85240795552168));
#57444=CARTESIAN_POINT('Ctrl Pts',(3.06118659362343,8.04938333787388,-7.60696626010066));
#57445=CARTESIAN_POINT('Ctrl Pts',(3.1007882722835,9.06163197815398,-6.10432194970029));
#57446=CARTESIAN_POINT('Ctrl Pts',(3.14038995094358,10.0738806184341,-4.60167763929991));
#57447=CARTESIAN_POINT('Ctrl Pts',(3.17999162960366,10.7043218372256,-2.84183071392017));
#57448=CARTESIAN_POINT('Ctrl Pts',(3.21959330826373,10.8764875829607,-1.03823813457975));
#57449=CARTESIAN_POINT('Ctrl Pts',(3.25919498692381,11.0486533286959,0.765354444760677));
#57450=CARTESIAN_POINT('Ctrl Pts',(3.29879666558388,10.7625436013745,2.61269267806179));
#57451=CARTESIAN_POINT('Ctrl Pts',(3.33839834424396,10.0528614831245,4.27970753273771));
#57452=CARTESIAN_POINT('Ctrl Pts',(3.37800002290404,9.34317936487456,5.94672238741363));
#57453=CARTESIAN_POINT('Ctrl Pts',(3.41760170156411,8.20992485569591,7.43341386346435));
#57454=CARTESIAN_POINT('Ctrl Pts',(3.45720338022419,6.7905536950832,8.55945682168118));
#57455=CARTESIAN_POINT('Ctrl Pts',(3.49680505888426,5.37118253447051,9.68549977989799));
#57456=CARTESIAN_POINT('Ctrl Pts',(3.53640673754434,3.66569472242377,10.4508942202809));
#57457=CARTESIAN_POINT('Ctrl Pts',(3.57600841620441,1.88095384223483,10.7628032226187));
#57458=CARTESIAN_POINT('Ctrl Pts',(3.61561009486449,0.0962129620458729,
11.0747122249566));
#57459=CARTESIAN_POINT('Ctrl Pts',(3.65521177352457,-1.7677809862853,10.9331357892493));
#57460=CARTESIAN_POINT('Ctrl Pts',(3.69481345218464,-3.48493874866277,10.3552461334805));
#57461=CARTESIAN_POINT('Ctrl Pts',(3.73441513084472,-5.20209651104025,9.77735647771168));
#57462=CARTESIAN_POINT('Ctrl Pts',(3.77401680950479,-6.77241808746404,8.76315360188128));
#57463=CARTESIAN_POINT('Ctrl Pts',(3.81361848816487,-8.00543460100157,7.43565312634651));
#57464=CARTESIAN_POINT('Ctrl Pts',(3.85322016682494,-9.23845111453912,6.10815265081174));
#57465=CARTESIAN_POINT('Ctrl Pts',(3.89282184548502,-10.1341625651904,4.46735457557259));
#57466=CARTESIAN_POINT('Ctrl Pts',(3.9324235241451,-10.5839255027173,2.71227607727802));
#57467=CARTESIAN_POINT('Ctrl Pts',(3.952386740975,-10.8106511201078,1.82754053574464));
#57468=CARTESIAN_POINT('Ctrl Pts',(3.9723499578049,-10.9240536033779,0.913764386768712));
#57469=CARTESIAN_POINT('Ctrl Pts',(3.99231317463481,-10.9240736852168,-6.866552131629E-6));
#57470=CARTESIAN_POINT('Origin',(21.9,0.,0.));
#57471=CARTESIAN_POINT('',(5.70768682536519,-10.9251067326884,-0.000279136740874882));
#57472=CARTESIAN_POINT('',(5.49231317463481,-10.9255540795388,0.000213857475631818));
#57473=CARTESIAN_POINT('',(21.9,-10.925,-1.33792662806848E-15));
#57474=CARTESIAN_POINT('Ctrl Pts',(5.70768682536519,-10.9251067326884,-0.000279136740874882));
#57475=CARTESIAN_POINT('Ctrl Pts',(5.67641302536139,-10.9236290933278,1.43081987113484));
#57476=CARTESIAN_POINT('Ctrl Pts',(5.64513922535759,-10.640931556177,2.86248539651479));
#57477=CARTESIAN_POINT('Ctrl Pts',(5.61386542535379,-10.0929987767102,4.18419393905209));
#57478=CARTESIAN_POINT('Ctrl Pts',(5.57417738440406,-9.3976442439533,5.86150922384157));
#57479=CARTESIAN_POINT('Ctrl Pts',(5.53448934345433,-8.27513102280277,7.36173989438199));
#57480=CARTESIAN_POINT('Ctrl Pts',(5.49480130250459,-6.86219412226636,8.50214061602178));
#57481=CARTESIAN_POINT('Ctrl Pts',(5.45511326155486,-5.44925722172996,9.64254133766156));
#57482=CARTESIAN_POINT('Ctrl Pts',(5.41542522060513,-3.74589664180768,10.4231121104007));
#57483=CARTESIAN_POINT('Ctrl Pts',(5.3757371796554,-1.95960127425644,10.7487704446698));
#57484=CARTESIAN_POINT('Ctrl Pts',(5.33604913870567,-0.173305906705207,
11.0744287789389));
#57485=CARTESIAN_POINT('Ctrl Pts',(5.29636109775594,1.69592424847499,10.9451746747378));
#57486=CARTESIAN_POINT('Ctrl Pts',(5.25667305680621,3.4203954792724,10.3767527672026));
#57487=CARTESIAN_POINT('Ctrl Pts',(5.21698501585648,5.14486671006981,9.80833085966738));
#57488=CARTESIAN_POINT('Ctrl Pts',(5.17729697490675,6.72457901648443,8.80074114879795));
#57489=CARTESIAN_POINT('Ctrl Pts',(5.13760893395702,7.9671052873008,7.47671963947679));
#57490=CARTESIAN_POINT('Ctrl Pts',(5.09792089300729,9.2096315581172,6.15269813015559));
#57491=CARTESIAN_POINT('Ctrl Pts',(5.05823285205756,10.1149717933353,4.51224482238265));
#57492=CARTESIAN_POINT('Ctrl Pts',(5.01854481110783,10.5728451491441,2.75518577930683));
#57493=CARTESIAN_POINT('Ctrl Pts',(4.9788567701581,11.0307185049528,0.998126736231025));
#57494=CARTESIAN_POINT('Ctrl Pts',(4.93916872920836,11.0411249813522,-0.875538042147655));
#57495=CARTESIAN_POINT('Ctrl Pts',(4.89948068825863,10.6027969499372,-2.63757465575414));
#57496=CARTESIAN_POINT('Ctrl Pts',(4.8597926473089,10.1644689185222,-4.39961126936062));
#57497=CARTESIAN_POINT('Ctrl Pts',(4.82010460635918,9.27740637929273,-6.05001971819488));
#57498=CARTESIAN_POINT('Ctrl Pts',(4.78041656540945,8.04966374266159,-7.38776128853348));
#57499=CARTESIAN_POINT('Ctrl Pts',(4.74072852445972,6.82192110603044,-8.72550285887207));
#57500=CARTESIAN_POINT('Ctrl Pts',(4.70104048350998,5.25349837199757,-9.75057755071499));
#57501=CARTESIAN_POINT('Ctrl Pts',(4.66135244256025,3.53544745213524,-10.3381194875792));
#57502=CARTESIAN_POINT('Ctrl Pts',(4.62166440161052,1.81739653227288,-10.9256614244434));
#57503=CARTESIAN_POINT('Ctrl Pts',(4.58197636066079,-0.0502825734189696,
-11.0756706063289));
#57504=CARTESIAN_POINT('Ctrl Pts',(4.54228831971106,-1.84008508857919,-10.7698741911437));
#57505=CARTESIAN_POINT('Ctrl Pts',(4.50260027876133,-3.62988760373941,-10.4640777759584));
#57506=CARTESIAN_POINT('Ctrl Pts',(4.4629122378116,-5.341813528368,-9.70247576370242));
#57507=CARTESIAN_POINT('Ctrl Pts',(4.42322419686186,-6.76733061329941,-8.57784003095039));
#57508=CARTESIAN_POINT('Ctrl Pts',(4.38353615591213,-8.1928476982308,-7.45320429819836));
#57509=CARTESIAN_POINT('Ctrl Pts',(4.34384811496241,-9.331955943465,-5.96553484495033));
#57510=CARTESIAN_POINT('Ctrl Pts',(4.30416007401268,-10.0458988753694,-4.29604690525213));
#57511=CARTESIAN_POINT('Ctrl Pts',(4.27200232446352,-10.6243803888725,-2.94332266501669));
#57512=CARTESIAN_POINT('Ctrl Pts',(4.23984457491436,-10.9237297922987,-1.47122984935265));
#57513=CARTESIAN_POINT('Ctrl Pts',(4.20768682536519,-10.9252346746171,0.00026931280733642));
#57514=CARTESIAN_POINT('Ctrl Pts',(3.99231317463481,-10.9240736852168,-6.866552131629E-6));
#57515=CARTESIAN_POINT('Ctrl Pts',(4.01195163646498,-10.9240934403711,-0.898913191757796));
#57516=CARTESIAN_POINT('Ctrl Pts',(4.03159009829515,-10.8143897236203,-1.79781477929459));
#57517=CARTESIAN_POINT('Ctrl Pts',(4.05122856012532,-10.5949061132788,-2.66906069943221));
#57518=CARTESIAN_POINT('Ctrl Pts',(4.0908302387854,-10.1523093619109,-4.42596005649798));
#57519=CARTESIAN_POINT('Ctrl Pts',(4.13043191744547,-9.26330143477245,-6.07039984927951));
#57520=CARTESIAN_POINT('Ctrl Pts',(4.17003359610555,-8.03571269221934,-7.4029211865655));
#57521=CARTESIAN_POINT('Ctrl Pts',(4.20963527476563,-6.80812394966622,-8.7354425238515));
#57522=CARTESIAN_POINT('Ctrl Pts',(4.2492369534257,-5.24195439169839,-9.75604540564196));
#57523=CARTESIAN_POINT('Ctrl Pts',(4.28883863208578,-3.52716928482937,-10.3409379363091));
#57524=CARTESIAN_POINT('Ctrl Pts',(4.32844031074586,-1.81238417796036,-10.9258304669763));
#57525=CARTESIAN_POINT('Ctrl Pts',(4.36804198940593,0.051016477809854,-11.0750126465202));
#57526=CARTESIAN_POINT('Ctrl Pts',(4.40764366806601,1.83701539055037,-10.7703897339555));
#57527=CARTESIAN_POINT('Ctrl Pts',(4.44724534672608,3.62301430329089,-10.4657668213908));
#57528=CARTESIAN_POINT('Ctrl Pts',(4.48684702538616,5.33161147300171,-9.70733881671743));
#57529=CARTESIAN_POINT('Ctrl Pts',(4.52644870404623,6.75556617337842,-8.58709766123175));
#57530=CARTESIAN_POINT('Ctrl Pts',(4.56605038270631,8.17952087375512,-7.46685650574606));
#57531=CARTESIAN_POINT('Ctrl Pts',(4.60565206136639,9.3188331047977,-5.98480219944806));
#57532=CARTESIAN_POINT('Ctrl Pts',(4.64525374002647,10.0353123682221,-4.32069742502651));
#57533=CARTESIAN_POINT('Ctrl Pts',(4.68485541868654,10.7517916316465,-2.65659265060497));
#57534=CARTESIAN_POINT('Ctrl Pts',(4.72445709734661,11.0454379274526,-0.810437408059887));
#57535=CARTESIAN_POINT('Ctrl Pts',(4.76405877600669,10.8806340412976,0.993842757068948));
#57536=CARTESIAN_POINT('Ctrl Pts',(4.80366045466677,10.7158301551426,2.79812292219779));
#57537=CARTESIAN_POINT('Ctrl Pts',(4.84326213332684,10.0925760870263,4.56052800991037));
#57538=CARTESIAN_POINT('Ctrl Pts',(4.88286381198692,9.08646813784316,6.06729077483388));
#57539=CARTESIAN_POINT('Ctrl Pts',(4.922465490647,8.08036018866002,7.57405353975738));
#57540=CARTESIAN_POINT('Ctrl Pts',(4.96206716930707,6.69139835840997,8.82517398189183));
#57541=CARTESIAN_POINT('Ctrl Pts',(5.00166884796715,5.08805387226729,9.66890005943429));
#57542=CARTESIAN_POINT('Ctrl Pts',(5.04127052662722,3.48470938612462,10.5126261369767));
#57543=CARTESIAN_POINT('Ctrl Pts',(5.0808722052873,1.6669822440893,10.9489578499272));
#57544=CARTESIAN_POINT('Ctrl Pts',(5.12047388394737,-0.144650135394457,
10.9249712541843));
#57545=CARTESIAN_POINT('Ctrl Pts',(5.16007556260745,-1.95628251487822,10.9009846584414));
#57546=CARTESIAN_POINT('Ctrl Pts',(5.19967724126753,-3.76182013181041,10.416679754005));
#57547=CARTESIAN_POINT('Ctrl Pts',(5.2392789199276,-5.34226407074355,9.53079929307428));
#57548=CARTESIAN_POINT('Ctrl Pts',(5.27888059858768,-6.92270800967669,8.64491883214355));
#57549=CARTESIAN_POINT('Ctrl Pts',(5.31848227724775,-8.27805827061078,7.35746281471844));
#57550=CARTESIAN_POINT('Ctrl Pts',(5.35808395590783,-9.24392047349389,5.82459053034145));
#57551=CARTESIAN_POINT('Ctrl Pts',(5.3976856345679,-10.209782676377,4.29171824596447));
#57552=CARTESIAN_POINT('Ctrl Pts',(5.43728731322798,-10.7861568212091,2.51342969463562));
#57553=CARTESIAN_POINT('Ctrl Pts',(5.47688899188806,-10.9031328095096,0.705418673283594));
#57554=CARTESIAN_POINT('Ctrl Pts',(5.48203038613697,-10.918319531231,0.470688788549498));
#57555=CARTESIAN_POINT('Ctrl Pts',(5.48717178038589,-10.9257629924177,0.235457924815266));
#57556=CARTESIAN_POINT('Ctrl Pts',(5.49231317463481,-10.9255540795388,0.000213857475631818));
#57557=CARTESIAN_POINT('Origin',(21.9,0.,0.));
#57558=CARTESIAN_POINT('',(7.2076868253652,-10.9242555967211,0.000178566634250859));
#57559=CARTESIAN_POINT('',(6.99231317463481,-10.9249214717915,-0.00028045959408001));
#57560=CARTESIAN_POINT('',(21.9,-10.925,-1.33792662806848E-15));
#57561=CARTESIAN_POINT('Ctrl Pts',(7.2076868253652,-10.9242555967211,0.000178566634250859));
#57562=CARTESIAN_POINT('Ctrl Pts',(7.19235755770789,-10.9246636458058,0.701807649372725));
#57563=CARTESIAN_POINT('Ctrl Pts',(7.17702829005058,-10.8581089457588,1.40336030847505));
#57564=CARTESIAN_POINT('Ctrl Pts',(7.16169902239328,-10.7238457643368,2.09170630084375));
#57565=CARTESIAN_POINT('Ctrl Pts',(7.12201098144355,-10.3762334216314,3.87385953499978));
#57566=CARTESIAN_POINT('Ctrl Pts',(7.08232294049381,-9.57476350967704,5.56748699601942));
#57567=CARTESIAN_POINT('Ctrl Pts',(7.04263489954408,-8.41706427334937,6.96628539787022));
#57568=CARTESIAN_POINT('Ctrl Pts',(7.00294685859435,-7.25936503702171,8.36508379972102));
#57569=CARTESIAN_POINT('Ctrl Pts',(6.96325881764462,-5.74543647632069,9.469053142403));
#57570=CARTESIAN_POINT('Ctrl Pts',(6.92357077669489,-4.05969248632037,10.1437172743915));
#57571=CARTESIAN_POINT('Ctrl Pts',(6.88388273574516,-2.37394849632007,10.81838140638));
#57572=CARTESIAN_POINT('Ctrl Pts',(6.84419469479543,-0.516389077020457,
11.063740327675));
#57573=CARTESIAN_POINT('Ctrl Pts',(6.8045066538457,1.28671368930408,10.8499065022714));
#57574=CARTESIAN_POINT('Ctrl Pts',(6.76481861289597,3.08981645562862,10.6360726768678));
#57575=CARTESIAN_POINT('Ctrl Pts',(6.72513057194625,4.83846256897808,9.96304610476567));
#57576=CARTESIAN_POINT('Ctrl Pts',(6.68544253099652,6.31964683925319,8.9128091561186));
#57577=CARTESIAN_POINT('Ctrl Pts',(6.64575449004679,7.8008311095283,7.86257220747154));
#57578=CARTESIAN_POINT('Ctrl Pts',(6.60606644909705,9.01455353672906,6.43512488227957));
#57579=CARTESIAN_POINT('Ctrl Pts',(6.56637840814732,9.81296878247627,4.80434666738573));
#57580=CARTESIAN_POINT('Ctrl Pts',(6.52669036719759,10.6113840282235,3.17356845249184));
#57581=CARTESIAN_POINT('Ctrl Pts',(6.48700232624786,10.9944920925172,1.33945934789606));
#57582=CARTESIAN_POINT('Ctrl Pts',(6.44731428529813,10.9156260108751,-0.474565081923047));
#57583=CARTESIAN_POINT('Ctrl Pts',(6.4076262443484,10.8367599292331,-2.28858951174213));
#57584=CARTESIAN_POINT('Ctrl Pts',(6.36793820339867,10.2959197016554,-4.08252926678453));
#57585=CARTESIAN_POINT('Ctrl Pts',(6.32825016244894,9.35898588259446,-5.6378618709287));
#57586=CARTESIAN_POINT('Ctrl Pts',(6.28856212149921,8.42205206353352,-7.19319447507288));
#57587=CARTESIAN_POINT('Ctrl Pts',(6.24887408054947,7.08902465298934,-8.50991992831882));
#57588=CARTESIAN_POINT('Ctrl Pts',(6.20918603959974,5.52228170723231,-9.42764594011897));
#57589=CARTESIAN_POINT('Ctrl Pts',(6.16949799865001,3.95553876147531,-10.3453719519191));
#57590=CARTESIAN_POINT('Ctrl Pts',(6.12980995770028,2.15508028050548,-10.8640985222735));
#57591=CARTESIAN_POINT('Ctrl Pts',(6.09012191675055,0.340222796168268,-10.920638794285));
#57592=CARTESIAN_POINT('Ctrl Pts',(6.05043387580082,-1.47463468816894,-10.9771790662965));
#57593=CARTESIAN_POINT('Ctrl Pts',(6.01074583485109,-3.30389117587354,-10.5715330399651));
#57594=CARTESIAN_POINT('Ctrl Pts',(5.97105779390136,-4.92472220696516,-9.75311306253027));
#57595=CARTESIAN_POINT('Ctrl Pts',(5.93136975295163,-6.5455532380568,-8.93469308509545));
#57596=CARTESIAN_POINT('Ctrl Pts',(5.8916817120019,-7.95795881253547,-7.70349915655719));
#57597=CARTESIAN_POINT('Ctrl Pts',(5.85199367105217,-8.98989170163808,-6.20950484492065));
#57598=CARTESIAN_POINT('Ctrl Pts',(5.81230563010244,-10.0218245907407,-4.7155105332841));
#57599=CARTESIAN_POINT('Ctrl Pts',(5.77261758915271,-10.6732847944673,-2.95871583854928));
#57600=CARTESIAN_POINT('Ctrl Pts',(5.73292954820297,-10.8649169741489,-1.1531185416626));
#57601=CARTESIAN_POINT('Ctrl Pts',(5.72451530725705,-10.9055448130204,-0.770314796661375));
#57602=CARTESIAN_POINT('Ctrl Pts',(5.71610106631112,-10.9255042927422,-0.385317471330169));
#57603=CARTESIAN_POINT('Ctrl Pts',(5.70768682536519,-10.9251067326884,-0.000279136740874882));
#57604=CARTESIAN_POINT('Ctrl Pts',(5.49231317463481,-10.9255540795388,0.000213857475631818));
#57605=CARTESIAN_POINT('Ctrl Pts',(5.52677345904597,-10.9241538373331,-1.57651359700247));
#57606=CARTESIAN_POINT('Ctrl Pts',(5.56123374345713,-10.5789803361197,-3.15383420680999));
#57607=CARTESIAN_POINT('Ctrl Pts',(5.59569402786829,-9.91739968676565,-4.58487775402611));
#57608=CARTESIAN_POINT('Ctrl Pts',(5.63529570652836,-9.15711274395221,-6.22942966860854));
#57609=CARTESIAN_POINT('Ctrl Pts',(5.67489738518843,-7.9789610265564,-7.68080000639817));
#57610=CARTESIAN_POINT('Ctrl Pts',(5.71449906384851,-6.52584598726614,-8.76294783260207));
#57611=CARTESIAN_POINT('Ctrl Pts',(5.75410074250859,-5.07273094797588,-9.84509565880597));
#57612=CARTESIAN_POINT('Ctrl Pts',(5.79370242116867,-3.34465258679113,-10.5580209734241));
#57613=CARTESIAN_POINT('Ctrl Pts',(5.83330409982874,-1.55121456046141,-10.8152509889431));
#57614=CARTESIAN_POINT('Ctrl Pts',(5.87290577848882,0.242223465868305,-11.0724810044621));
#57615=CARTESIAN_POINT('Ctrl Pts',(5.91250745714889,2.10102115734298,-10.874015720882));
#57616=CARTESIAN_POINT('Ctrl Pts',(5.95210913580897,3.79971952897577,-10.2439275703972));
#57617=CARTESIAN_POINT('Ctrl Pts',(5.99171081446904,5.49841790060856,-9.61383941991229));
#57618=CARTESIAN_POINT('Ctrl Pts',(6.03131249312912,7.03701695239944,-8.55212840252267));
#57619=CARTESIAN_POINT('Ctrl Pts',(6.0709141717892,8.22889552481629,-7.18757253932655));
#57620=CARTESIAN_POINT('Ctrl Pts',(6.11051585044927,9.42077409723316,-5.82301667613042));
#57621=CARTESIAN_POINT('Ctrl Pts',(6.15011752910935,10.265932190276,-4.15561596712778));
#57622=CARTESIAN_POINT('Ctrl Pts',(6.18971920776942,10.6618581176624,-2.38761429993609));
#57623=CARTESIAN_POINT('Ctrl Pts',(6.2293208864295,11.0577840450488,-0.61961263274444));
#57624=CARTESIAN_POINT('Ctrl Pts',(6.26892256508958,11.0044778067788,1.24898999263627));
#57625=CARTESIAN_POINT('Ctrl Pts',(6.30852424374965,10.5084050717247,2.99154532223279));
#57626=CARTESIAN_POINT('Ctrl Pts',(6.34812592240973,10.0123323366707,4.73410065182934));
#57627=CARTESIAN_POINT('Ctrl Pts',(6.3877276010698,9.07349310483258,6.3506086856417));
#57628=CARTESIAN_POINT('Ctrl Pts',(6.42732927972988,7.80576192062532,7.64499845683035));
#57629=CARTESIAN_POINT('Ctrl Pts',(6.46693095838995,6.53803073641807,8.93938822801901));
#57630=CARTESIAN_POINT('Ctrl Pts',(6.50653263705003,4.94140759984165,9.91165973658394));
#57631=CARTESIAN_POINT('Ctrl Pts',(6.54613431571011,3.20955158064322,10.4438833399083));
#57632=CARTESIAN_POINT('Ctrl Pts',(6.58573599437018,1.47769556144478,10.9761069432326));
#57633=CARTESIAN_POINT('Ctrl Pts',(6.62533767303026,-0.389393340375631,
11.0682826413163));
#57634=CARTESIAN_POINT('Ctrl Pts',(6.66493935169033,-2.16525047478358,10.7092301753148));
#57635=CARTESIAN_POINT('Ctrl Pts',(6.70454103035041,-3.94110760919151,10.3501777093133));
#57636=CARTESIAN_POINT('Ctrl Pts',(6.74414270901049,-5.62573297618696,9.53989707922652));
#57637=CARTESIAN_POINT('Ctrl Pts',(6.78374438767056,-7.01479345922472,8.3766695822887));
#57638=CARTESIAN_POINT('Ctrl Pts',(6.82334606633064,-8.40385394226249,7.21344208535088));
#57639=CARTESIAN_POINT('Ctrl Pts',(6.86294774499071,-9.49734954134259,5.69726772156196));
#57640=CARTESIAN_POINT('Ctrl Pts',(6.90254942365079,-10.1626469908939,4.01204769474357));
#57641=CARTESIAN_POINT('Ctrl Pts',(6.93247067397879,-10.6653158727229,2.73877110682369));
#57642=CARTESIAN_POINT('Ctrl Pts',(6.9623919243068,-10.9235420555249,1.36899251819409));
#57643=CARTESIAN_POINT('Ctrl Pts',(6.99231317463481,-10.9249214717915,-0.00028045959408001));
#57644=CARTESIAN_POINT('Origin',(21.9,0.,0.));
#57645=CARTESIAN_POINT('',(8.70768682536519,-10.9259303319926,-2.98385707583761E-5));
#57646=CARTESIAN_POINT('',(8.4923131746348,-10.9242785920375,0.000183038237066875));
#57647=CARTESIAN_POINT('',(21.9,-10.925,-1.33792662806848E-15));
#57648=CARTESIAN_POINT('Ctrl Pts',(8.70768682536519,-10.9259303319926,-2.98385707583761E-5));
#57649=CARTESIAN_POINT('Ctrl Pts',(8.66861404910465,-10.9256497463441,1.7875629141296));
#57650=CARTESIAN_POINT('Ctrl Pts',(8.62954127284411,-10.4780185717367,3.57529106564087));
#57651=CARTESIAN_POINT('Ctrl Pts',(8.59046849658358,-9.63515114517691,5.15169541373229));
#57652=CARTESIAN_POINT('Ctrl Pts',(8.55078045563384,-8.77901139412766,6.75292282340506));
#57653=CARTESIAN_POINT('Ctrl Pts',(8.51109241468412,-7.51509010889808,8.13611875357229));
#57654=CARTESIAN_POINT('Ctrl Pts',(8.47140437373439,-5.99734742560453,9.13279404579283));
#57655=CARTESIAN_POINT('Ctrl Pts',(8.43171633278466,-4.47960474231098,10.1294693380134));
#57656=CARTESIAN_POINT('Ctrl Pts',(8.39202829183492,-2.70804066095336,10.7396239922872));
#57657=CARTESIAN_POINT('Ctrl Pts',(8.35234025088519,-0.898452043482406,
10.8889341605061));
#57658=CARTESIAN_POINT('Ctrl Pts',(8.31265220993546,0.911136573988525,11.0382443287249));
#57659=CARTESIAN_POINT('Ctrl Pts',(8.27296416898573,2.75874972757288,10.7267100108889));
#57660=CARTESIAN_POINT('Ctrl Pts',(8.233276128036,4.41932690445194,9.99227966671578));
#57661=CARTESIAN_POINT('Ctrl Pts',(8.19358808708627,6.07990408133099,9.25784932254263));
#57662=CARTESIAN_POINT('Ctrl Pts',(8.15390004613654,7.55344528150469,8.10052295203235));
#57663=CARTESIAN_POINT('Ctrl Pts',(8.11421200518681,8.66045625449776,6.66127620581861));
#57664=CARTESIAN_POINT('Ctrl Pts',(8.07452396423708,9.76746722749084,5.22202945960484));
#57665=CARTESIAN_POINT('Ctrl Pts',(8.03483592328735,10.5079479733033,3.50086233768759));
#57666=CARTESIAN_POINT('Ctrl Pts',(7.99514788233762,10.7916994283153,1.70743277325173));
#57667=CARTESIAN_POINT('Ctrl Pts',(7.95545984138789,11.0754508833272,-0.0859967911841325));
#57668=CARTESIAN_POINT('Ctrl Pts',(7.91577180043816,10.9024730475387,-1.9516887981386));
#57669=CARTESIAN_POINT('Ctrl Pts',(7.87608375948843,10.2938366090174,-3.66238052271029));
#57670=CARTESIAN_POINT('Ctrl Pts',(7.8363957185387,9.68520017049604,-5.37307224728197));
#57671=CARTESIAN_POINT('Ctrl Pts',(7.79670767758897,8.64090512924188,-6.92876368947084));
#57672=CARTESIAN_POINT('Ctrl Pts',(7.75701963663924,7.28815862115501,-8.13995375534519));
#57673=CARTESIAN_POINT('Ctrl Pts',(7.71733159568951,5.9354121130681,-9.35114382121957));
#57674=CARTESIAN_POINT('Ctrl Pts',(7.67764355473977,4.27421413814847,-10.2178325107794));
#57675=CARTESIAN_POINT('Ctrl Pts',(7.63795551379004,2.50691769837805,-10.6344471826152));
#57676=CARTESIAN_POINT('Ctrl Pts',(7.59826747284031,0.739621258607676,-11.0510618544511));
#57677=CARTESIAN_POINT('Ctrl Pts',(7.55857943189058,-1.13377364601349,-11.017602508563));
#57678=CARTESIAN_POINT('Ctrl Pts',(7.51889139094085,-2.88506598913512,-10.5381448777577));
#57679=CARTESIAN_POINT('Ctrl Pts',(7.47920334999113,-4.63635833225675,-10.0586872469523));
#57680=CARTESIAN_POINT('Ctrl Pts',(7.4395153090414,-6.26554811387886,-9.13323133122978));
#57681=CARTESIAN_POINT('Ctrl Pts',(7.39982726809166,-7.57418129776567,-7.87450829543351));
#57682=CARTESIAN_POINT('Ctrl Pts',(7.36013922714193,-8.8828144816525,-6.61578525963721));
#57683=CARTESIAN_POINT('Ctrl Pts',(7.3204511861922,-9.87089106780401,-5.02379510376719));
#57684=CARTESIAN_POINT('Ctrl Pts',(7.28076314524247,-10.4180519741515,-3.29246052218596));
#57685=CARTESIAN_POINT('Ctrl Pts',(7.25640437195004,-10.7538752638189,-2.22984353336837));
#57686=CARTESIAN_POINT('Ctrl Pts',(7.23204559865762,-10.923607191633,-1.1147359970535));
#57687=CARTESIAN_POINT('Ctrl Pts',(7.2076868253652,-10.9242555967211,0.000178566634250859));
#57688=CARTESIAN_POINT('Ctrl Pts',(6.99231317463481,-10.9249214717915,-0.00028045959408001));
#57689=CARTESIAN_POINT('Ctrl Pts',(7.00199360296688,-10.9253677546226,-0.443281630441308));
#57690=CARTESIAN_POINT('Ctrl Pts',(7.01167403129895,-10.8989294252916,-0.88622987809406));
#57691=CARTESIAN_POINT('Ctrl Pts',(7.02135445963102,-10.8451864264073,-1.32584008948809));
#57692=CARTESIAN_POINT('Ctrl Pts',(7.0609561382911,-10.6253291123467,-3.12424215705347));
#57693=CARTESIAN_POINT('Ctrl Pts',(7.10055781695117,-9.94851518420288,-4.86678060233632));
#57694=CARTESIAN_POINT('Ctrl Pts',(7.14015949561124,-8.89683737426413,-6.34209786287786));
#57695=CARTESIAN_POINT('Ctrl Pts',(7.17976117427132,-7.84515956432538,-7.81741512341939));
#57696=CARTESIAN_POINT('Ctrl Pts',(7.2193628529314,-6.4186178725917,-9.02551119921961));
#57697=CARTESIAN_POINT('Ctrl Pts',(7.25896453159147,-4.79024169507264,-9.81985259915903));
#57698=CARTESIAN_POINT('Ctrl Pts',(7.29856621025155,-3.16186551755356,-10.6141939990985));
#57699=CARTESIAN_POINT('Ctrl Pts',(7.33816788891163,-1.33165485424912,-10.9947807231771));
#57700=CARTESIAN_POINT('Ctrl Pts',(7.3777695675717,0.478398713748622,-10.9154502993283));
#57701=CARTESIAN_POINT('Ctrl Pts',(7.41737124623178,2.28845228174635,-10.8361198754795));
#57702=CARTESIAN_POINT('Ctrl Pts',(7.45697292489185,4.07834875443735,-10.2968723037033));
#57703=CARTESIAN_POINT('Ctrl Pts',(7.49657460355193,5.6309863763076,-9.3631144923183));
#57704=CARTESIAN_POINT('Ctrl Pts',(7.536176282212,7.18362399817784,-8.42935668093334));
#57705=CARTESIAN_POINT('Ctrl Pts',(7.57577796087208,8.49900276922735,-7.10108862993964));
#57706=CARTESIAN_POINT('Ctrl Pts',(7.61537963953216,9.41757656781287,-5.53941983927964));
#57707=CARTESIAN_POINT('Ctrl Pts',(7.65498131819223,10.3361503663984,-3.97775104861962));
#57708=CARTESIAN_POINT('Ctrl Pts',(7.69458299685231,10.8579191925199,-2.1826815182933));
#57709=CARTESIAN_POINT('Ctrl Pts',(7.73418467551238,10.919596185819,-0.371940459039667));
#57710=CARTESIAN_POINT('Ctrl Pts',(7.77378635417246,10.981273179118,1.43880060021396));
#57711=CARTESIAN_POINT('Ctrl Pts',(7.81338803283254,10.5828583395945,3.26521318839486));
#57712=CARTESIAN_POINT('Ctrl Pts',(7.85298971149261,9.77267656335449,4.88576640400303));
#57713=CARTESIAN_POINT('Ctrl Pts',(7.89259139015269,8.9624947871145,6.50631961961119));
#57714=CARTESIAN_POINT('Ctrl Pts',(7.93219306881276,7.74054607415802,7.92101346264662));
#57715=CARTESIAN_POINT('Ctrl Pts',(7.97179474747283,6.25504414230537,8.95825559717036));
#57716=CARTESIAN_POINT('Ctrl Pts',(8.01139642613291,4.76954221045273,9.9954977316941));
#57717=CARTESIAN_POINT('Ctrl Pts',(8.05099810479299,3.02048705970387,10.6552881577062));
#57718=CARTESIAN_POINT('Ctrl Pts',(8.09059978345307,1.22002668270086,10.8575989730658));
#57719=CARTESIAN_POINT('Ctrl Pts',(8.13020146211315,-0.58043369430216,11.0599097884255));
#57720=CARTESIAN_POINT('Ctrl Pts',(8.16980314077322,-2.43229929755934,10.8047409931328));
#57721=CARTESIAN_POINT('Ctrl Pts',(8.20940481943329,-4.11095195525057,10.1230427534435));
#57722=CARTESIAN_POINT('Ctrl Pts',(8.24900649809337,-5.78960461294178,9.44134451375414));
#57723=CARTESIAN_POINT('Ctrl Pts',(8.28860817675345,-7.29504432506704,8.33311682966819));
#57724=CARTESIAN_POINT('Ctrl Pts',(8.32820985541352,-8.44467192496528,6.93277986424824));
#57725=CARTESIAN_POINT('Ctrl Pts',(8.3678115340736,-9.59429952486353,5.53244289882829));
#57726=CARTESIAN_POINT('Ctrl Pts',(8.40741321273367,-10.3881150125348,3.83999665207435));
#57727=CARTESIAN_POINT('Ctrl Pts',(8.44701489139375,-10.7298341958164,2.06072285781258));
#57728=CARTESIAN_POINT('Ctrl Pts',(8.46211431914076,-10.8601257463848,1.38231686575294));
#57729=CARTESIAN_POINT('Ctrl Pts',(8.47721374688778,-10.9246931825979,0.691288201032229));
#57730=CARTESIAN_POINT('Ctrl Pts',(8.4923131746348,-10.9242785920375,0.000183038237066875));
#57731=CARTESIAN_POINT('Origin',(21.9,0.,0.));
#57732=CARTESIAN_POINT('',(10.2076868253652,-10.924167183502,-0.000134674578820061));
#57733=CARTESIAN_POINT('',(9.99231317463481,-10.9259274088367,1.33692176457333E-5));
#57734=CARTESIAN_POINT('',(21.9,-10.925,-1.33792662806848E-15));
#57735=CARTESIAN_POINT('Ctrl Pts',(10.2076868253652,-10.924167183502,-0.000134674578820061));
#57736=CARTESIAN_POINT('Ctrl Pts',(10.1845585814512,-10.9237076188205,1.05848240286772));
#57737=CARTESIAN_POINT('Ctrl Pts',(10.1614303375371,-10.7709362504589,2.11722930447063));
#57738=CARTESIAN_POINT('Ctrl Pts',(10.1383020936231,-10.4677166887345,3.13097597414337));
#57739=CARTESIAN_POINT('Ctrl Pts',(10.0986140526733,-9.94739225652934,4.87056413691764));
#57740=CARTESIAN_POINT('Ctrl Pts',(10.0589260117236,-8.98405022072023,6.47764226772867));
#57741=CARTESIAN_POINT('Ctrl Pts',(10.0192379707739,-7.69503671092234,7.75644978349191));
#57742=CARTESIAN_POINT('Ctrl Pts',(9.97954992982415,-6.40602320112446,9.03525729925515));
#57743=CARTESIAN_POINT('Ctrl Pts',(9.93986188887442,-4.7913382173378,9.98579419997061));
#57744=CARTESIAN_POINT('Ctrl Pts',(9.90017384792469,-3.04766894474881,10.4922741686199));
#57745=CARTESIAN_POINT('Ctrl Pts',(9.86048580697496,-1.30399967215984,10.9987541372692));
#57746=CARTESIAN_POINT('Ctrl Pts',(9.82079776602523,0.568653889231388,11.0611771738523));
#57747=CARTESIAN_POINT('Ctrl Pts',(9.7811097250755,2.3421810171988,10.6719394352174));
#57748=CARTESIAN_POINT('Ctrl Pts',(9.74142168412577,4.11570814516621,10.2827016965825));
#57749=CARTESIAN_POINT('Ctrl Pts',(9.70173364317603,5.79010883970979,9.44180318272959));
#57750=CARTESIAN_POINT('Ctrl Pts',(9.66204560222631,7.16142185588636,8.25167499531504));
#57751=CARTESIAN_POINT('Ctrl Pts',(9.62235756127658,8.53273487206292,7.06154680790049));
#57752=CARTESIAN_POINT('Ctrl Pts',(9.58266952032685,9.60096020987254,5.52218894692426));
#57753=CARTESIAN_POINT('Ctrl Pts',(9.54298147937712,10.2359757483143,3.8211128884391));
#57754=CARTESIAN_POINT('Ctrl Pts',(9.50329343842738,10.8709912867561,2.12003682995393));
#57755=CARTESIAN_POINT('Ctrl Pts',(9.46360539747765,11.0727970258301,0.257242573959836));
#57756=CARTESIAN_POINT('Ctrl Pts',(9.42391735652792,10.8168107075902,-1.5403601340065));
#57757=CARTESIAN_POINT('Ctrl Pts',(9.38422931557819,10.5608243893503,-3.3379628419729));
#57758=CARTESIAN_POINT('Ctrl Pts',(9.34454127462846,9.84704601379663,-5.07037400191152));
#57759=CARTESIAN_POINT('Ctrl Pts',(9.30485323367873,8.76242198901756,-6.52656602760255));
#57760=CARTESIAN_POINT('Ctrl Pts',(9.265165192729,7.67779796423852,-7.98275805329355));
#57761=CARTESIAN_POINT('Ctrl Pts',(9.22547715177927,6.22232829023412,-9.16273094473696));
#57762=CARTESIAN_POINT('Ctrl Pts',(9.18578911082954,4.57330589793434,-9.92275044482089));
#57763=CARTESIAN_POINT('Ctrl Pts',(9.14610106987981,2.92428350563452,-10.6827699449049));
#57764=CARTESIAN_POINT('Ctrl Pts',(9.10641302893008,1.08170839503929,-11.0228360536293));
#57765=CARTESIAN_POINT('Ctrl Pts',(9.06672498798035,-0.729972612560106,
-10.9015248112907));
#57766=CARTESIAN_POINT('Ctrl Pts',(9.02703694703061,-2.54165362015945,-10.7802135689521));
#57767=CARTESIAN_POINT('Ctrl Pts',(8.98734890608088,-4.32244052476298,-10.1975249755504));
#57768=CARTESIAN_POINT('Ctrl Pts',(8.94766086513115,-5.85541301857049,-9.22443719737033));
#57769=CARTESIAN_POINT('Ctrl Pts',(8.90797282418142,-7.38838551237801,-8.25134941919023));
#57770=CARTESIAN_POINT('Ctrl Pts',(8.8682847832317,-8.67354359538951,-6.88786245623167));
#57771=CARTESIAN_POINT('Ctrl Pts',(8.82859674228197,-9.55434024548907,-5.30006468825638));
#57772=CARTESIAN_POINT('Ctrl Pts',(8.78890870133224,-10.4351368955886,-3.71226692028107));
#57773=CARTESIAN_POINT('Ctrl Pts',(8.7492206603825,-10.9115721127762,-1.90015834728901));
#57774=CARTESIAN_POINT('Ctrl Pts',(8.70953261943277,-10.9256106129356,-0.0844746162038638));
#57775=CARTESIAN_POINT('Ctrl Pts',(8.70891735474358,-10.9258282450795,-0.0563269409912714));
#57776=CARTESIAN_POINT('Ctrl Pts',(8.70830209005439,-10.925934750272,-0.0281784065675201));
#57777=CARTESIAN_POINT('Ctrl Pts',(8.70768682536519,-10.9259303319926,-2.98385707583761E-5));
#57778=CARTESIAN_POINT('Ctrl Pts',(8.4923131746348,-10.9242785920375,0.000183038237066875));
#57779=CARTESIAN_POINT('Ctrl Pts',(8.51681542554786,-10.9236058246911,-1.12129205272877));
#57780=CARTESIAN_POINT('Ctrl Pts',(8.54131767646092,-10.7518195701733,-2.24296858173727));
#57781=CARTESIAN_POINT('Ctrl Pts',(8.56581992737398,-10.4120907949402,-3.31123630149607));
#57782=CARTESIAN_POINT('Ctrl Pts',(8.60542160603405,-9.86300533189009,-5.03782032477338));
#57783=CARTESIAN_POINT('Ctrl Pts',(8.64502328469413,-8.87521152689784,-6.62488702955846));
#57784=CARTESIAN_POINT('Ctrl Pts',(8.68462496335421,-7.56852176711635,-7.87993647354526));
#57785=CARTESIAN_POINT('Ctrl Pts',(8.72422664201428,-6.26183200733487,-9.13498591753203));
#57786=CARTESIAN_POINT('Ctrl Pts',(8.76382832067435,-4.63624629276417,-10.0580181007206));
#57787=CARTESIAN_POINT('Ctrl Pts',(8.80342999933443,-2.88893664857795,-10.5370757616583));
#57788=CARTESIAN_POINT('Ctrl Pts',(8.84303167799451,-1.1416270043917,-11.016133422596));
#57789=CARTESIAN_POINT('Ctrl Pts',(8.88263335665459,0.727406569410031,-11.0512165612828));
#57790=CARTESIAN_POINT('Ctrl Pts',(8.92223503531466,2.49146354786511,-10.6380698416622));
#57791=CARTESIAN_POINT('Ctrl Pts',(8.96183671397473,4.2555205263202,-10.2249231220415));
#57792=CARTESIAN_POINT('Ctrl Pts',(9.00143839263481,5.91460090942858,-9.36354654411344));
#57793=CARTESIAN_POINT('Ctrl Pts',(9.04104007129488,7.26747000613012,-8.1584189814217));
#57794=CARTESIAN_POINT('Ctrl Pts',(9.08064174995496,8.62033910283164,-6.95329141872997));
#57795=CARTESIAN_POINT('Ctrl Pts',(9.12024342861504,9.66699691312632,-5.40441287127457));
#57796=CARTESIAN_POINT('Ctrl Pts',(9.15984510727512,10.2804912632407,-3.69965132855166));
#57797=CARTESIAN_POINT('Ctrl Pts',(9.19944678593519,10.8939856133551,-1.99488978582873));
#57798=CARTESIAN_POINT('Ctrl Pts',(9.23904846459526,11.0743165032893,-0.134245247838266));
#57799=CARTESIAN_POINT('Ctrl Pts',(9.27865014325534,10.7996110742631,1.65659929104078));
#57800=CARTESIAN_POINT('Ctrl Pts',(9.31825182191542,10.5249056452369,3.44744382991983));
#57801=CARTESIAN_POINT('Ctrl Pts',(9.3578535005755,9.79516389725042,5.16848836968742));
#57802=CARTESIAN_POINT('Ctrl Pts',(9.39745517923557,8.69889833199122,6.61098240627693));
#57803=CARTESIAN_POINT('Ctrl Pts',(9.43705685789565,7.60263276673204,8.05347644286642));
#57804=CARTESIAN_POINT('Ctrl Pts',(9.47665853655572,6.13984338420013,9.21741997627785));
#57805=CARTESIAN_POINT('Ctrl Pts',(9.51626021521579,4.48795616837859,9.96163490583425));
#57806=CARTESIAN_POINT('Ctrl Pts',(9.55586189387587,2.83606895255704,10.7058498353907));
#57807=CARTESIAN_POINT('Ctrl Pts',(9.59546357253595,0.995083903445857,11.0303361610921));
#57808=CARTESIAN_POINT('Ctrl Pts',(9.63506525119603,-0.811700541232406,
10.8957359915605));
#57809=CARTESIAN_POINT('Ctrl Pts',(9.6746669298561,-2.61848498591067,10.7611358220289));
#57810=CARTESIAN_POINT('Ctrl Pts',(9.71426860851617,-4.39106882615596,10.1674491572642));
#57811=CARTESIAN_POINT('Ctrl Pts',(9.75387028717625,-5.91445020605962,9.18668598170548));
#57812=CARTESIAN_POINT('Ctrl Pts',(9.79347196583632,-7.43783158596328,8.20592280614672));
#57813=CARTESIAN_POINT('Ctrl Pts',(9.8330736444964,-8.71201050552532,6.83808311979378));
#57814=CARTESIAN_POINT('Ctrl Pts',(9.87267532315648,-9.58243809306706,5.24907618147805));
#57815=CARTESIAN_POINT('Ctrl Pts',(9.91227700181656,-10.4528656806088,3.66006924316229));
#57816=CARTESIAN_POINT('Ctrl Pts',(9.95187868047663,-10.9195419361303,1.84989505288373));
#57817=CARTESIAN_POINT('Ctrl Pts',(9.99148035913671,-10.9258623375956,0.0381149095731016));
#57818=CARTESIAN_POINT('Ctrl Pts',(9.99175796430274,-10.9259066431947,0.0254144497815587));
#57819=CARTESIAN_POINT('Ctrl Pts',(9.99203556946878,-10.9259283272851,0.0127139110748031));
#57820=CARTESIAN_POINT('Ctrl Pts',(9.99231317463481,-10.9259274088367,1.33692176457333E-5));
#57821=CARTESIAN_POINT('Origin',(21.9,0.,0.));
#57822=CARTESIAN_POINT('',(11.7076868253652,-10.9252842859753,0.000263961161978608));
#57823=CARTESIAN_POINT('',(11.4923131746348,-10.924327996449,-0.000200333677245087));
#57824=CARTESIAN_POINT('',(21.9,-10.925,-1.33792662806848E-15));
#57825=CARTESIAN_POINT('Ctrl Pts',(11.7076868253652,-10.9252842859753,0.000263961161978608));
#57826=CARTESIAN_POINT('Ctrl Pts',(11.7005031137977,-10.9256174345997,0.328977483484901));
#57827=CARTESIAN_POINT('Ctrl Pts',(11.6933194022301,-10.9110769211568,0.657661639621172));
#57828=CARTESIAN_POINT('Ctrl Pts',(11.6861356906626,-10.8814483208165,0.984980034150224));
#57829=CARTESIAN_POINT('Ctrl Pts',(11.6464476497128,-10.7177584103109,2.79332460972552));
#57830=CARTESIAN_POINT('Ctrl Pts',(11.6067596087631,-10.0935408315302,4.55998258761169));
#57831=CARTESIAN_POINT('Ctrl Pts',(11.5670715678134,-9.08483245838282,6.06975472563663));
#57832=CARTESIAN_POINT('Ctrl Pts',(11.5273835268636,-8.07612408523548,7.57952686366158));
#57833=CARTESIAN_POINT('Ctrl Pts',(11.4876954859139,-6.68292491772155,8.8324131618253));
#57834=CARTESIAN_POINT('Ctrl Pts',(11.4480074449642,-5.07494262353716,9.67579767223768));
#57835=CARTESIAN_POINT('Ctrl Pts',(11.4083194040144,-3.4669603293528,10.51918218265));
#57836=CARTESIAN_POINT('Ctrl Pts',(11.3686313630647,-1.64419490849798,10.9530649053111));
#57837=CARTESIAN_POINT('Ctrl Pts',(11.328943322115,0.171319865577336,10.9245939389038));
#57838=CARTESIAN_POINT('Ctrl Pts',(11.2892552811653,1.98683463965268,10.8961229724964));
#57839=CARTESIAN_POINT('Ctrl Pts',(11.2495672402155,3.79509876694853,10.4052983170207));
#57840=CARTESIAN_POINT('Ctrl Pts',(11.2098791992658,5.37584489820313,9.51190805552375));
#57841=CARTESIAN_POINT('Ctrl Pts',(11.1701911583161,6.95659102945774,8.61851779402679));
#57842=CARTESIAN_POINT('Ctrl Pts',(11.1305031173663,8.3098191646711,7.32256192650859));
#57843=CARTESIAN_POINT('Ctrl Pts',(11.0908150764166,9.27069056718387,5.78190276931412));
#57844=CARTESIAN_POINT('Ctrl Pts',(11.0511270354669,10.2315619696966,4.24124361211968));
#57845=CARTESIAN_POINT('Ctrl Pts',(11.0114389945171,10.8000766395088,2.45588116524898));
#57846=CARTESIAN_POINT('Ctrl Pts',(10.9717509535674,10.9069829570999,0.643293090127379));
#57847=CARTESIAN_POINT('Ctrl Pts',(10.9320629126177,11.0138892746911,-1.16929498499427));
#57848=CARTESIAN_POINT('Ctrl Pts',(10.892374871668,10.6591872400612,-3.00910868836681));
#57849=CARTESIAN_POINT('Ctrl Pts',(10.8526868307182,9.88608363686888,-4.65203756982978));
#57850=CARTESIAN_POINT('Ctrl Pts',(10.8129987897685,9.11298003367656,-6.29496645129269));
#57851=CARTESIAN_POINT('Ctrl Pts',(10.7733107488188,7.92147486192183,-7.74101051084603));
#57852=CARTESIAN_POINT('Ctrl Pts',(10.733622707869,6.45670714297461,-8.81402496570863));
#57853=CARTESIAN_POINT('Ctrl Pts',(10.6939346669193,4.99193942402739,-9.88703942057122));
#57854=CARTESIAN_POINT('Ctrl Pts',(10.6542466259696,3.25390915788768,-10.5870242707431));
#57855=CARTESIAN_POINT('Ctrl Pts',(10.6145585850198,1.45432840247911,-10.8287133180271));
#57856=CARTESIAN_POINT('Ctrl Pts',(10.5748705440701,-0.34525235292946,-11.0704023653111));
#57857=CARTESIAN_POINT('Ctrl Pts',(10.5351825031204,-2.20638359760688,-10.8537956097072));
#57858=CARTESIAN_POINT('Ctrl Pts',(10.4954944621706,-3.90235815990432,-10.2052782430516));
#57859=CARTESIAN_POINT('Ctrl Pts',(10.4558064212209,-5.59833272220181,-9.55676087639598));
#57860=CARTESIAN_POINT('Ctrl Pts',(10.4161183802712,-7.12915060211931,-8.47633289868858));
#57861=CARTESIAN_POINT('Ctrl Pts',(10.3764303393215,-8.30834059142896,-7.095602852689));
#57862=CARTESIAN_POINT('Ctrl Pts',(10.3367422983717,-9.48753058073859,-5.71487280668943));
#57863=CARTESIAN_POINT('Ctrl Pts',(10.297054257422,-10.3150926794404,-4.03384069239769));
#57864=CARTESIAN_POINT('Ctrl Pts',(10.2573662164723,-10.6902203144907,-2.25727553788306));
#57865=CARTESIAN_POINT('Ctrl Pts',(10.2408064194366,-10.8467419605648,-1.51600543042925));
#57866=CARTESIAN_POINT('Ctrl Pts',(10.2242466224009,-10.9244962313051,-0.758103329967473));
#57867=CARTESIAN_POINT('Ctrl Pts',(10.2076868253652,-10.924167183502,-0.000134674578820061));
#57868=CARTESIAN_POINT('Ctrl Pts',(9.99231317463481,-10.9259274088367,1.33692176457333E-5));
#57869=CARTESIAN_POINT('Ctrl Pts',(10.0316372481289,-10.9257973063143,-1.79907793928067));
#57870=CARTESIAN_POINT('Ctrl Pts',(10.0709613216229,-10.4721235095465,-3.59823246389915));
#57871=CARTESIAN_POINT('Ctrl Pts',(10.1102853951169,-9.61882726206042,-5.18209249908432));
#57872=CARTESIAN_POINT('Ctrl Pts',(10.149887073777,-8.75950723765072,-6.77713366808835));
#57873=CARTESIAN_POINT('Ctrl Pts',(10.1894887524371,-7.49490264142214,-8.15382990975378));
#57874=CARTESIAN_POINT('Ctrl Pts',(10.2290904310972,-5.97840104749487,-9.14519772786434));
#57875=CARTESIAN_POINT('Ctrl Pts',(10.2686921097572,-4.46189945356757,-10.1365655459749));
#57876=CARTESIAN_POINT('Ctrl Pts',(10.3082937884173,-2.69350086194156,-10.7426049405306));
#57877=CARTESIAN_POINT('Ctrl Pts',(10.3478954670774,-0.887699487532714,
-10.8898076285239));
#57878=CARTESIAN_POINT('Ctrl Pts',(10.3874971457375,0.918101886876135,-11.0370103165172));
#57879=CARTESIAN_POINT('Ctrl Pts',(10.4270988243975,2.76130604406783,-10.7253762979481));
#57880=CARTESIAN_POINT('Ctrl Pts',(10.4667005030576,4.41834538423843,-9.99270457043546));
#57881=CARTESIAN_POINT('Ctrl Pts',(10.5063021817177,6.07538472440902,-9.26003284292284));
#57882=CARTESIAN_POINT('Ctrl Pts',(10.5459038603778,7.54625924755853,-8.10632340646668));
#57883=CARTESIAN_POINT('Ctrl Pts',(10.5855055390378,8.65256229945373,-6.67151303832157));
#57884=CARTESIAN_POINT('Ctrl Pts',(10.6251072176979,9.75886535134895,-5.23670267017645));
#57885=CARTESIAN_POINT('Ctrl Pts',(10.664708896358,10.5005969319898,-3.52079137034244));
#57886=CARTESIAN_POINT('Ctrl Pts',(10.7043105750181,10.7877902579707,-1.73190701726606));
#57887=CARTESIAN_POINT('Ctrl Pts',(10.7439122536781,11.0749835839515,0.056977335810294));
#57888=CARTESIAN_POINT('Ctrl Pts',(10.7835139323382,10.9076386552723,1.91883474212895));
#57889=CARTESIAN_POINT('Ctrl Pts',(10.8231156109983,10.3060532256562,3.62783509497938));
#57890=CARTESIAN_POINT('Ctrl Pts',(10.8627172896584,9.70446779604009,5.33683544782982));
#57891=CARTESIAN_POINT('Ctrl Pts',(10.9023189683185,8.66864186548706,6.89297874721206));
#57892=CARTESIAN_POINT('Ctrl Pts',(10.9419206469785,7.32421377753323,8.10751584071318));
#57893=CARTESIAN_POINT('Ctrl Pts',(10.9815223256386,5.97978568957941,9.3220529342143));
#57894=CARTESIAN_POINT('Ctrl Pts',(11.0211240042987,4.32675544422477,10.1949838218343));
#57895=CARTESIAN_POINT('Ctrl Pts',(11.0607256829587,2.56562389370283,10.6204281741596));
#57896=CARTESIAN_POINT('Ctrl Pts',(11.1003273616188,0.804492343180889,11.045872526485));
#57897=CARTESIAN_POINT('Ctrl Pts',(11.1399290402789,-1.06474051250837,11.0238303435156));
#57898=CARTESIAN_POINT('Ctrl Pts',(11.179530718939,-2.81534997692229,10.5569751858128));
#57899=CARTESIAN_POINT('Ctrl Pts',(11.2191323975991,-4.56595944133621,10.0901200281099));
#57900=CARTESIAN_POINT('Ctrl Pts',(11.2587340762591,-6.1979455144748,9.17845189567358));
#57901=CARTESIAN_POINT('Ctrl Pts',(11.2983357549192,-7.51335985303518,7.93254967114748));
#57902=CARTESIAN_POINT('Ctrl Pts',(11.3379374335793,-8.82877419159556,6.68664744662138));
#57903=CARTESIAN_POINT('Ctrl Pts',(11.3775391122394,-9.82761679557775,5.10651113000551));
#57904=CARTESIAN_POINT('Ctrl Pts',(11.4171407908994,-10.3887351368242,3.38380005664291));
#57905=CARTESIAN_POINT('Ctrl Pts',(11.4421982521446,-10.7437756695854,2.29377641578027));
#57906=CARTESIAN_POINT('Ctrl Pts',(11.4672557133897,-10.9235704244,1.1466720364512));
#57907=CARTESIAN_POINT('Ctrl Pts',(11.4923131746348,-10.924327996449,-0.000200333677245087));
#57908=CARTESIAN_POINT('Origin',(21.9,0.,0.));
#57909=CARTESIAN_POINT('',(13.2076868253652,-10.9250564040338,-0.00028148019367122));
#57910=CARTESIAN_POINT('',(12.9923131746348,-10.9248434092042,0.000278809958667608));
#57911=CARTESIAN_POINT('',(21.9,-10.925,-1.33792662806848E-15));
#57912=CARTESIAN_POINT('Ctrl Pts',(13.2076868253652,-10.9250564040338,-0.00028148019367122));
#57913=CARTESIAN_POINT('Ctrl Pts',(13.1767596051944,-10.923596904997,1.41497669743632));
#57914=CARTESIAN_POINT('Ctrl Pts',(13.1458323850236,-10.6472890348987,2.83078810371605));
#57915=CARTESIAN_POINT('Ctrl Pts',(13.1149051648529,-10.1111262094871,4.14019685547656));
#57916=CARTESIAN_POINT('Ctrl Pts',(13.0752171239031,-9.42308337688983,5.82052466615086));
#57917=CARTESIAN_POINT('Ctrl Pts',(13.0355290829534,-8.30711466167061,7.32562991932744));
#57918=CARTESIAN_POINT('Ctrl Pts',(12.9958410420037,-6.89915787681248,8.47217350017636));
#57919=CARTESIAN_POINT('Ctrl Pts',(12.9561530010539,-5.49120109195431,9.61871708102531));
#57920=CARTESIAN_POINT('Ctrl Pts',(12.9164649601042,-3.7912562374572,10.4066989895466));
#57921=CARTESIAN_POINT('Ctrl Pts',(12.8767769191545,-2.00639613047163,10.740133974672));
#57922=CARTESIAN_POINT('Ctrl Pts',(12.8370888782047,-0.221536023486108,
11.0735689597973));
#57923=CARTESIAN_POINT('Ctrl Pts',(12.797400837255,1.64823933598789,10.9524570215267));
#57924=CARTESIAN_POINT('Ctrl Pts',(12.7577127963053,3.37516982379076,10.3915509856251));
#57925=CARTESIAN_POINT('Ctrl Pts',(12.7180247553556,5.10210031159368,9.8306449497235));
#57926=CARTESIAN_POINT('Ctrl Pts',(12.6783367144058,6.6861859277254,8.82994481619083));
#57927=CARTESIAN_POINT('Ctrl Pts',(12.6386486734561,7.93446684159381,7.51134736022258));
#57928=CARTESIAN_POINT('Ctrl Pts',(12.5989606325064,9.18274775546218,6.19274990425436));
#57929=CARTESIAN_POINT('Ctrl Pts',(12.5592725915566,10.0952239670672,4.55625512585054));
#57930=CARTESIAN_POINT('Ctrl Pts',(12.5195845506069,10.5607453886752,2.80120689379593));
#57931=CARTESIAN_POINT('Ctrl Pts',(12.4798965096572,11.0262668102832,1.04615866174129));
#57932=CARTESIAN_POINT('Ctrl Pts',(12.4402084687074,11.0448334418941,-0.827443023964217));
#57933=CARTESIAN_POINT('Ctrl Pts',(12.4005204277577,10.6141836544306,-2.5913719486581));
#57934=CARTESIAN_POINT('Ctrl Pts',(12.360832386808,10.1835338669672,-4.35530087335198));
#57935=CARTESIAN_POINT('Ctrl Pts',(12.3211443458583,9.30366766042947,-6.00955703703417));
#57936=CARTESIAN_POINT('Ctrl Pts',(12.2814563049085,8.08176284921606,-7.35263303009916));
#57937=CARTESIAN_POINT('Ctrl Pts',(12.2417682639588,6.85985803800267,-8.69570902316414));
#57938=CARTESIAN_POINT('Ctrl Pts',(12.2020802230091,5.29591462211355,-9.7276048456119));
#57939=CARTESIAN_POINT('Ctrl Pts',(12.1623921820593,3.58043888069976,-10.3226237288709));
#57940=CARTESIAN_POINT('Ctrl Pts',(12.1227041411096,1.86496313928596,-10.9176426121298));
#57941=CARTESIAN_POINT('Ctrl Pts',(12.0830161001599,-0.00204492765251058,
-11.0757845562));
#57942=CARTESIAN_POINT('Ctrl Pts',(12.0433280592101,-1.79316228398563,-10.7777860551027));
#57943=CARTESIAN_POINT('Ctrl Pts',(12.0036400182604,-3.58427964031875,-10.4797875540053));
#57944=CARTESIAN_POINT('Ctrl Pts',(11.9639519773107,-5.29950628604645,-9.72564860774038));
#57945=CARTESIAN_POINT('Ctrl Pts',(11.924263936361,-6.72990790624508,-8.60723200568767));
#57946=CARTESIAN_POINT('Ctrl Pts',(11.8845758954112,-8.16030952644373,-7.48881540363494));
#57947=CARTESIAN_POINT('Ctrl Pts',(11.8448878544615,-9.30588612111331,-6.00612114579443));
#57948=CARTESIAN_POINT('Ctrl Pts',(11.8051998135118,-10.0270932973329,-4.33975843024193));
#57949=CARTESIAN_POINT('Ctrl Pts',(11.7726954841296,-10.6177587735737,-2.97501476236694));
#57950=CARTESIAN_POINT('Ctrl Pts',(11.7401911547474,-10.9237768795993,-1.48707479144505));
#57951=CARTESIAN_POINT('Ctrl Pts',(11.7076868253652,-10.9252842859753,0.000263961161978608));
#57952=CARTESIAN_POINT('Ctrl Pts',(11.4923131746348,-10.924327996449,-0.000200333677245087));
#57953=CARTESIAN_POINT('Ctrl Pts',(11.5068573920498,-10.9247677174758,-0.665884735427885));
#57954=CARTESIAN_POINT('Ctrl Pts',(11.5214016094647,-10.8648890379775,-1.33149097227628));
#57955=CARTESIAN_POINT('Ctrl Pts',(11.5359458268797,-10.7439505452392,-1.98581148346912));
#57956=CARTESIAN_POINT('Ctrl Pts',(11.5755475055397,-10.4146535338969,-3.76742612010928));
#57957=CARTESIAN_POINT('Ctrl Pts',(11.6151491841998,-9.63266543270149,-5.46536956328023));
#57958=CARTESIAN_POINT('Ctrl Pts',(11.6547508628599,-8.49283585566751,-6.87369330819401));
#57959=CARTESIAN_POINT('Ctrl Pts',(11.69435254152,-7.35300627863354,-8.28201705310777));
#57960=CARTESIAN_POINT('Ctrl Pts',(11.73395422018,-5.85533522576098,-9.40072109976435));
#57961=CARTESIAN_POINT('Ctrl Pts',(11.7735558988401,-4.18147958040706,-10.0941145765769));
#57962=CARTESIAN_POINT('Ctrl Pts',(11.8131575775002,-2.50762393505313,-10.7875080533894));
#57963=CARTESIAN_POINT('Ctrl Pts',(11.8527592561603,-0.657583697217856,
-11.0555909603578));
#57964=CARTESIAN_POINT('Ctrl Pts',(11.8923609348203,1.14424436516629,-10.8658467410142));
#57965=CARTESIAN_POINT('Ctrl Pts',(11.9319626134804,2.94607242755045,-10.6761025216705));
#57966=CARTESIAN_POINT('Ctrl Pts',(11.9715642921405,4.69968831448346,-10.0285311760147));
#57967=CARTESIAN_POINT('Ctrl Pts',(12.0111659708006,6.19239084835027,-9.00167851834815));
#57968=CARTESIAN_POINT('Ctrl Pts',(12.0507676494607,7.68509338221708,-7.97482586068155));
#57969=CARTESIAN_POINT('Ctrl Pts',(12.0903693281207,8.91688256301768,-6.56869189100413));
#57970=CARTESIAN_POINT('Ctrl Pts',(12.1299710067808,9.73835109393064,-4.95383069328804));
#57971=CARTESIAN_POINT('Ctrl Pts',(12.1695726854409,10.5598196248436,-3.33896949557195));
#57972=CARTESIAN_POINT('Ctrl Pts',(12.2091743641009,10.9709675058689,-1.51538106981721));
#57973=CARTESIAN_POINT('Ctrl Pts',(12.248776042761,10.921925413217,0.295746233361029));
#57974=CARTESIAN_POINT('Ctrl Pts',(12.2883777214211,10.8728833205651,2.10687353653924));
#57975=CARTESIAN_POINT('Ctrl Pts',(12.3279794000812,10.3636512542359,3.90553971714101));
#57976=CARTESIAN_POINT('Ctrl Pts',(12.3675810787413,9.45599545448473,5.47357931624151));
#57977=CARTESIAN_POINT('Ctrl Pts',(12.4071827574013,8.54833965473349,7.04161891534205));
#57978=CARTESIAN_POINT('Ctrl Pts',(12.4467844360614,7.24226012156024,8.37903193294132));
#57979=CARTESIAN_POINT('Ctrl Pts',(12.4863861147215,5.69617504496584,9.32359964946647));
#57980=CARTESIAN_POINT('Ctrl Pts',(12.5259877933816,4.15008996837146,10.2681673659916));
#57981=CARTESIAN_POINT('Ctrl Pts',(12.5655894720416,2.36399934835599,10.8198897814425));
#57982=CARTESIAN_POINT('Ctrl Pts',(12.6051911507017,0.554543317479457,10.9118468773834));
#57983=CARTESIAN_POINT('Ctrl Pts',(12.6447928293618,-1.25491271339705,11.0038039733242));
#57984=CARTESIAN_POINT('Ctrl Pts',(12.6843945080219,-3.0877341551347,10.635995749755));
#57985=CARTESIAN_POINT('Ctrl Pts',(12.7239961866819,-4.72161275772225,9.85303473720342));
#57986=CARTESIAN_POINT('Ctrl Pts',(12.763597865342,-6.35549136030983,9.07007372465182));
#57987=CARTESIAN_POINT('Ctrl Pts',(12.8031995440021,-7.79042712374736,7.87195992311785));
#57988=CARTESIAN_POINT('Ctrl Pts',(12.8428012226622,-8.85237251062407,6.40401604460592));
#57989=CARTESIAN_POINT('Ctrl Pts',(12.8824029013222,-9.91431789750078,4.936072166094));
#57990=CARTESIAN_POINT('Ctrl Pts',(12.9220045799823,-10.6032729078167,3.19829821060413));
#57991=CARTESIAN_POINT('Ctrl Pts',(12.9616062586424,-10.8356721820708,1.4014738417535));
#57992=CARTESIAN_POINT('Ctrl Pts',(12.9718418973065,-10.8957392064384,0.937058049172143));
#57993=CARTESIAN_POINT('Ctrl Pts',(12.9820775359707,-10.9253064649804,0.468697450651115));
#57994=CARTESIAN_POINT('Ctrl Pts',(12.9923131746348,-10.9248434092042,0.000278809958667608));
#57995=CARTESIAN_POINT('Origin',(21.9,0.,0.));
#57996=CARTESIAN_POINT('',(14.7076868253652,-10.9242850111832,0.000189904277848944));
#57997=CARTESIAN_POINT('',(14.4923131746348,-10.9256212207963,-0.00019638491873492));
#57998=CARTESIAN_POINT('',(21.9,-10.925,-1.33792662806848E-15));
#57999=CARTESIAN_POINT('Ctrl Pts',(14.7076868253652,-10.9242850111832,0.000189904277848944));
#58000=CARTESIAN_POINT('Ctrl Pts',(14.6927041375409,-10.9247106493509,0.685950548282512));
#58001=CARTESIAN_POINT('Ctrl Pts',(14.6777214497166,-10.8611501816942,1.37163326897208));
#58002=CARTESIAN_POINT('Ctrl Pts',(14.6627387618924,-10.7328539348121,2.0449815745532));
#58003=CARTESIAN_POINT('Ctrl Pts',(14.6230507209426,-10.3930065883499,3.82863184069748));
#58004=CARTESIAN_POINT('Ctrl Pts',(14.5833626799929,-9.59892042635426,5.52573383050678));
#58005=CARTESIAN_POINT('Ctrl Pts',(14.5436746390432,-8.44732426810974,6.9295610204167));
#58006=CARTESIAN_POINT('Ctrl Pts',(14.5039865980934,-7.29572810986518,8.33338821032666));
#58007=CARTESIAN_POINT('Ctrl Pts',(14.4642985571437,-5.78662195537179,9.44394060033721));
#58008=CARTESIAN_POINT('Ctrl Pts',(14.424610516194,-4.10383227521378,10.125940148114));
#58009=CARTESIAN_POINT('Ctrl Pts',(14.3849224752442,-2.42104259505577,10.8079396958909));
#58010=CARTESIAN_POINT('Ctrl Pts',(14.3452344342945,-0.564569389233146,
11.061386401434));
#58011=CARTESIAN_POINT('Ctrl Pts',(14.3055463933448,1.23944757326274,10.855407543681));
#58012=CARTESIAN_POINT('Ctrl Pts',(14.2658583523951,3.04346453575858,10.6494286859281));
#58013=CARTESIAN_POINT('Ctrl Pts',(14.2261703114453,4.79502525492768,9.98402426487906));
#58014=CARTESIAN_POINT('Ctrl Pts',(14.1864822704956,6.28076950819055,8.94024818510415));
#58015=CARTESIAN_POINT('Ctrl Pts',(14.1467942295459,7.76651376145342,7.89647210532924));
#58016=CARTESIAN_POINT('Ctrl Pts',(14.1071061885961,8.98644154881006,6.47432436682845));
#58017=CARTESIAN_POINT('Ctrl Pts',(14.0674181476464,9.79195164770917,4.84703890588883));
#58018=CARTESIAN_POINT('Ctrl Pts',(14.0277301066967,10.5974617466083,3.21975344494919));
#58019=CARTESIAN_POINT('Ctrl Pts',(13.9880420657469,10.9885541570499,1.38733026157065));
#58020=CARTESIAN_POINT('Ctrl Pts',(13.9483540247972,10.9175893294438,-0.427020444345068));
#58021=CARTESIAN_POINT('Ctrl Pts',(13.9086659838475,10.8466245018377,-2.24137115026071));
#58022=CARTESIAN_POINT('Ctrl Pts',(13.8689779428978,10.3136024361841,-4.03764937871359));
#58023=CARTESIAN_POINT('Ctrl Pts',(13.829289901948,9.38345134497521,-5.59704780064966));
#58024=CARTESIAN_POINT('Ctrl Pts',(13.7896018609983,8.4533002537663,-7.15644622258583));
#58025=CARTESIAN_POINT('Ctrl Pts',(13.7499138200486,7.12602013700219,-8.47896483800514));
#58026=CARTESIAN_POINT('Ctrl Pts',(13.7102257790988,5.56328896452938,-9.40350568263878));
#58027=CARTESIAN_POINT('Ctrl Pts',(13.6705377381491,4.00055779205657,-10.3280465272724));
#58028=CARTESIAN_POINT('Ctrl Pts',(13.6308496971994,2.20237556387508,-10.8546096011204));
#58029=CARTESIAN_POINT('Ctrl Pts',(13.5911616562496,0.387781538084555,-10.9190534711116));
#58030=CARTESIAN_POINT('Ctrl Pts',(13.5514736152999,-1.42681248770592,-10.9834973411029));
#58031=CARTESIAN_POINT('Ctrl Pts',(13.5117855743502,-3.2578183111054,-10.5858220072375));
#58032=CARTESIAN_POINT('Ctrl Pts',(13.4720975334004,-4.88219838294451,-9.77446889482228));
#58033=CARTESIAN_POINT('Ctrl Pts',(13.4324094924507,-6.50657845478361,-8.96311578240702));
#58034=CARTESIAN_POINT('Ctrl Pts',(13.392721451501,-7.92433277506231,-7.7380848914419));
#58035=CARTESIAN_POINT('Ctrl Pts',(13.3530334105513,-8.96276257631729,-6.24859906113686));
#58036=CARTESIAN_POINT('Ctrl Pts',(13.3133453696015,-10.0011923775723,-4.75911323083179));
#58037=CARTESIAN_POINT('Ctrl Pts',(13.2736573286518,-10.6602976598035,-3.0051724611868));
#58038=CARTESIAN_POINT('Ctrl Pts',(13.2339692877021,-10.8597918259315,-1.20042689227826));
#58039=CARTESIAN_POINT('Ctrl Pts',(13.2252084669231,-10.9038285834552,-0.802043598407917));
#58040=CARTESIAN_POINT('Ctrl Pts',(13.2164476461442,-10.9254698394935,-0.40118473569794));
#58041=CARTESIAN_POINT('Ctrl Pts',(13.2076868253652,-10.9250564040338,-0.00028148019367122));
#58042=CARTESIAN_POINT('Ctrl Pts',(12.9923131746348,-10.9248434092042,0.000278809958667608));
#58043=CARTESIAN_POINT('Ctrl Pts',(13.0216792146307,-10.923514902514,-1.34361393467423));
#58044=CARTESIAN_POINT('Ctrl Pts',(13.0510452546267,-10.6750021672134,-2.68798443352631));
#58045=CARTESIAN_POINT('Ctrl Pts',(13.0804112946226,-10.1903913866649,-3.9410460480701));
#58046=CARTESIAN_POINT('Ctrl Pts',(13.1200129732827,-9.53686777881229,-5.63086678683168));
#58047=CARTESIAN_POINT('Ctrl Pts',(13.1596146519428,-8.45397702491467,-7.15463348214339));
#58048=CARTESIAN_POINT('Ctrl Pts',(13.1992163306028,-7.07306609798857,-8.32752403418373));
#58049=CARTESIAN_POINT('Ctrl Pts',(13.2388180092629,-5.69215517106246,-9.50041458622407));
#58050=CARTESIAN_POINT('Ctrl Pts',(13.278419687923,-4.01322407110788,-10.322428994993));
#58051=CARTESIAN_POINT('Ctrl Pts',(13.3180213665831,-2.23991524043845,-10.6938627390702));
#58052=CARTESIAN_POINT('Ctrl Pts',(13.3576230452432,-0.466606409769066,
-11.0652964831474));
#58053=CARTESIAN_POINT('Ctrl Pts',(13.3972247239032,1.40108015161521,-10.9861495625329));
#58054=CARTESIAN_POINT('Ctrl Pts',(13.4368264025633,3.13660730181091,-10.4660219377111));
#58055=CARTESIAN_POINT('Ctrl Pts',(13.4764280812234,4.87213445200664,-9.94589431288922));
#58056=CARTESIAN_POINT('Ctrl Pts',(13.5160297598834,6.47550219101383,-8.98478598386001));
#58057=CARTESIAN_POINT('Ctrl Pts',(13.5556314385435,7.75223337661556,-7.69927257868629));
#58058=CARTESIAN_POINT('Ctrl Pts',(13.5952331172036,9.0289645622173,-6.41375917351256));
#58059=CARTESIAN_POINT('Ctrl Pts',(13.6348347958637,9.97905919441357,-4.80384069219434));
#58060=CARTESIAN_POINT('Ctrl Pts',(13.6744364745238,10.4872775285034,-3.06478883555969));
#58061=CARTESIAN_POINT('Ctrl Pts',(13.7140381531838,10.9954958625931,-1.32573697892507));
#58062=CARTESIAN_POINT('Ctrl Pts',(13.7536398318439,11.0618378985764,0.542448253025954));
#58063=CARTESIAN_POINT('Ctrl Pts',(13.793241510504,10.6782568177147,2.31316923318468));
#58064=CARTESIAN_POINT('Ctrl Pts',(13.8328431891641,10.294675736853,4.08389021334341));
#58065=CARTESIAN_POINT('Ctrl Pts',(13.8724448678241,9.46117153914633,5.75714694170988));
#58066=CARTESIAN_POINT('Ctrl Pts',(13.9120465464842,8.27884237597458,7.12998523702471));
#58067=CARTESIAN_POINT('Ctrl Pts',(13.9516482251443,7.09651321280282,8.50282353233955));
#58068=CARTESIAN_POINT('Ctrl Pts',(13.9912499038044,5.565359084166,9.57524339460272));
#58069=CARTESIAN_POINT('Ctrl Pts',(14.0308515824644,3.87109813318651,10.2171678957362));
#58070=CARTESIAN_POINT('Ctrl Pts',(14.0704532611245,2.17683718220705,10.8590923968697));
#58071=CARTESIAN_POINT('Ctrl Pts',(14.1100549397846,0.319469408884921,11.0705215368734));
#58072=CARTESIAN_POINT('Ctrl Pts',(14.1496566184447,-1.47571964072968,10.8258104596555));
#58073=CARTESIAN_POINT('Ctrl Pts',(14.1892582971048,-3.27090869034427,10.5810993824376));
#58074=CARTESIAN_POINT('Ctrl Pts',(14.2288599757648,-5.00391901625139,9.88024808799808));
#58075=CARTESIAN_POINT('Ctrl Pts',(14.2684616544249,-6.46454874933802,8.80826487078216));
#58076=CARTESIAN_POINT('Ctrl Pts',(14.308063333085,-7.92517848242467,7.73628165356621));
#58077=CARTESIAN_POINT('Ctrl Pts',(14.3476650117451,-9.11342762269081,6.29316651357394));
#58078=CARTESIAN_POINT('Ctrl Pts',(14.3872666904051,-9.88516997162404,4.65395908861747));
#58079=CARTESIAN_POINT('Ctrl Pts',(14.4222821851484,-10.5675385245874,3.20458469556979));
#58080=CARTESIAN_POINT('Ctrl Pts',(14.4572976798916,-10.9242838098394,1.601906174158));
#58081=CARTESIAN_POINT('Ctrl Pts',(14.4923131746348,-10.9256212207963,-0.00019638491873492));
#58082=CARTESIAN_POINT('Origin',(21.9,0.,0.));
#58083=CARTESIAN_POINT('',(16.2076868253652,-10.9259207307055,-4.64929610923717E-5));
#58084=CARTESIAN_POINT('',(15.9923131746348,-10.9240749080107,-1.66041913914505E-5));
#58085=CARTESIAN_POINT('',(21.9,-10.925,-1.33792662806848E-15));
#58086=CARTESIAN_POINT('Ctrl Pts',(16.2076868253652,-10.9259207307055,-4.64929610923717E-5));
#58087=CARTESIAN_POINT('Ctrl Pts',(16.1689606289377,-10.925497342121,1.77169465316328));
#58088=CARTESIAN_POINT('Ctrl Pts',(16.1302344325102,-10.486075079379,3.54363821346978));
#58089=CARTESIAN_POINT('Ctrl Pts',(16.0915082360827,-9.65749661830683,5.10968318916803));
#58090=CARTESIAN_POINT('Ctrl Pts',(16.0518201951329,-8.80833871160026,6.71462410405917));
#58091=CARTESIAN_POINT('Ctrl Pts',(16.0121321541832,-7.55045355941333,8.10331159244359));
#58092=CARTESIAN_POINT('Ctrl Pts',(15.9724441132335,-6.03706602749741,9.10658756098633));
#58093=CARTESIAN_POINT('Ctrl Pts',(15.9327560722837,-4.52367849558144,10.1098635295291));
#58094=CARTESIAN_POINT('Ctrl Pts',(15.893068031334,-2.75478858393648,10.7277279782301));
#58095=CARTESIAN_POINT('Ctrl Pts',(15.8533799903843,-0.945867409913358,
10.8849179174277));
#58096=CARTESIAN_POINT('Ctrl Pts',(15.8136919494345,0.863053764109711,11.0421078566252));
#58097=CARTESIAN_POINT('Ctrl Pts',(15.7740039084848,2.71200620051092,10.7386232863193));
#58098=CARTESIAN_POINT('Ctrl Pts',(15.7343158675351,4.37576624643479,10.0114321144797));
#58099=CARTESIAN_POINT('Ctrl Pts',(15.6946278265854,6.03952629235865,9.2842409426402));
#58100=CARTESIAN_POINT('Ctrl Pts',(15.6549397856356,7.51809394780516,8.13334316926709));
#58101=CARTESIAN_POINT('Ctrl Pts',(15.6152517446859,8.63136268228842,6.69893136799245));
#58102=CARTESIAN_POINT('Ctrl Pts',(15.5755637037362,9.74463141677171,5.26451956671777));
#58103=CARTESIAN_POINT('Ctrl Pts',(15.5358756627864,10.4926012302917,3.54659373754155));
#58104=CARTESIAN_POINT('Ctrl Pts',(15.4961876218367,10.7841608047258,1.75441698694747));
#58105=CARTESIAN_POINT('Ctrl Pts',(15.456499580887,11.0757203791599,-0.0377597636465252));
#58106=CARTESIAN_POINT('Ctrl Pts',(15.4168115399372,10.910869714508,-1.90418743565843));
#58107=CARTESIAN_POINT('Ctrl Pts',(15.3771234989875,10.3096895160051,-3.61751369172929));
#58108=CARTESIAN_POINT('Ctrl Pts',(15.3374354580378,9.70850931750215,-5.33083994780018));
#58109=CARTESIAN_POINT('Ctrl Pts',(15.2977474170881,8.67099958514808,-6.89106478793008));
#58110=CARTESIAN_POINT('Ctrl Pts',(15.2580593761383,7.32354092624979,-8.10813489822527));
#58111=CARTESIAN_POINT('Ctrl Pts',(15.2183713351886,5.97608226735146,-9.32520500852049));
#58112=CARTESIAN_POINT('Ctrl Pts',(15.1786832942389,4.3186746819089,-10.199120388981));
#58113=CARTESIAN_POINT('Ctrl Pts',(15.1389952532891,2.55320945891076,-10.6234281042045));
#58114=CARTESIAN_POINT('Ctrl Pts',(15.0993072123394,0.787744235912617,-11.0477358194281));
#58115=CARTESIAN_POINT('Ctrl Pts',(15.0596191713897,-1.08577862464108,-11.0224358694147));
#58116=CARTESIAN_POINT('Ctrl Pts',(15.0199311304399,-2.83914250989711,-10.5506100787949));
#58117=CARTESIAN_POINT('Ctrl Pts',(14.9802430894902,-4.59250639515309,-10.0787842881751));
#58118=CARTESIAN_POINT('Ctrl Pts',(14.9405550485405,-6.22571130511138,-9.16043265694893));
#58119=CARTESIAN_POINT('Ctrl Pts',(14.9008670075907,-7.53981411476752,-7.90742096647363));
#58120=CARTESIAN_POINT('Ctrl Pts',(14.861178966641,-8.85391692442365,-6.65440927599832));
#58121=CARTESIAN_POINT('Ctrl Pts',(14.8214909256913,-9.84891763377762,-5.06673752627394));
#58122=CARTESIAN_POINT('Ctrl Pts',(14.7818028847416,-10.4036137229903,-3.33780238017213));
#58123=CARTESIAN_POINT('Ctrl Pts',(14.7570975316161,-10.7489057160786,-2.26155995819044));
#58124=CARTESIAN_POINT('Ctrl Pts',(14.7323921784907,-10.9235831650685,-1.13057909180407));
#58125=CARTESIAN_POINT('Ctrl Pts',(14.7076868253652,-10.9242850111832,0.000189904277848944));
#58126=CARTESIAN_POINT('Ctrl Pts',(14.4923131746348,-10.9256212207963,-0.00019638491873492));
#58127=CARTESIAN_POINT('Ctrl Pts',(14.4968993585516,-10.9257963893229,-0.210033117013062));
#58128=CARTESIAN_POINT('Ctrl Pts',(14.5014855424685,-10.9198746526023,-0.419859968662869));
#58129=CARTESIAN_POINT('Ctrl Pts',(14.5060717263853,-10.9077890891653,-0.629331194768391));
#58130=CARTESIAN_POINT('Ctrl Pts',(14.5456734050454,-10.8034303001731,-2.4381143432772));
#58131=CARTESIAN_POINT('Ctrl Pts',(14.5852750837055,-10.2394771645883,-4.22038093037418));
#58132=CARTESIAN_POINT('Ctrl Pts',(14.6248767623656,-9.28433320050895,-5.75995465158798));
#58133=CARTESIAN_POINT('Ctrl Pts',(14.6644784410257,-8.32918923642961,-7.2995283728017));
#58134=CARTESIAN_POINT('Ctrl Pts',(14.7040801196857,-6.98285444385562,-8.59640922813228));
#58135=CARTESIAN_POINT('Ctrl Pts',(14.7436817983458,-5.40862969042774,-9.49329476200157));
#58136=CARTESIAN_POINT('Ctrl Pts',(14.7832834770059,-3.83440493699978,-10.3901802958709));
#58137=CARTESIAN_POINT('Ctrl Pts',(14.822885155666,-2.0322902227179,-10.887070508279));
#58138=CARTESIAN_POINT('Ctrl Pts',(14.862486834326,-0.220869289199256,-10.9236961383733));
#58139=CARTESIAN_POINT('Ctrl Pts',(14.9020885129861,1.59055164431939,-10.9603217684676));
#58140=CARTESIAN_POINT('Ctrl Pts',(14.9416901916462,3.41127879707475,-10.5366828162482));
#58141=CARTESIAN_POINT('Ctrl Pts',(14.9812918703063,5.0204708705861,-9.70416368390492));
#58142=CARTESIAN_POINT('Ctrl Pts',(15.0208935489663,6.62966294409743,-8.87164455156165));
#58143=CARTESIAN_POINT('Ctrl Pts',(15.0604952276264,8.02731993836476,-7.63024523909446));
#58144=CARTESIAN_POINT('Ctrl Pts',(15.1000969062865,9.04391596644903,-6.13053868418029));
#58145=CARTESIAN_POINT('Ctrl Pts',(15.1396985849466,10.0605119945333,-4.63083212926609));
#58146=CARTESIAN_POINT('Ctrl Pts',(15.1793002636066,10.6960470564346,-2.87281833190489));
#58147=CARTESIAN_POINT('Ctrl Pts',(15.2189019422667,10.873435253759,-1.06973190507467));
#58148=CARTESIAN_POINT('Ctrl Pts',(15.2585036209268,11.0508234510833,0.73335452175556));
#58149=CARTESIAN_POINT('Ctrl Pts',(15.2981052995869,10.7700647838307,2.58151357805476));
#58150=CARTESIAN_POINT('Ctrl Pts',(15.3377069782469,10.0652132883471,4.25057666987718));
#58151=CARTESIAN_POINT('Ctrl Pts',(15.377308656907,9.36036179286343,5.91963976169957));
#58152=CARTESIAN_POINT('Ctrl Pts',(15.4169103355671,8.23141746914867,7.40960688904521));
#58153=CARTESIAN_POINT('Ctrl Pts',(15.4565120142272,6.81531326181477,8.53975560011845));
#58154=CARTESIAN_POINT('Ctrl Pts',(15.4961136928873,5.39920905448085,9.66990431119172));
#58155=CARTESIAN_POINT('Ctrl Pts',(15.5357153715473,3.69594496352779,10.4402346059926));
#58156=CARTESIAN_POINT('Ctrl Pts',(15.5753170502074,1.91211485060719,10.7573108797929));
#58157=CARTESIAN_POINT('Ctrl Pts',(15.6149187288675,0.128284737686591,11.0743871535931));
#58158=CARTESIAN_POINT('Ctrl Pts',(15.6545204075276,-1.73611139720149,10.9382094063928));
#58159=CARTESIAN_POINT('Ctrl Pts',(15.6941220861876,-3.45493551756541,10.3652950337117));
#58160=CARTESIAN_POINT('Ctrl Pts',(15.7337237648477,-5.1737596379293,9.79238066103058));
#58161=CARTESIAN_POINT('Ctrl Pts',(15.7733254435078,-6.74701174376905,8.78272966286875));
#58162=CARTESIAN_POINT('Ctrl Pts',(15.8129271221679,-7.98386750571404,7.45880554898881));
#58163=CARTESIAN_POINT('Ctrl Pts',(15.8525288008279,-9.22072326765904,6.13488143510886));
#58164=CARTESIAN_POINT('Ctrl Pts',(15.892130479488,-10.1211826857093,4.4966842055108));
#58165=CARTESIAN_POINT('Ctrl Pts',(15.9317321581481,-10.5760264148298,2.74291557275187));
#58166=CARTESIAN_POINT('Ctrl Pts',(15.9519258303103,-10.8079601474817,1.84863457213206));
#58167=CARTESIAN_POINT('Ctrl Pts',(15.9721195024726,-10.9240257803778,0.92430292652148));
#58168=CARTESIAN_POINT('Ctrl Pts',(15.9923131746348,-10.9240749080107,-1.66041913914505E-5));
#58169=CARTESIAN_POINT('Origin',(21.9,0.,0.));
#58170=CARTESIAN_POINT('',(17.7076868253652,-10.9241469997933,-0.000121431705876017));
#58171=CARTESIAN_POINT('',(17.4923131746348,-10.9255250468596,0.000220564452133845));
#58172=CARTESIAN_POINT('',(21.9,-10.925,-1.33792662806848E-15));
#58173=CARTESIAN_POINT('Ctrl Pts',(17.7076868253652,-10.9241469997933,-0.000121431705876017));
#58174=CARTESIAN_POINT('Ctrl Pts',(17.6849051612842,-10.9237397718092,1.04263764050594));
#58175=CARTESIAN_POINT('Ctrl Pts',(17.6621234972032,-10.7755775513635,2.08551002071988));
#58176=CARTESIAN_POINT('Ctrl Pts',(17.6393418331222,-10.4812535539502,3.08535689411804));
#58177=CARTESIAN_POINT('Ctrl Pts',(17.5996537921724,-9.96851037503723,4.8271946946299));
#58178=CARTESIAN_POINT('Ctrl Pts',(17.5599657512227,-9.01217668156319,6.43845316651263));
#58179=CARTESIAN_POINT('Ctrl Pts',(17.520277710273,-7.7287449065147,7.72286251310336));
#58180=CARTESIAN_POINT('Ctrl Pts',(17.4805896693232,-6.44531313146618,9.00727185969413));
#58181=CARTESIAN_POINT('Ctrl Pts',(17.4409016283735,-4.83478327484319,9.96483208099287));
#58182=CARTESIAN_POINT('Ctrl Pts',(17.4012135874238,-3.09333637959754,10.47890133883));
#58183=CARTESIAN_POINT('Ctrl Pts',(17.361525546474,-1.35188948435184,10.9929705966671));
#58184=CARTESIAN_POINT('Ctrl Pts',(17.3218375055243,0.520474449516534,11.0635488910425));
#58185=CARTESIAN_POINT('Ctrl Pts',(17.2821494645746,2.29567997974171,10.6820389746943));
#58186=CARTESIAN_POINT('Ctrl Pts',(17.2424614236248,4.07088550996683,10.300529058346));
#58187=CARTESIAN_POINT('Ctrl Pts',(17.2027733826751,5.74893263654875,9.46693093127401));
#58188=CARTESIAN_POINT('Ctrl Pts',(17.1630853417254,7.12541593722142,8.28278642413682));
#58189=CARTESIAN_POINT('Ctrl Pts',(17.1233973007757,8.50189923789409,7.09864191699962));
#58190=CARTESIAN_POINT('Ctrl Pts',(17.0837092598259,9.57681871265749,5.5639510297972));
#58191=CARTESIAN_POINT('Ctrl Pts',(17.0440212188762,10.2192368177082,3.86565674754899));
#58192=CARTESIAN_POINT('Ctrl Pts',(17.0043331779265,10.861654922759,2.16736246530074));
#58193=CARTESIAN_POINT('Ctrl Pts',(16.9646451369767,11.071571658097,0.305464788006678));
#58194=CARTESIAN_POINT('Ctrl Pts',(16.924957096027,10.8234167532288,-1.49323575238463));
#58195=CARTESIAN_POINT('Ctrl Pts',(16.8852690550773,10.5752618483607,-3.29193629277588));
#58196=CARTESIAN_POINT('Ctrl Pts',(16.8455810141275,9.86903530328639,-5.02743969626439));
#58197=CARTESIAN_POINT('Ctrl Pts',(16.8058929731778,8.79076362636478,-6.48834170583333));
#58198=CARTESIAN_POINT('Ctrl Pts',(16.7662049322281,7.71249194944316,-7.94924371540227));
#58199=CARTESIAN_POINT('Ctrl Pts',(16.7265168912783,6.26217514067423,-9.13554433105165));
#58200=CARTESIAN_POINT('Ctrl Pts',(16.6868288503286,4.61647845279128,-9.90273850615011));
#58201=CARTESIAN_POINT('Ctrl Pts',(16.6471408093789,2.97078176490829,-10.6699326812486));
#58202=CARTESIAN_POINT('Ctrl Pts',(16.6074527684292,1.12970519791126,-11.0180204157961));
#58203=CARTESIAN_POINT('Ctrl Pts',(16.5677647274794,-0.68248696673842,-10.9046006238884));
#58204=CARTESIAN_POINT('Ctrl Pts',(16.5280766865297,-2.49467913138805,-10.7911808319806));
#58205=CARTESIAN_POINT('Ctrl Pts',(16.48838864558,-4.27798689369034,-10.2162535136175));
#58206=CARTESIAN_POINT('Ctrl Pts',(16.4487006046302,-5.81518287641051,-9.24985142260005));
#58207=CARTESIAN_POINT('Ctrl Pts',(16.4090125636805,-7.35237885913073,-8.28344933158258));
#58208=CARTESIAN_POINT('Ctrl Pts',(16.3693245227308,-8.64346306226881,-6.92557246791073));
#58209=CARTESIAN_POINT('Ctrl Pts',(16.329636481781,-9.53116659418101,-5.3416258367881));
#58210=CARTESIAN_POINT('Ctrl Pts',(16.2899484408313,-10.4188701260932,-3.75767920566548));
#58211=CARTESIAN_POINT('Ctrl Pts',(16.2502603998816,-10.9031929867795,-1.94766280709209));
#58212=CARTESIAN_POINT('Ctrl Pts',(16.2105723589318,-10.9251390865096,-0.132057437106436));
#58213=CARTESIAN_POINT('Ctrl Pts',(16.2096105144096,-10.9256709529183,-0.0880560191016058));
#58214=CARTESIAN_POINT('Ctrl Pts',(16.2086486698874,-10.9259312464294,-0.0440513184638894));
#58215=CARTESIAN_POINT('Ctrl Pts',(16.2076868253652,-10.9259207307055,-4.64929610923717E-5));
#58216=CARTESIAN_POINT('Ctrl Pts',(15.9923131746348,-10.9240749080107,-1.66041913914505E-5));
#58217=CARTESIAN_POINT('Ctrl Pts',(16.0117211811326,-10.9241221242581,-0.888374071521812));
#58218=CARTESIAN_POINT('Ctrl Pts',(16.0311291876305,-10.8170048177228,-1.7767203483131));
#58219=CARTESIAN_POINT('Ctrl Pts',(16.0505371941283,-10.6025912395345,-2.63836683836235));
#58220=CARTESIAN_POINT('Ctrl Pts',(16.0901388727884,-10.1650842949278,-4.39654058079809));
#58221=CARTESIAN_POINT('Ctrl Pts',(16.1297405514485,-9.28084236552374,-6.04354802974975));
#58222=CARTESIAN_POINT('Ctrl Pts',(16.1693422301085,-8.05711772993261,-7.37961885549847));
#58223=CARTESIAN_POINT('Ctrl Pts',(16.2089439087686,-6.83339309434154,-8.71568968124711));
#58224=CARTESIAN_POINT('Ctrl Pts',(16.2485455874287,-5.27018575256344,-9.74082388379285));
#58225=CARTESIAN_POINT('Ctrl Pts',(16.2881472660888,-3.55710167528453,-10.3306799504249));
#58226=CARTESIAN_POINT('Ctrl Pts',(16.3277489447489,-1.84401759800552,-10.920536017057));
#58227=CARTESIAN_POINT('Ctrl Pts',(16.3673506234089,0.0189432147743154,
-11.0751139477753));
#58228=CARTESIAN_POINT('Ctrl Pts',(16.406952302069,1.80581682096157,-10.775664535218));
#58229=CARTESIAN_POINT('Ctrl Pts',(16.4465539807291,3.59269042714872,-10.4762151226608));
#58230=CARTESIAN_POINT('Ctrl Pts',(16.4861556593892,5.30347682674344,-9.7227383668279));
#58231=CARTESIAN_POINT('Ctrl Pts',(16.5257573380492,6.730669755373,-8.60662565762738));
#58232=CARTESIAN_POINT('Ctrl Pts',(16.5653590167093,8.15786268400264,-7.4905129484268));
#58233=CARTESIAN_POINT('Ctrl Pts',(16.6049606953694,9.30146214166717,-6.01176428585859));
#58234=CARTESIAN_POINT('Ctrl Pts',(16.6445623740295,10.022757619881,-4.34974140145602));
#58235=CARTESIAN_POINT('Ctrl Pts',(16.6841640526895,10.7440530980948,-2.6877185170535));
#58236=CARTESIAN_POINT('Ctrl Pts',(16.7237657313496,11.0430445968578,-0.842421410816738));
#58237=CARTESIAN_POINT('Ctrl Pts',(16.7633674100097,10.8834665665946,0.96232845756576));
#58238=CARTESIAN_POINT('Ctrl Pts',(16.8029690886698,10.7238885363314,2.76707832594826));
#58239=CARTESIAN_POINT('Ctrl Pts',(16.8425707673298,10.105740977042,4.53128095647652));
#58240=CARTESIAN_POINT('Ctrl Pts',(16.8821724459899,9.10400080629451,6.04095107457523));
#58241=CARTESIAN_POINT('Ctrl Pts',(16.92177412465,8.10226063554708,7.55062119267389));
#58242=CARTESIAN_POINT('Ctrl Pts',(16.9613758033101,6.71692785334159,8.80575879834305));
#58243=CARTESIAN_POINT('Ctrl Pts',(17.0009774819701,5.11603350704683,9.65412459631618));
#58244=CARTESIAN_POINT('Ctrl Pts',(17.0405791606302,3.51513916075197,10.5024903942894));
#58245=CARTESIAN_POINT('Ctrl Pts',(17.0801808392903,1.69868325036779,10.9440843845665));
#58246=CARTESIAN_POINT('Ctrl Pts',(17.1197825179504,-0.113010997050352,
10.925344346105));
#58247=CARTESIAN_POINT('Ctrl Pts',(17.1593841966104,-1.92470524446839,10.9066043076435));
#58248=CARTESIAN_POINT('Ctrl Pts',(17.1989858752705,-3.7316378289204,10.4275302404434));
#58249=CARTESIAN_POINT('Ctrl Pts',(17.2385875539306,-5.31464063528618,9.54623043322273));
#58250=CARTESIAN_POINT('Ctrl Pts',(17.2781892325907,-6.89764344165204,8.66493062600198));
#58251=CARTESIAN_POINT('Ctrl Pts',(17.3177909112507,-8.25671646993164,7.38140507876055));
#58252=CARTESIAN_POINT('Ctrl Pts',(17.3573925899108,-9.22701379478065,5.85133634286651));
#58253=CARTESIAN_POINT('Ctrl Pts',(17.3969942685709,-10.1973111196296,4.32126760697252));
#58254=CARTESIAN_POINT('Ctrl Pts',(17.436595947231,-10.7788327410481,2.54465568242592));
#58255=CARTESIAN_POINT('Ctrl Pts',(17.4761976258911,-10.9010442081302,0.736991003210511));
#58256=CARTESIAN_POINT('Ctrl Pts',(17.4815694754723,-10.9176218290918,0.49178668160984));
#58257=CARTESIAN_POINT('Ctrl Pts',(17.4869413250536,-10.9257480912012,0.246010985806838));
#58258=CARTESIAN_POINT('Ctrl Pts',(17.4923131746348,-10.9255250468596,0.000220564452133845));
#58259=CARTESIAN_POINT('Origin',(21.9,0.,0.));
#58260=CARTESIAN_POINT('',(19.2076868253652,-10.9253333599821,0.000257774600414338));
#58261=CARTESIAN_POINT('',(18.9923131746348,-10.9249542541001,-0.00028052102294644));
#58262=CARTESIAN_POINT('',(21.9,-10.925,-1.33792662806848E-15));
#58263=CARTESIAN_POINT('Ctrl Pts',(19.2076868253652,-10.9253333599821,0.000257774600414338));
#58264=CARTESIAN_POINT('Ctrl Pts',(19.2008496936307,-10.9256465756084,0.313108382291331));
#58265=CARTESIAN_POINT('Ctrl Pts',(19.1940125618962,-10.912477062548,0.625932705642993));
#58266=CARTESIAN_POINT('Ctrl Pts',(19.1871754301617,-10.8856349415437,0.937579407686716));
#58267=CARTESIAN_POINT('Ctrl Pts',(19.1474873892119,-10.7298223524402,2.74661974109307));
#58268=CARTESIAN_POINT('Ctrl Pts',(19.1077993482622,-10.1133049077402,4.51597957924599));
#58269=CARTESIAN_POINT('Ctrl Pts',(19.0681113073125,-9.11118151653967,6.03013056234606));
#58270=CARTESIAN_POINT('Ctrl Pts',(19.0284232663627,-8.1090581253392,7.54428154544608));
#58271=CARTESIAN_POINT('Ctrl Pts',(18.988735225413,-6.7213287876383,8.80322367349329));
#58272=CARTESIAN_POINT('Ctrl Pts',(18.9490471844633,-5.11703488300871,9.65360332893093));
#58273=CARTESIAN_POINT('Ctrl Pts',(18.9093591435135,-3.51274097837912,10.5039829843686));
#58274=CARTESIAN_POINT('Ctrl Pts',(18.8696711025638,-1.6918825068208,10.9458001671966));
#58275=CARTESIAN_POINT('Ctrl Pts',(18.8299830616141,0.123739046553112,10.9252364676758));
#58276=CARTESIAN_POINT('Ctrl Pts',(18.7902950206644,1.93936059992708,10.9046727681549));
#58277=CARTESIAN_POINT('Ctrl Pts',(18.7506069797146,3.74974523511668,10.421728186285));
#58278=CARTESIAN_POINT('Ctrl Pts',(18.7109189387649,5.33436730063216,9.53523092159915));
#58279=CARTESIAN_POINT('Ctrl Pts',(18.6712308978151,6.91898936614763,8.64873365691327));
#58280=CARTESIAN_POINT('Ctrl Pts',(18.6315428568654,8.277848861989,7.35868370941133));
#58281=CARTESIAN_POINT('Ctrl Pts',(18.5918548159157,9.24542108706308,5.8222239865161));
#58282=CARTESIAN_POINT('Ctrl Pts',(18.552166774966,10.2129933121371,4.28576426362096));
#58283=CARTESIAN_POINT('Ctrl Pts',(18.5124787340162,10.7892782664439,2.50289476533254));
#58284=CARTESIAN_POINT('Ctrl Pts',(18.4727906930665,10.9040778205241,0.690789483292698));
#58285=CARTESIAN_POINT('Ctrl Pts',(18.4331026521168,11.0188773746044,-1.12131579874729));
#58286=CARTESIAN_POINT('Ctrl Pts',(18.393414611167,10.672191528458,-2.96265686453859));
#58287=CARTESIAN_POINT('Ctrl Pts',(18.3537265702173,9.90625060187318,-4.60893721362761));
#58288=CARTESIAN_POINT('Ctrl Pts',(18.3140385292676,9.14030967528842,-6.25521756271648));
#58289=CARTESIAN_POINT('Ctrl Pts',(18.2743504883178,7.95511366826528,-7.70643719510299));
#58290=CARTESIAN_POINT('Ctrl Pts',(18.2346624473681,6.49503307341151,-8.78582088376293));
#58291=CARTESIAN_POINT('Ctrl Pts',(18.1949744064184,5.03495247855769,-9.86520457242291));
#58292=CARTESIAN_POINT('Ctrl Pts',(18.1552863654687,3.29998729587319,-10.5727523173563));
#58293=CARTESIAN_POINT('Ctrl Pts',(18.1155983245189,1.5014762208963,-10.8222766728797));
#58294=CARTESIAN_POINT('Ctrl Pts',(18.0759102835692,-0.297034854080688,
-11.0718010284032));
#58295=CARTESIAN_POINT('Ctrl Pts',(18.0362222426195,-2.1590918213501,-10.8633019945166));
#58296=CARTESIAN_POINT('Ctrl Pts',(17.9965342016697,-3.85787474561397,-10.2221771493859));
#58297=CARTESIAN_POINT('Ctrl Pts',(17.95684616072,-5.55665766987775,-9.58105230425535));
#58298=CARTESIAN_POINT('Ctrl Pts',(17.9171581197703,-7.09216655113603,-8.5073016478808));
#58299=CARTESIAN_POINT('Ctrl Pts',(17.8774700788205,-8.27735876329387,-7.13172034855521));
#58300=CARTESIAN_POINT('Ctrl Pts',(17.8377820378708,-9.46255097545171,-5.75613904922961));
#58301=CARTESIAN_POINT('Ctrl Pts',(17.7980939969211,-10.2974265185091,-4.07872710695295));
#58302=CARTESIAN_POINT('Ctrl Pts',(17.7584059559714,-10.680287957862,-2.3038125712441));
#58303=CARTESIAN_POINT('Ctrl Pts',(17.7414995791026,-10.8433799026218,-1.54773156214473));
#58304=CARTESIAN_POINT('Ctrl Pts',(17.7245932022339,-10.9244492055384,-0.773957697370454));
#58305=CARTESIAN_POINT('Ctrl Pts',(17.7076868253652,-10.9241469997933,-0.000121431705876017));
#58306=CARTESIAN_POINT('Ctrl Pts',(17.4923131746348,-10.9255250468596,0.000220564452133845));
#58307=CARTESIAN_POINT('Ctrl Pts',(17.5265430037136,-10.9241037915595,-1.56597446482467));
#58308=CARTESIAN_POINT('Ctrl Pts',(17.5607728327924,-10.5836727962495,-3.13276740070408));
#58309=CARTESIAN_POINT('Ctrl Pts',(17.5950026618713,-9.93063582780699,-4.55613790637411));
#58310=CARTESIAN_POINT('Ctrl Pts',(17.6346043405313,-9.17511466765573,-6.20288470285888));
#58311=CARTESIAN_POINT('Ctrl Pts',(17.6742060191914,-8.00117103460732,-7.65766086194424));
#58312=CARTESIAN_POINT('Ctrl Pts',(17.7138076978515,-6.55119597054485,-8.74401234685425));
#58313=CARTESIAN_POINT('Ctrl Pts',(17.7534093765116,-5.10122090648234,-9.83036383176429));
#58314=CARTESIAN_POINT('Ctrl Pts',(17.7930110551716,-3.37521441140574,-10.548290642499));
#58315=CARTESIAN_POINT('Ctrl Pts',(17.8326127338317,-1.5825288393908,-10.8107133455161));
#58316=CARTESIAN_POINT('Ctrl Pts',(17.8722144124918,0.21015673262414,-11.0731360485332));
#58317=CARTESIAN_POINT('Ctrl Pts',(17.9118160911519,2.06952138157742,-10.8800546438327));
#58318=CARTESIAN_POINT('Ctrl Pts',(17.951417769812,3.77003735455852,-10.2548885372614));
#58319=CARTESIAN_POINT('Ctrl Pts',(17.991019448472,5.47055332753962,-9.62972243069016));
#58320=CARTESIAN_POINT('Ctrl Pts',(18.0306211271321,7.01222062454853,-8.57247162224806));
#58321=CARTESIAN_POINT('Ctrl Pts',(18.0702228057922,8.20804592965566,-7.21137314130159));
#58322=CARTESIAN_POINT('Ctrl Pts',(18.1098244844523,9.40387123476282,-5.85027466035508));
#58323=CARTESIAN_POINT('Ctrl Pts',(18.1494261631123,10.2538545479682,-4.18532850690418));
#58324=CARTESIAN_POINT('Ctrl Pts',(18.1890278417724,10.6548989179843,-2.41848084837561));
#58325=CARTESIAN_POINT('Ctrl Pts',(18.2286295204325,11.0559432880004,-0.651633189847145));
#58326=CARTESIAN_POINT('Ctrl Pts',(18.2682311990926,11.0080487148274,1.21711597375898));
#58327=CARTESIAN_POINT('Ctrl Pts',(18.3078328777526,10.5170244707187,2.96110061442146));
#58328=CARTESIAN_POINT('Ctrl Pts',(18.3474345564127,10.02600022661,4.70508525508395));
#58329=CARTESIAN_POINT('Ctrl Pts',(18.3870362350728,9.09184631156565,6.32430537280278));
#58330=CARTESIAN_POINT('Ctrl Pts',(18.4266379137329,7.82786897428255,7.62236104418359));
#58331=CARTESIAN_POINT('Ctrl Pts',(18.466239592393,6.56389163699937,8.92041671556447));
#58332=CARTESIAN_POINT('Ctrl Pts',(18.505841271053,4.97009087747741,9.89730794060729));
#58333=CARTESIAN_POINT('Ctrl Pts',(18.5454429497131,3.23978343113185,10.4345447378305));
#58334=CARTESIAN_POINT('Ctrl Pts',(18.5850446283732,1.5094759847864,10.9717815350537));
#58335=CARTESIAN_POINT('Ctrl Pts',(18.6246463070332,-0.357338148382625,
11.0693639044573));
#58336=CARTESIAN_POINT('Ctrl Pts',(18.6642479856933,-2.13422764583061,10.7154557962877));
#58337=CARTESIAN_POINT('Ctrl Pts',(18.7038496643534,-3.91111714327869,10.361547688118));
#58338=CARTESIAN_POINT('Ctrl Pts',(18.7434513430135,-5.59808200500573,9.55614910237504));
#58339=CARTESIAN_POINT('Ctrl Pts',(18.7830530216736,-6.9905053503377,8.39694917891747));
#58340=CARTESIAN_POINT('Ctrl Pts',(18.8226547003336,-8.38292869566959,7.23774925545996));
#58341=CARTESIAN_POINT('Ctrl Pts',(18.8622563789937,-9.48081052460645,5.72474799428789));
#58342=CARTESIAN_POINT('Ctrl Pts',(18.9018580576538,-10.1509855529848,4.0414617243661));
#58343=CARTESIAN_POINT('Ctrl Pts',(18.9320097633141,-10.6612396856448,2.75985059397857));
#58344=CARTESIAN_POINT('Ctrl Pts',(18.9621614689745,-10.9235560233316,1.37952677178609));
#58345=CARTESIAN_POINT('Ctrl Pts',(18.9923131746348,-10.9249542541001,-0.00028052102294644));
#58346=CARTESIAN_POINT('Origin',(21.9,0.,0.));
#58347=CARTESIAN_POINT('',(20.7076868253652,-10.925006192269,-0.000282974249596251));
#58348=CARTESIAN_POINT('',(20.4923131746348,-10.92425950121,0.000175479587483748));
#58349=CARTESIAN_POINT('',(21.9,-10.925,-1.33792662806848E-15));
#58350=CARTESIAN_POINT('Ctrl Pts',(20.7076868253652,-10.925006192269,-0.000282974249596251));
#58351=CARTESIAN_POINT('Ctrl Pts',(20.6771061850275,-10.9235686517141,1.39913390215185));
#58352=CARTESIAN_POINT('Ctrl Pts',(20.6465255446897,-10.6535723682374,2.79908945206647));
#58353=CARTESIAN_POINT('Ctrl Pts',(20.615944904352,-10.1290618526216,4.0961212399098));
#58354=CARTESIAN_POINT('Ctrl Pts',(20.5762568634022,-9.44834377110301,5.77942970371189));
#58355=CARTESIAN_POINT('Ctrl Pts',(20.5365688224525,-8.33894072970833,7.28938099042024));
#58356=CARTESIAN_POINT('Ctrl Pts',(20.4968807815027,-6.93599076690339,8.44204568263552));
#58357=CARTESIAN_POINT('Ctrl Pts',(20.457192740553,-5.5330408040985,9.59471037485078));
#58358=CARTESIAN_POINT('Ctrl Pts',(20.4175046996033,-3.8365439198834,10.390088472573));
#58359=CARTESIAN_POINT('Ctrl Pts',(20.3778166586536,-2.05315292900791,10.7312937839004));
#58360=CARTESIAN_POINT('Ctrl Pts',(20.3381286177038,-0.269761938132422,
11.0724990952279));
#58361=CARTESIAN_POINT('Ctrl Pts',(20.2984405767541,1.60052315940342,10.9595316201607));
#58362=CARTESIAN_POINT('Ctrl Pts',(20.2587525358044,3.32988014748677,10.4061520952583));
#58363=CARTESIAN_POINT('Ctrl Pts',(20.2190644948546,5.05923713557017,9.85277257035582));
#58364=CARTESIAN_POINT('Ctrl Pts',(20.1793764539049,6.64766601420104,8.85898099561823));
#58365=CARTESIAN_POINT('Ctrl Pts',(20.1396884129552,7.90167789350684,7.54583260439427));
#58366=CARTESIAN_POINT('Ctrl Pts',(20.1000003720054,9.1556897728126,6.23268421317035));
#58367=CARTESIAN_POINT('Ctrl Pts',(20.0603123310557,10.0752846527933,4.60017900546012));
#58368=CARTESIAN_POINT('Ctrl Pts',(20.020624290106,10.5484453101073,2.84717487449404));
#58369=CARTESIAN_POINT('Ctrl Pts',(19.9809362491563,11.0216059674212,1.094170743528));
#58370=CARTESIAN_POINT('Ctrl Pts',(19.9412482082065,11.0483324020685,-0.779332310693993));
#58371=CARTESIAN_POINT('Ctrl Pts',(19.9015601672568,10.6253690271986,-2.54512008795728));
#58372=CARTESIAN_POINT('Ctrl Pts',(19.8618721263071,10.2024056523286,-4.31090786522066));
#58373=CARTESIAN_POINT('Ctrl Pts',(19.8221840853573,9.32975246794149,-5.96898036552543));
#58374=CARTESIAN_POINT('Ctrl Pts',(19.7824960444076,8.11370865945383,-7.31736530561227));
#58375=CARTESIAN_POINT('Ctrl Pts',(19.7428080034579,6.89766485096618,-8.6657502456991));
#58376=CARTESIAN_POINT('Ctrl Pts',(19.7031199625081,5.33823041837804,-9.70444762556797));
#58377=CARTESIAN_POINT('Ctrl Pts',(19.6634319215584,3.62536239486206,-10.3069321687976));
#58378=CARTESIAN_POINT('Ctrl Pts',(19.6237438806087,1.91249437134617,-10.9094167120271));
#58379=CARTESIAN_POINT('Ctrl Pts',(19.584055839659,0.0461927569025075,-11.0756884186175));
#58380=CARTESIAN_POINT('Ctrl Pts',(19.5443677987092,-1.74620546637049,-10.7854934840967));
#58381=CARTESIAN_POINT('Ctrl Pts',(19.5046797577595,-3.5386036896436,-10.4952985495759));
#58382=CARTESIAN_POINT('Ctrl Pts',(19.4649917168098,-5.25709852174599,-9.74863697394382));
#58383=CARTESIAN_POINT('Ctrl Pts',(19.42530367586,-6.69235754509926,-8.63646071691566));
#58384=CARTESIAN_POINT('Ctrl Pts',(19.3856156349103,-8.12761656845248,-7.52428445988753));
#58385=CARTESIAN_POINT('Ctrl Pts',(19.3459275939606,-9.27963978305655,-6.04659352146332));
#58386=CARTESIAN_POINT('Ctrl Pts',(19.3062395530108,-10.0080975236052,-4.38338763792133));
#58387=CARTESIAN_POINT('Ctrl Pts',(19.2733886437956,-10.6110625107708,-3.00670528779863));
#58388=CARTESIAN_POINT('Ctrl Pts',(19.2405377345804,-10.9238284280163,-1.50292035772768));
#58389=CARTESIAN_POINT('Ctrl Pts',(19.2076868253652,-10.9253333599821,0.000257774600414338));
#58390=CARTESIAN_POINT('Ctrl Pts',(18.9923131746348,-10.9249542541001,-0.00028052102294644));
#58391=CARTESIAN_POINT('Ctrl Pts',(19.0017631476345,-10.9253924794913,-0.432731733195183));
#58392=CARTESIAN_POINT('Ctrl Pts',(19.0112131206343,-10.9002011192736,-0.865132207478021));
#58393=CARTESIAN_POINT('Ctrl Pts',(19.020663093634,-10.8489805590025,-1.29442705349038));
#58394=CARTESIAN_POINT('Ctrl Pts',(19.0602647722941,-10.634332308822,-3.09345828275344));
#58395=CARTESIAN_POINT('Ctrl Pts',(19.0998664509542,-9.96256758064119,-4.83794946260802));
#58396=CARTESIAN_POINT('Ctrl Pts',(19.1394681296142,-8.91516667458106,-6.31630617773253));
#58397=CARTESIAN_POINT('Ctrl Pts',(19.1790698082743,-7.86776576852089,-7.79466289285708));
#58398=CARTESIAN_POINT('Ctrl Pts',(19.2186714869344,-6.44472868458153,-9.00688514325149));
#58399=CARTESIAN_POINT('Ctrl Pts',(19.2582731655945,-4.8186597346872,-9.80593896206412));
#58400=CARTESIAN_POINT('Ctrl Pts',(19.2978748442545,-3.19259078479291,-10.6049927808767));
#58401=CARTESIAN_POINT('Ctrl Pts',(19.3374765229146,-1.36348996894375,-10.9908781681075));
#58402=CARTESIAN_POINT('Ctrl Pts',(19.3770782015747,0.446785748397966,-10.9167899614058));
#58403=CARTESIAN_POINT('Ctrl Pts',(19.4166798802348,2.25706146573963,-10.8427017547042));
#58404=CARTESIAN_POINT('Ctrl Pts',(19.4562815588948,4.04851208457388,-10.3086399540701));
#58405=CARTESIAN_POINT('Ctrl Pts',(19.4958832375549,5.60384734247514,-9.37938247053915));
#58406=CARTESIAN_POINT('Ctrl Pts',(19.535484916215,7.15918260037649,-8.45012498700811));
#58407=CARTESIAN_POINT('Ctrl Pts',(19.5750865948751,8.47840249734486,-7.12567182058006));
#58408=CARTESIAN_POINT('Ctrl Pts',(19.6146882735351,9.40149501038858,-5.56666975273918));
#58409=CARTESIAN_POINT('Ctrl Pts',(19.6542899521952,10.3245875234323,-4.00766768489835));
#58410=CARTESIAN_POINT('Ctrl Pts',(19.6938916308553,10.8515526525514,-2.21411671564468));
#58411=CARTESIAN_POINT('Ctrl Pts',(19.7334933095154,10.9184732626646,-0.403561865022531));
#58412=CARTESIAN_POINT('Ctrl Pts',(19.7730949881754,10.9853938727779,1.40699298559962));
#58413=CARTESIAN_POINT('Ctrl Pts',(19.8126966668355,10.5922699638853,3.23455171759028));
#58414=CARTESIAN_POINT('Ctrl Pts',(19.8522983454956,9.78678467970898,4.857444410329));
#58415=CARTESIAN_POINT('Ctrl Pts',(19.8919000241557,8.98129939553267,6.48033710306778));
#58416=CARTESIAN_POINT('Ctrl Pts',(19.9315017028158,7.76345273607263,7.89856375655464));
#58417=CARTESIAN_POINT('Ctrl Pts',(19.9711033814758,6.28096086913506,8.94010352998313));
#58418=CARTESIAN_POINT('Ctrl Pts',(20.0107050601359,4.79846900219757,9.98164330341156));
#58419=CARTESIAN_POINT('Ctrl Pts',(20.050306738796,3.05133192778256,10.6464961967817));
#58420=CARTESIAN_POINT('Ctrl Pts',(20.0899084174561,1.25146498946789,10.8540202665445));
#58421=CARTESIAN_POINT('Ctrl Pts',(20.1295100961161,-0.548401948846876,
11.0615443363074));
#58422=CARTESIAN_POINT('Ctrl Pts',(20.1691117747762,-2.40099875106118,10.8117395824629));
#58423=CARTESIAN_POINT('Ctrl Pts',(20.2087134534363,-4.08161855610429,10.1349055510591));
#58424=CARTESIAN_POINT('Ctrl Pts',(20.2483151320964,-5.76223836114735,9.45807151965526));
#58425=CARTESIAN_POINT('Ctrl Pts',(20.2879168107564,-7.27088116901912,8.3542082106921));
#58426=CARTESIAN_POINT('Ctrl Pts',(20.3275184894165,-8.42455930024771,6.95720641946411));
#58427=CARTESIAN_POINT('Ctrl Pts',(20.3671201680766,-9.5782374314763,5.56020462823612));
#58428=CARTESIAN_POINT('Ctrl Pts',(20.4067218467367,-10.3769508860618,3.87006435474326));
#58429=CARTESIAN_POINT('Ctrl Pts',(20.4463235253967,-10.7238213831711,2.09178763459974));
#58430=CARTESIAN_POINT('Ctrl Pts',(20.4616534084761,-10.8580955943734,1.40341342610875));
#58431=CARTESIAN_POINT('Ctrl Pts',(20.4769832915555,-10.9246621132901,0.701832161249542));
#58432=CARTESIAN_POINT('Ctrl Pts',(20.4923131746348,-10.92425950121,0.000175479587483748));
#58433=CARTESIAN_POINT('Origin',(21.9,0.,0.));
#58434=CARTESIAN_POINT('',(22.2076868253652,-10.9243163058926,0.000200730939527199));
#58435=CARTESIAN_POINT('',(21.9923131746348,-10.9259241478433,2.44403535691233E-5));
#58436=CARTESIAN_POINT('',(21.9,-10.925,-1.33792662806848E-15));
#58437=CARTESIAN_POINT('Ctrl Pts',(22.2076868253652,-10.9243163058926,0.000200730939527199));
#58438=CARTESIAN_POINT('Ctrl Pts',(22.193050717374,-10.9247574703059,0.670092849737773));
#58439=CARTESIAN_POINT('Ctrl Pts',(22.1784146093827,-10.8641210749225,1.33990606260495));
#58440=CARTESIAN_POINT('Ctrl Pts',(22.1637785013914,-10.7416585226029,1.99821805868802));
#58441=CARTESIAN_POINT('Ctrl Pts',(22.1240904604417,-10.409582618669,3.78333152422476));
#58442=CARTESIAN_POINT('Ctrl Pts',(22.084402419492,-9.62289526899957,5.48387585189108));
#58443=CARTESIAN_POINT('Ctrl Pts',(22.0447143785423,-8.47742403251909,6.89270520181605));
#58444=CARTESIAN_POINT('Ctrl Pts',(22.0050263375925,-7.33195279603862,8.30153455174101));
#58445=CARTESIAN_POINT('Ctrl Pts',(21.9653382966428,-5.8276976727471,9.41864892392462));
#58446=CARTESIAN_POINT('Ctrl Pts',(21.9256502556931,-4.14789422188571,10.1079709512009));
#58447=CARTESIAN_POINT('Ctrl Pts',(21.8859622147433,-2.46809077102438,10.7972929784772));
#58448=CARTESIAN_POINT('Ctrl Pts',(21.8462741737936,-0.612738992593189,
11.0588226608461));
#58449=CARTESIAN_POINT('Ctrl Pts',(21.8065861328439,1.19215794715898,10.8607026777875));
#58450=CARTESIAN_POINT('Ctrl Pts',(21.7668980918941,2.99705488691115,10.6625826947288));
#58451=CARTESIAN_POINT('Ctrl Pts',(21.7272100509444,4.75149698798431,10.0048130462425));
#58452=CARTESIAN_POINT('Ctrl Pts',(21.6875220099947,6.2417730423734,8.96751763387031));
#58453=CARTESIAN_POINT('Ctrl Pts',(21.647833969045,7.73204909676249,7.93022222149811));
#58454=CARTESIAN_POINT('Ctrl Pts',(21.6081459280952,8.95815910446752,6.51340104524003));
#58455=CARTESIAN_POINT('Ctrl Pts',(21.5684578871455,9.77074877745958,4.88963920489503));
#58456=CARTESIAN_POINT('Ctrl Pts',(21.5287698461958,10.5833384504516,3.26587736455003));
#58457=CARTESIAN_POINT('Ctrl Pts',(21.489081805246,10.9824077887307,1.43517486011812));
#58458=CARTESIAN_POINT('Ctrl Pts',(21.4493937642963,10.9193455612341,-0.37946770696695));
#58459=CARTESIAN_POINT('Ctrl Pts',(21.4097057233466,10.8562833337375,-2.19411027405207));
#58460=CARTESIAN_POINT('Ctrl Pts',(21.3700176823968,10.3310895404653,-3.99269290379035));
#58461=CARTESIAN_POINT('Ctrl Pts',(21.3303296414471,9.40773882037989,-5.55612756457152));
#58462=CARTESIAN_POINT('Ctrl Pts',(21.2906416004974,8.48438810029453,-7.1195622253527));
#58463=CARTESIAN_POINT('Ctrl Pts',(21.2509535595476,7.16288045339608,-8.44784891717677));
#58464=CARTESIAN_POINT('Ctrl Pts',(21.2112655185979,5.60419069637065,-9.37918705778848));
#58465=CARTESIAN_POINT('Ctrl Pts',(21.1715774776482,4.04550093934525,-10.3105251984002));
#58466=CARTESIAN_POINT('Ctrl Pts',(21.1318894366984,2.24962907219287,-10.8449147877995));
#58467=CARTESIAN_POINT('Ctrl Pts',(21.0922013957487,0.435332924491733,-10.9172610333878));
#58468=CARTESIAN_POINT('Ctrl Pts',(21.052513354799,-1.37896322320941,-10.9896072789761));
#58469=CARTESIAN_POINT('Ctrl Pts',(21.0128253138493,-3.21168365145931,-10.5999101807533));
#58470=CARTESIAN_POINT('Ctrl Pts',(20.9731372728995,-4.83958195251546,-9.79563932324792));
#58471=CARTESIAN_POINT('Ctrl Pts',(20.9334492319498,-6.46748025357165,-8.99136846574253));
#58472=CARTESIAN_POINT('Ctrl Pts',(20.8937611910001,-7.89055642743409,-7.77252384895453));
#58473=CARTESIAN_POINT('Ctrl Pts',(20.8540731500503,-8.93546344372008,-6.28757475281339));
#58474=CARTESIAN_POINT('Ctrl Pts',(20.8143851091006,-9.98037046000605,-4.80262565667228));
#58475=CARTESIAN_POINT('Ctrl Pts',(20.7746970681509,-10.6471083187156,-3.05157208117804));
#58476=CARTESIAN_POINT('Ctrl Pts',(20.7350090272011,-10.8544606872491,-1.24771247298303));
#58477=CARTESIAN_POINT('Ctrl Pts',(20.7259016265892,-10.9020428062675,-0.833772361391162));
#58478=CARTESIAN_POINT('Ctrl Pts',(20.7167942259772,-10.9254343146885,-0.417051556456601));
#58479=CARTESIAN_POINT('Ctrl Pts',(20.7076868253652,-10.925006192269,-0.000282974249596251));
#58480=CARTESIAN_POINT('Ctrl Pts',(20.4923131746348,-10.92425950121,0.000175479587483748));
#58481=CARTESIAN_POINT('Ctrl Pts',(20.5165849702155,-10.9236220457217,-1.11075716464629));
#58482=CARTESIAN_POINT('Ctrl Pts',(20.5408567657962,-10.7551038830222,-2.22187886652514));
#58483=CARTESIAN_POINT('Ctrl Pts',(20.565128561377,-10.4216364174784,-3.28106917761739));
#58484=CARTESIAN_POINT('Ctrl Pts',(20.604730240037,-9.8775534150429,-5.00923610289699));
#58485=CARTESIAN_POINT('Ctrl Pts',(20.6443319186971,-8.89435987053856,-6.59915678666188));
#58486=CARTESIAN_POINT('Ctrl Pts',(20.6839335973572,-7.59131019212733,-7.8579851191846));
#58487=CARTESIAN_POINT('Ctrl Pts',(20.7235352760173,-6.28826051371616,-9.11681345170724));
#58488=CARTESIAN_POINT('Ctrl Pts',(20.7631369546773,-4.66535470139817,-10.0445494329877));
#58489=CARTESIAN_POINT('Ctrl Pts',(20.8027386333374,-2.91943972719868,-10.528665264205));
#58490=CARTESIAN_POINT('Ctrl Pts',(20.8423403119975,-1.17352475299909,-11.0127810954223));
#58491=CARTESIAN_POINT('Ctrl Pts',(20.8819419906576,0.695399383082116,-11.0532767765763));
#58492=CARTESIAN_POINT('Ctrl Pts',(20.9215436693177,2.4606454301023,-10.6452404685728));
#58493=CARTESIAN_POINT('Ctrl Pts',(20.9611453479777,4.22589147712238,-10.2372041605693));
#58494=CARTESIAN_POINT('Ctrl Pts',(21.0007470266378,5.88745943508158,-9.38063586340824));
#58495=CARTESIAN_POINT('Ctrl Pts',(21.0403487052979,7.24381288772203,-8.17943124025717));
#58496=CARTESIAN_POINT('Ctrl Pts',(21.079950383958,8.60016634036252,-6.97822661710607));
#58497=CARTESIAN_POINT('Ctrl Pts',(21.119552062618,9.65130528768423,-5.43238566796492));
#58498=CARTESIAN_POINT('Ctrl Pts',(21.1591537412781,10.2697340257543,-3.72940794318446));
#58499=CARTESIAN_POINT('Ctrl Pts',(21.1987554199382,10.8881627638244,-2.026430218404));
#58500=CARTESIAN_POINT('Ctrl Pts',(21.2383570985983,11.0738812926428,-0.166315717984266));
#58501=CARTESIAN_POINT('Ctrl Pts',(21.2779587772583,10.8043632710199,1.62531685349624));
#58502=CARTESIAN_POINT('Ctrl Pts',(21.3175604559184,10.534845249397,3.4169494249767));
#58503=CARTESIAN_POINT('Ctrl Pts',(21.3571621345785,9.81009067733293,5.1401000675179));
#58504=CARTESIAN_POINT('Ctrl Pts',(21.3967638132386,8.71800714742444,6.58576282171467));
#58505=CARTESIAN_POINT('Ctrl Pts',(21.4363654918986,7.62592361751589,8.03142557591153));
#58506=CARTESIAN_POINT('Ctrl Pts',(21.4759671705587,6.16651112976293,9.19960044176388));
#58507=CARTESIAN_POINT('Ctrl Pts',(21.5155688492188,4.51678607474703,9.94859608796106));
#58508=CARTESIAN_POINT('Ctrl Pts',(21.5551705278789,2.86706101973122,10.6975917341582));
#58509=CARTESIAN_POINT('Ctrl Pts',(21.5947722065389,1.02702339745236,11.0274081607002));
#58510=CARTESIAN_POINT('Ctrl Pts',(21.634373885199,-0.780143270526186,10.8980409727563));
#58511=CARTESIAN_POINT('Ctrl Pts',(21.6739755638591,-2.58730993850478,10.7686737848124));
#58512=CARTESIAN_POINT('Ctrl Pts',(21.7135772425192,-4.36160565218317,10.1801229823827));
#58513=CARTESIAN_POINT('Ctrl Pts',(21.7531789211792,-5.88782091753883,9.20377560620721));
#58514=CARTESIAN_POINT('Ctrl Pts',(21.7927805998393,-7.41403618289454,8.22742823003172));
#58515=CARTESIAN_POINT('Ctrl Pts',(21.8323822784994,-8.69217099992747,6.86328428011052));
#58516=CARTESIAN_POINT('Ctrl Pts',(21.8719839571595,-9.56719667463488,5.2768047486408));
#58517=CARTESIAN_POINT('Ctrl Pts',(21.9115856358196,-10.4422223493422,3.69032521717116));
#58518=CARTESIAN_POINT('Ctrl Pts',(21.9511873144796,-10.9141388817241,1.88151010415307));
#58519=CARTESIAN_POINT('Ctrl Pts',(21.9907889931397,-10.925706141304,0.0697558620785545));
#58520=CARTESIAN_POINT('Ctrl Pts',(21.9912970536381,-10.9258545407625,0.0465123836628863));
#58521=CARTESIAN_POINT('Ctrl Pts',(21.9918051141364,-10.9259271712951,0.0232684214957185));
#58522=CARTESIAN_POINT('Ctrl Pts',(21.9923131746348,-10.9259241478433,2.44403535691233E-5));
#58523=CARTESIAN_POINT('Origin',(21.9,0.,0.));
#58524=CARTESIAN_POINT('',(23.7076868253652,-10.9259072644299,-6.29504943074994E-5));
#58525=CARTESIAN_POINT('',(23.4923131746348,-10.9243498732306,-0.000207109954374048));
#58526=CARTESIAN_POINT('',(21.9,-10.925,-1.33792662806848E-15));
#58527=CARTESIAN_POINT('Ctrl Pts',(23.7076868253652,-10.9259072644299,-6.29504943074994E-5));
#58528=CARTESIAN_POINT('Ctrl Pts',(23.6693072087707,-10.9253516253319,1.75582831417521));
#58529=CARTESIAN_POINT('Ctrl Pts',(23.6309275921762,-10.494054765262,3.51198273621341));
#58530=CARTESIAN_POINT('Ctrl Pts',(23.5925479755817,-9.67965890632121,5.06757404322333));
#58531=CARTESIAN_POINT('Ctrl Pts',(23.552859934632,-8.83749895093565,6.67619802052782));
#58532=CARTESIAN_POINT('Ctrl Pts',(23.5131718936823,-7.58567379158093,8.07035072625783));
#58533=CARTESIAN_POINT('Ctrl Pts',(23.4734838527325,-6.07667011724678,9.08020834080552));
#58534=CARTESIAN_POINT('Ctrl Pts',(23.4337958117828,-4.56766644291259,10.0900659553532));
#58535=CARTESIAN_POINT('Ctrl Pts',(23.3941077708331,-2.80148425359894,10.7156284787186));
#58536=CARTESIAN_POINT('Ctrl Pts',(23.3544197298834,-0.993264834962619,
10.880695207288));
#58537=CARTESIAN_POINT('Ctrl Pts',(23.3147316889336,0.814954583673604,11.0457619358575));
#58538=CARTESIAN_POINT('Ctrl Pts',(23.2750436479839,2.66521123163251,10.750332869631));
#58539=CARTESIAN_POINT('Ctrl Pts',(23.2353556070342,4.33212258810432,10.0303946636167));
#58540=CARTESIAN_POINT('Ctrl Pts',(23.1956675660844,5.99903394457623,9.31045645760242));
#58541=CARTESIAN_POINT('Ctrl Pts',(23.1559795251347,7.48260000956104,8.1660091118003));
#58542=CARTESIAN_POINT('Ctrl Pts',(23.116291484185,8.60210538885491,6.73645946364317));
#58543=CARTESIAN_POINT('Ctrl Pts',(23.0766034432352,9.72161076814875,5.30690981548607));
#58544=CARTESIAN_POINT('Ctrl Pts',(23.0369154022855,10.4770554617517,3.59225786497398));
#58545=CARTESIAN_POINT('Ctrl Pts',(22.9972273613358,10.7764176252539,1.8013679225495));
#58546=CARTESIAN_POINT('Ctrl Pts',(22.957539320386,11.0757797887562,0.0104779801250157));
#58547=CARTESIAN_POINT('Ctrl Pts',(22.9178512794363,10.9190594221578,-1.85664995421185));
#58548=CARTESIAN_POINT('Ctrl Pts',(22.8781632384866,10.3253468669663,-3.57257824310445));
#58549=CARTESIAN_POINT('Ctrl Pts',(22.8384751975369,9.73163431177479,-5.2885065319971));
#58550=CARTESIAN_POINT('Ctrl Pts',(22.7987871565872,8.70092956799014,-6.85323517544548));
#58551=CARTESIAN_POINT('Ctrl Pts',(22.7590991156374,7.35878431711615,-8.07616224455897));
#58552=CARTESIAN_POINT('Ctrl Pts',(22.7194110746877,6.01663906624216,-9.29908931367245));
#58553=CARTESIAN_POINT('Ctrl Pts',(22.6797230337379,4.36305330827881,-10.180214808451));
#58554=CARTESIAN_POINT('Ctrl Pts',(22.6400349927882,2.59945278971167,-10.612207518718));
#58555=CARTESIAN_POINT('Ctrl Pts',(22.6003469518385,0.835852271144566,-11.0442002289849));
#58556=CARTESIAN_POINT('Ctrl Pts',(22.5606589108888,-1.03776300802633,-11.0270601547403));
#58557=CARTESIAN_POINT('Ctrl Pts',(22.520970869939,-2.79316517729827,-10.5628751539816));
#58558=CARTESIAN_POINT('Ctrl Pts',(22.4812828289893,-4.54856734657022,-10.098690153223));
#58559=CARTESIAN_POINT('Ctrl Pts',(22.4415947880396,-6.1857564059432,-9.18746022595042));
#58560=CARTESIAN_POINT('Ctrl Pts',(22.4019067470898,-7.50530391523259,-7.94018364814497));
#58561=CARTESIAN_POINT('Ctrl Pts',(22.3622187061401,-8.82485142452198,-6.69290707033951));
#58562=CARTESIAN_POINT('Ctrl Pts',(22.3225306651904,-9.82675738372778,-5.10958384200119));
#58563=CARTESIAN_POINT('Ctrl Pts',(22.2828426242406,-10.3889781342315,-3.38308092612848));
#58564=CARTESIAN_POINT('Ctrl Pts',(22.2577906912822,-10.7438637927935,-2.29327567835032));
#58565=CARTESIAN_POINT('Ctrl Pts',(22.2327387583237,-10.9235611856575,-1.14642188619113));
#58566=CARTESIAN_POINT('Ctrl Pts',(22.2076868253652,-10.9243163058926,0.000200730939527199));
#58567=CARTESIAN_POINT('Ctrl Pts',(21.9923131746348,-10.9259241478433,2.44403535691233E-5));
#58568=CARTESIAN_POINT('Ctrl Pts',(22.0314067927965,-10.9256915029675,-1.78852500648809));
#58569=CARTESIAN_POINT('Ctrl Pts',(22.0705004109582,-10.4775262491999,-3.57718680052355));
#58570=CARTESIAN_POINT('Ctrl Pts',(22.1095940291199,-9.6337941789156,-5.15421480777767));
#58571=CARTESIAN_POINT('Ctrl Pts',(22.14919570778,-8.77909697016932,-6.75173786442839));
#58572=CARTESIAN_POINT('Ctrl Pts',(22.1887973864401,-7.5184845658988,-8.13209060659888));
#58573=CARTESIAN_POINT('Ctrl Pts',(22.2283990651001,-6.00486031563601,-9.12784603047853));
#58574=CARTESIAN_POINT('Ctrl Pts',(22.2680007437602,-4.49123606537322,-10.1236014543582));
#58575=CARTESIAN_POINT('Ctrl Pts',(22.3076024224203,-2.72459996911815,-10.734759559947));
#58576=CARTESIAN_POINT('Ctrl Pts',(22.3472041010804,-0.919232463590588,
-10.8871912008701));
#58577=CARTESIAN_POINT('Ctrl Pts',(22.3868057797405,0.886135041936973,-11.0396228417933));
#58578=CARTESIAN_POINT('Ctrl Pts',(22.4264074584005,2.73023395673704,-10.7333280180507));
#58579=CARTESIAN_POINT('Ctrl Pts',(22.4660091370606,4.38938815324973,-10.0054581207726));
#58580=CARTESIAN_POINT('Ctrl Pts',(22.5056108157207,6.04854234976241,-9.27758822349444));
#58581=CARTESIAN_POINT('Ctrl Pts',(22.5452124943808,7.52275182798774,-8.12814325268073));
#58582=CARTESIAN_POINT('Ctrl Pts',(22.5848141730408,8.63320542727963,-6.69654273612976));
#58583=CARTESIAN_POINT('Ctrl Pts',(22.6244158517009,9.74365902657153,-5.2649422195788));
#58584=CARTESIAN_POINT('Ctrl Pts',(22.664017530361,10.49035674693,-3.55118615729054));
#58585=CARTESIAN_POINT('Ctrl Pts',(22.7036192090211,10.7827294474011,-1.76314101267351));
#58586=CARTESIAN_POINT('Ctrl Pts',(22.7432208876811,11.0751021478722,0.0249041319435206));
#58587=CARTESIAN_POINT('Ctrl Pts',(22.7828225663412,10.913149828456,1.88723835888937));
#58588=CARTESIAN_POINT('Ctrl Pts',(22.8224242450013,10.3165161575942,3.59797372649108));
#58589=CARTESIAN_POINT('Ctrl Pts',(22.8620259236614,9.71988248673245,5.30870909409284));
#58590=CARTESIAN_POINT('Ctrl Pts',(22.9016276023214,8.68856746442526,6.86784560235035));
#58591=CARTESIAN_POINT('Ctrl Pts',(22.9412292809815,7.34766229301129,8.08627104382996));
#58592=CARTESIAN_POINT('Ctrl Pts',(22.9808309596416,6.00675712159735,9.30469648530953));
#58593=CARTESIAN_POINT('Ctrl Pts',(23.0204326383017,4.35626180107671,10.1824108600111));
#58594=CARTESIAN_POINT('Ctrl Pts',(23.0600343169617,2.59636971526783,10.612953635443));
#58595=CARTESIAN_POINT('Ctrl Pts',(23.0996359956218,0.836477629458958,11.0434964108749));
#58596=CARTESIAN_POINT('Ctrl Pts',(23.1392376742819,-1.03281122163818,11.0268675870371));
#58597=CARTESIAN_POINT('Ctrl Pts',(23.178839352942,-2.78476534973483,10.5650841223977));
#58598=CARTESIAN_POINT('Ctrl Pts',(23.218441031602,-4.53671947783147,10.1033006577582));
#58599=CARTESIAN_POINT('Ctrl Pts',(23.2580427102621,-6.17133888292765,9.19636255231694));
#58600=CARTESIAN_POINT('Ctrl Pts',(23.2976443889222,-7.49035581721883,7.95427496996922));
#58601=CARTESIAN_POINT('Ctrl Pts',(23.3372460675823,-8.80937275151001,6.71218738762149));
#58602=CARTESIAN_POINT('Ctrl Pts',(23.3768477462423,-9.81278721499622,5.13495032836725));
#58603=CARTESIAN_POINT('Ctrl Pts',(23.4164494249024,-10.378892145367,3.41387146818122));
#58604=CARTESIAN_POINT('Ctrl Pts',(23.4417373414799,-10.7403822320925,2.31486505955907));
#58605=CARTESIAN_POINT('Ctrl Pts',(23.4670252580573,-10.9235573285534,1.15720648950317));
#58606=CARTESIAN_POINT('Ctrl Pts',(23.4923131746348,-10.9243498732306,-0.000207109954374048));
#58607=CARTESIAN_POINT('Origin',(21.9,0.,0.));
#58608=CARTESIAN_POINT('',(25.2076868253652,-10.9241289668202,-0.000107867347247034));
#58609=CARTESIAN_POINT('',(24.9923131746348,-10.9248114762173,0.000277509097762489));
#58610=CARTESIAN_POINT('',(21.9,-10.925,-1.33792662806848E-15));
#58611=CARTESIAN_POINT('Ctrl Pts',(25.2076868253652,-10.9241289668202,-0.000107867347247034));
#58612=CARTESIAN_POINT('Ctrl Pts',(25.1852517411172,-10.9237734560773,1.02679245281844));
#58613=CARTESIAN_POINT('Ctrl Pts',(25.1628166568692,-10.7801469522487,2.05379018050121));
#58614=CARTESIAN_POINT('Ctrl Pts',(25.1403815726212,-10.4945916088821,3.03967929049346));
#58615=CARTESIAN_POINT('Ctrl Pts',(25.1006935316715,-9.98943940906542,4.78373368925349));
#58616=CARTESIAN_POINT('Ctrl Pts',(25.0610054907218,-9.04013219783419,6.39914193957047));
#58617=CARTESIAN_POINT('Ctrl Pts',(25.0213174497721,-7.76230650189744,7.68912875408358));
#58618=CARTESIAN_POINT('Ctrl Pts',(24.9816294088223,-6.48448080596066,8.97911556859673));
#58619=CARTESIAN_POINT('Ctrl Pts',(24.9419413678726,-4.87813662531833,9.943680947306));
#58620=CARTESIAN_POINT('Ctrl Pts',(24.9022533269229,-3.13894513949073,10.4653297433737));
#58621=CARTESIAN_POINT('Ctrl Pts',(24.8625652859731,-1.39975365366312,10.9869785394414));
#58622=CARTESIAN_POINT('Ctrl Pts',(24.8228772450234,0.47228513734978,11.0657107528675));
#58623=CARTESIAN_POINT('Ctrl Pts',(24.7831892040736,2.24913539741806,10.6919358953538));
#58624=CARTESIAN_POINT('Ctrl Pts',(24.7435011631239,4.02598565748635,10.3181610378401));
#58625=CARTESIAN_POINT('Ctrl Pts',(24.7038131221742,5.70764738661004,9.49187910938671));
#58626=CARTESIAN_POINT('Ctrl Pts',(24.6641250812245,7.08927486239847,8.31374074359067));
#58627=CARTESIAN_POINT('Ctrl Pts',(24.6244370402747,8.47090233818682,7.13560237779469));
#58628=CARTESIAN_POINT('Ctrl Pts',(24.584748999325,9.55249556063996,5.60560757465611));
#58629=CARTESIAN_POINT('Ctrl Pts',(24.5450609583753,10.2023040467986,3.91012728219324));
#58630=CARTESIAN_POINT('Ctrl Pts',(24.5053729174255,10.8521125329572,2.21464698973033));
#58631=CARTESIAN_POINT('Ctrl Pts',(24.4656848764758,11.0701362828213,0.353681207943237));
#58632=CARTESIAN_POINT('Ctrl Pts',(24.4259968355261,10.8298174983713,-1.44608304680081));
#58633=CARTESIAN_POINT('Ctrl Pts',(24.3863087945764,10.5894987139214,-3.2458473015449));
#58634=CARTESIAN_POINT('Ctrl Pts',(24.3466207536266,9.89083739515729,-4.98441002924584));
#58635=CARTESIAN_POINT('Ctrl Pts',(24.3069327126769,8.81893851894224,-6.44999431204332));
#58636=CARTESIAN_POINT('Ctrl Pts',(24.2672446717272,7.74703964272719,-7.91557859484079));
#58637=CARTESIAN_POINT('Ctrl Pts',(24.2275566307774,6.30190320906113,-9.10818443273484));
#58638=CARTESIAN_POINT('Ctrl Pts',(24.1878685898277,4.65956344146277,-9.88253873057211));
#58639=CARTESIAN_POINT('Ctrl Pts',(24.148180548878,3.01722367386441,-10.6568930284094));
#58640=CARTESIAN_POINT('Ctrl Pts',(24.1084925079282,1.17768057233372,-11.0129957861899));
#58641=CARTESIAN_POINT('Ctrl Pts',(24.0688044669785,-0.634988375382582,
-10.9074695960797));
#58642=CARTESIAN_POINT('Ctrl Pts',(24.0291164260288,-2.44765732309878,-10.8019434059696));
#58643=CARTESIAN_POINT('Ctrl Pts',(23.9894283850791,-4.23345211700061,-10.2347882679688));
#58644=CARTESIAN_POINT('Ctrl Pts',(23.9497403441293,-5.77484243082628,-9.27509019500095));
#58645=CARTESIAN_POINT('Ctrl Pts',(23.9100523031796,-7.31623274465203,-8.31539212203307));
#58646=CARTESIAN_POINT('Ctrl Pts',(23.8703642622299,-8.61321857840161,-6.96315111409812));
#58647=CARTESIAN_POINT('Ctrl Pts',(23.8306762212801,-9.50781215400779,-5.38308566440996));
#58648=CARTESIAN_POINT('Ctrl Pts',(23.7909881803304,-10.402405729614,-3.80302021472186));
#58649=CARTESIAN_POINT('Ctrl Pts',(23.7513001393807,-10.8946070470768,-1.99513032328054));
#58650=CARTESIAN_POINT('Ctrl Pts',(23.7116120984309,-10.9244603301,-0.179637753120411));
#58651=CARTESIAN_POINT('Ctrl Pts',(23.7103036740757,-10.9254445248765,-0.119785096282008));
#58652=CARTESIAN_POINT('Ctrl Pts',(23.7089952497205,-10.9259262070821,-0.0599241763142232));
#58653=CARTESIAN_POINT('Ctrl Pts',(23.7076868253652,-10.9259072644299,-6.29504943074994E-5));
#58654=CARTESIAN_POINT('Ctrl Pts',(23.4923131746348,-10.9243498732306,-0.000207109954374048));
#58655=CARTESIAN_POINT('Ctrl Pts',(23.5066269367174,-10.9247984786312,-0.655339882283325));
#58656=CARTESIAN_POINT('Ctrl Pts',(23.5209406988,-10.8668131970724,-1.31039416802399));
#58657=CARTESIAN_POINT('Ctrl Pts',(23.5352544608827,-10.7496563683361,-1.95468885736663));
#58658=CARTESIAN_POINT('Ctrl Pts',(23.5748561395427,-10.4255202636791,-3.73724966161065));
#58659=CARTESIAN_POINT('Ctrl Pts',(23.6144578182028,-9.64845265710961,-5.43745060898089));
#58660=CARTESIAN_POINT('Ctrl Pts',(23.6540594968629,-8.51270634152007,-6.849069375431));
#58661=CARTESIAN_POINT('Ctrl Pts',(23.693661175523,-7.37696002593053,-8.26068814188111));
#58662=CARTESIAN_POINT('Ctrl Pts',(23.7332628541831,-5.88253500132106,-9.383724727411));
#58663=CARTESIAN_POINT('Ctrl Pts',(23.7728645328431,-4.21069443082789,-10.0819627541773));
#58664=CARTESIAN_POINT('Ctrl Pts',(23.8124662115032,-2.53885386033478,-10.7802007809435));
#58665=CARTESIAN_POINT('Ctrl Pts',(23.8520678901633,-0.689597743957951,
-11.0536402489461));
#58666=CARTESIAN_POINT('Ctrl Pts',(23.8916695688233,1.11277225874495,-10.8691148888302));
#58667=CARTESIAN_POINT('Ctrl Pts',(23.9312712474834,2.91514226144791,-10.6845895287144));
#58668=CARTESIAN_POINT('Ctrl Pts',(23.9708729261435,4.67062615047709,-10.0420993404801));
#58669=CARTESIAN_POINT('Ctrl Pts',(24.0104746048036,6.16629617280339,-9.01957383004835));
#58670=CARTESIAN_POINT('Ctrl Pts',(24.0500762834636,7.66196619512969,-7.99704831961655));
#58671=CARTESIAN_POINT('Ctrl Pts',(24.0896779621237,8.8978223507531,-6.59448748698719));
#58672=CARTESIAN_POINT('Ctrl Pts',(24.1292796407838,9.72396404763253,-4.98201201993459));
#58673=CARTESIAN_POINT('Ctrl Pts',(24.1688813194439,10.550105744512,-3.36953655288199));
#58674=CARTESIAN_POINT('Ctrl Pts',(24.2084829981039,10.9665329826474,-1.54714645140614));
#58675=CARTESIAN_POINT('Ctrl Pts',(24.248084676764,10.9227360896514,0.264115282119209));
#58676=CARTESIAN_POINT('Ctrl Pts',(24.2876863554241,10.8789391966555,2.07537701564461));
#58677=CARTESIAN_POINT('Ctrl Pts',(24.3272880340842,10.374918172528,3.87551038121951));
#58678=CARTESIAN_POINT('Ctrl Pts',(24.3668897127443,9.47180719504063,5.44617196078122));
#58679=CARTESIAN_POINT('Ctrl Pts',(24.4064913914043,8.56869621755328,7.01683354034283));
#58680=CARTESIAN_POINT('Ctrl Pts',(24.4460930700644,7.26649528670601,8.35802333389129));
#58681=CARTESIAN_POINT('Ctrl Pts',(24.4856947487245,5.72315214552883,9.30706452570044));
#58682=CARTESIAN_POINT('Ctrl Pts',(24.5252964273845,4.17980900435165,10.2561057175096));
#58683=CARTESIAN_POINT('Ctrl Pts',(24.5648981060446,2.39532365284457,10.8129983075794));
#58684=CARTESIAN_POINT('Ctrl Pts',(24.6044997847047,0.586141515875516,10.9101951719385));
#58685=CARTESIAN_POINT('Ctrl Pts',(24.6441014633648,-1.22304062109364,11.0073920362976));
#58686=CARTESIAN_POINT('Ctrl Pts',(24.6837031420249,-3.05691954352477,10.6448931749458));
#58687=CARTESIAN_POINT('Ctrl Pts',(24.7233048206849,-4.69305873649397,9.86666713040632));
#58688=CARTESIAN_POINT('Ctrl Pts',(24.762906499345,-6.32919792946312,9.08844108586681));
#58689=CARTESIAN_POINT('Ctrl Pts',(24.8025081780051,-7.76759739297034,7.89448785813953));
#58690=CARTESIAN_POINT('Ctrl Pts',(24.8421098566652,-8.83378946733678,6.42962551111591));
#58691=CARTESIAN_POINT('Ctrl Pts',(24.8817115353252,-9.89998154170322,4.9647631640923));
#58692=CARTESIAN_POINT('Ctrl Pts',(24.9213132139853,-10.5939662269289,3.22899169777235));
#58693=CARTESIAN_POINT('Ctrl Pts',(24.9609148926454,-10.8315680995962,1.4328478880304));
#58694=CARTESIAN_POINT('Ctrl Pts',(24.9713809866419,-10.8943624966322,0.958155638105639));
#58695=CARTESIAN_POINT('Ctrl Pts',(24.9818470806384,-10.9252803407565,0.479246616325014));
#58696=CARTESIAN_POINT('Ctrl Pts',(24.9923131746348,-10.9248114762173,0.000277509097762489));
#58697=CARTESIAN_POINT('Origin',(21.9,0.,0.));
#58698=CARTESIAN_POINT('',(26.7076868253652,-10.9253817421283,0.000250763240793613));
#58699=CARTESIAN_POINT('',(26.4923131746348,-10.9256477953395,-0.000188607126753371));
#58700=CARTESIAN_POINT('',(21.9,-10.925,-1.33792662806848E-15));
#58701=CARTESIAN_POINT('Ctrl Pts',(26.7076868253652,-10.9253817421283,0.000250763240793613));
#58702=CARTESIAN_POINT('Ctrl Pts',(26.7011962734637,-10.9256744620931,0.297238919885603));
#58703=CARTESIAN_POINT('Ctrl Pts',(26.6947057215622,-10.9138078189524,0.59420375076102));
#58704=CARTESIAN_POINT('Ctrl Pts',(26.6882151696607,-10.8896150816089,0.890160997050293));
#58705=CARTESIAN_POINT('Ctrl Pts',(26.648527128711,-10.7416827693886,2.69986277408845));
#58706=CARTESIAN_POINT('Ctrl Pts',(26.6088390877613,-10.1328771529819,4.47189091097551));
#58707=CARTESIAN_POINT('Ctrl Pts',(26.5691510468115,-9.13735775218322,5.99039201846518));
#58708=CARTESIAN_POINT('Ctrl Pts',(26.5294630058618,-8.14183835138456,7.50889312595481));
#58709=CARTESIAN_POINT('Ctrl Pts',(26.4897749649121,-6.75960516619393,8.77386720404705));
#58710=CARTESIAN_POINT('Ctrl Pts',(26.4500869239624,-5.1590300816516,9.63122587435723));
#58711=CARTESIAN_POINT('Ctrl Pts',(26.4103988830126,-3.55845499710918,10.4885845446675));
#58712=CARTESIAN_POINT('Ctrl Pts',(26.3707108420629,-1.73953801321505,10.9383278071956));
#58713=CARTESIAN_POINT('Ctrl Pts',(26.3310228011132,0.0761558804246215,
10.9256717646171));
#58714=CARTESIAN_POINT('Ctrl Pts',(26.2913347601634,1.89184977406434,10.9130157220386));
#58715=CARTESIAN_POINT('Ctrl Pts',(26.2516467192137,3.70432057744957,10.4379603743534));
#58716=CARTESIAN_POINT('Ctrl Pts',(26.211958678264,5.29278851983245,9.55837292171655));
#58717=CARTESIAN_POINT('Ctrl Pts',(26.1722706373142,6.88125646221528,8.6787854690797));
#58718=CARTESIAN_POINT('Ctrl Pts',(26.1325825963645,8.24572154359574,7.39466591149117));
#58719=CARTESIAN_POINT('Ctrl Pts',(26.0928945554148,9.21997623814888,5.8624347667368));
#58720=CARTESIAN_POINT('Ctrl Pts',(26.053206514465,10.194230932702,4.33020362198251));
#58721=CARTESIAN_POINT('Ctrl Pts',(26.0135184735153,10.7782752404278,2.54986089006244));
#58722=CARTESIAN_POINT('Ctrl Pts',(25.9738304325656,10.9009658534587,0.738272773439941));
#58723=CARTESIAN_POINT('Ctrl Pts',(25.9341423916158,11.0236564664896,-1.07331534318261));
#58724=CARTESIAN_POINT('Ctrl Pts',(25.8944543506661,10.6849933848255,-2.91614884450771));
#58725=CARTESIAN_POINT('Ctrl Pts',(25.8547663097164,9.92622966335209,-4.56574943428384));
#58726=CARTESIAN_POINT('Ctrl Pts',(25.8150782687667,9.16746594187869,-6.21535002405998));
#58727=CARTESIAN_POINT('Ctrl Pts',(25.7753902278169,7.98860158059606,-7.67171770228717));
#58728=CARTESIAN_POINT('Ctrl Pts',(25.7357021868672,6.53323580490431,-8.75745015080249));
#58729=CARTESIAN_POINT('Ctrl Pts',(25.6960141459175,5.07787002921256,-9.84318259931782));
#58730=CARTESIAN_POINT('Ctrl Pts',(25.6563261049677,3.34600283911165,-10.5582798181212));
#58731=CARTESIAN_POINT('Ctrl Pts',(25.616638064018,1.54859555904473,-10.8156347488615));
#58732=CARTESIAN_POINT('Ctrl Pts',(25.5769500230683,-0.248811721022244,
-11.0729896796019));
#58733=CARTESIAN_POINT('Ctrl Pts',(25.5372619821185,-2.11175909105534,-10.8726023222793));
#58734=CARTESIAN_POINT('Ctrl Pts',(25.4975739411688,-3.81331815446851,-10.2388821596439));
#58735=CARTESIAN_POINT('Ctrl Pts',(25.4578859002191,-5.51487721788164,-9.6051619970086));
#58736=CARTESIAN_POINT('Ctrl Pts',(25.4181978592693,-7.05504797467484,-8.53810902906051));
#58737=CARTESIAN_POINT('Ctrl Pts',(25.3785098183196,-8.24621992874398,-7.16770256867986));
#58738=CARTESIAN_POINT('Ctrl Pts',(25.3388217773699,-9.43739188281316,-5.79729610829917));
#58739=CARTESIAN_POINT('Ctrl Pts',(25.2991337364202,-10.2795650341583,-4.12353615548591));
#58740=CARTESIAN_POINT('Ctrl Pts',(25.2594456954704,-10.6701530156297,-2.35030590547769));
#58741=CARTESIAN_POINT('Ctrl Pts',(25.2421927387687,-10.8399471745573,-1.57945745860301));
#58742=CARTESIAN_POINT('Ctrl Pts',(25.224939782067,-10.9244023605542,-0.789811465736947));
#58743=CARTESIAN_POINT('Ctrl Pts',(25.2076868253652,-10.9241289668202,-0.000107867347247034));
#58744=CARTESIAN_POINT('Ctrl Pts',(24.9923131746348,-10.9248114762173,0.000277509097762489));
#58745=CARTESIAN_POINT('Ctrl Pts',(25.0214487592984,-10.9235062478788,-1.33307999558033));
#58746=CARTESIAN_POINT('Ctrl Pts',(25.050584343962,-10.6789671832647,-2.66690313728472));
#58747=CARTESIAN_POINT('Ctrl Pts',(25.0797199286256,-10.2017618572325,-3.91151832090029));
#58748=CARTESIAN_POINT('Ctrl Pts',(25.1193216072857,-9.55313468209254,-5.60322456692508));
#58749=CARTESIAN_POINT('Ctrl Pts',(25.1589232859458,-8.47466127170361,-7.13012090581071));
#58750=CARTESIAN_POINT('Ctrl Pts',(25.1985249646059,-7.09715280662447,-8.30700563415272));
#58751=CARTESIAN_POINT('Ctrl Pts',(25.2381266432659,-5.71964434154533,-9.48389036249474));
#58752=CARTESIAN_POINT('Ctrl Pts',(25.277728321926,-4.04310082177598,-10.3107634802931));
#58753=CARTESIAN_POINT('Ctrl Pts',(25.3173300005861,-2.27087509307646,-10.6873311391604));
#58754=CARTESIAN_POINT('Ctrl Pts',(25.3569316792461,-0.498649364376934,
-11.0638987980277));
#58755=CARTESIAN_POINT('Ctrl Pts',(25.3965333579062,1.36925857325276,-10.9901609979639));
#58756=CARTESIAN_POINT('Ctrl Pts',(25.4361350365663,3.1062847265397,-10.4750616114698));
#58757=CARTESIAN_POINT('Ctrl Pts',(25.4757367152264,4.84331087982664,-9.95996222497581));
#58758=CARTESIAN_POINT('Ctrl Pts',(25.5153383938864,6.44945524877083,-9.00350125205159));
#58759=CARTESIAN_POINT('Ctrl Pts',(25.5549400725465,7.72990390562453,-7.72169062940451));
#58760=CARTESIAN_POINT('Ctrl Pts',(25.5945417512066,9.01035256247823,-6.43988000675743));
#58761=CARTESIAN_POINT('Ctrl Pts',(25.6341434298667,9.96510550724145,-4.83271973438749));
#58762=CARTESIAN_POINT('Ctrl Pts',(25.6737451085268,10.4783579749164,-3.09514696192733));
#58763=CARTESIAN_POINT('Ctrl Pts',(25.7133467871868,10.9916104425914,-1.35757418946712));
#58764=CARTESIAN_POINT('Ctrl Pts',(25.7529484658469,11.0633624331782,0.510411083083306));
#58765=CARTESIAN_POINT('Ctrl Pts',(25.792550144507,10.6849109387901,2.28223548227329));
#58766=CARTESIAN_POINT('Ctrl Pts',(25.8321518231671,10.306459444402,4.05405988146317));
#58767=CARTESIAN_POINT('Ctrl Pts',(25.8717535018271,9.4778044650391,5.72972340729261));
#58768=CARTESIAN_POINT('Ctrl Pts',(25.9113551804872,8.29945597626702,7.10597995102917));
#58769=CARTESIAN_POINT('Ctrl Pts',(25.9509568591473,7.12110748749493,8.48223649476573));
#58770=CARTESIAN_POINT('Ctrl Pts',(25.9905585378074,5.59306548931364,9.5590860564094));
#58771=CARTESIAN_POINT('Ctrl Pts',(26.0301602164674,3.90067064547983,10.2059144167446));
#58772=CARTESIAN_POINT('Ctrl Pts',(26.0697618951275,2.20827580164592,10.8527427770798));
#58773=CARTESIAN_POINT('Ctrl Pts',(26.1093635737876,0.351528112159476,11.0695499361064));
#58774=CARTESIAN_POINT('Ctrl Pts',(26.1489652524477,-1.44436208870353,10.830038722144));
#58775=CARTESIAN_POINT('Ctrl Pts',(26.1885669311077,-3.24025228956654,10.5905275081816));
#58776=CARTESIAN_POINT('Ctrl Pts',(26.2281686097678,-4.97528500180612,9.89469792123011));
#58777=CARTESIAN_POINT('Ctrl Pts',(26.2677702884279,-6.43901305518162,8.82694915820995));
#58778=CARTESIAN_POINT('Ctrl Pts',(26.307371967088,-7.90274110855705,7.75920039518985));
#58779=CARTESIAN_POINT('Ctrl Pts',(26.346973645748,-9.09516450306844,6.31953245610114));
#58780=CARTESIAN_POINT('Ctrl Pts',(26.3865753244081,-9.87165073275015,4.68256685771984));
#58781=CARTESIAN_POINT('Ctrl Pts',(26.4218212744837,-10.5627324194797,3.22564862323762));
#58782=CARTESIAN_POINT('Ctrl Pts',(26.4570672245593,-10.9243417515293,1.61244686836693));
#58783=CARTESIAN_POINT('Ctrl Pts',(26.4923131746348,-10.9256477953395,-0.000188607126753371));
#58784=CARTESIAN_POINT('Origin',(21.9,0.,0.));
#58785=CARTESIAN_POINT('',(28.2076868253652,-10.9249562302737,-0.000283622248641526));
#58786=CARTESIAN_POINT('',(27.9923131746348,-10.9240771448479,-2.63224792766081E-5));
#58787=CARTESIAN_POINT('',(21.9,-10.925,-1.33792662806848E-15));
#58788=CARTESIAN_POINT('Ctrl Pts',(28.2076868253652,-10.9249562302737,-0.000283622248641526));
#58789=CARTESIAN_POINT('Ctrl Pts',(28.1774527648605,-10.9235442202493,1.38329143549077));
#58790=CARTESIAN_POINT('Ctrl Pts',(28.1472187043558,-10.6597816637334,2.76738948567407));
#58791=CARTESIAN_POINT('Ctrl Pts',(28.116984643851,-10.1468053659073,4.05196792838614));
#58792=CARTESIAN_POINT('Ctrl Pts',(28.0772966029013,-9.47342494744909,5.73822511602129));
#58793=CARTESIAN_POINT('Ctrl Pts',(28.0376085619516,-8.3706086232334,7.25299379523649));
#58794=CARTESIAN_POINT('Ctrl Pts',(27.9979205210018,-6.97269209388642,8.41175773486898));
#58795=CARTESIAN_POINT('Ctrl Pts',(27.9582324800521,-5.57477556453952,9.5705216745014));
#58796=CARTESIAN_POINT('Ctrl Pts',(27.9185444391024,-3.88175883006137,10.3732808745511));
#58797=CARTESIAN_POINT('Ctrl Pts',(27.8788563981526,-2.09987078297384,10.7222500400376));
#58798=CARTESIAN_POINT('Ctrl Pts',(27.8391683572029,-0.317982735886218,
11.0712192055241));
#58799=CARTESIAN_POINT('Ctrl Pts',(27.7994803162532,1.55277662381079,10.9663983364473));
#58800=CARTESIAN_POINT('Ctrl Pts',(27.7597922753034,3.28452730942337,10.4205558191455));
#58801=CARTESIAN_POINT('Ctrl Pts',(27.7201042343537,5.0162779950359,9.87471330184359));
#58802=CARTESIAN_POINT('Ctrl Pts',(27.680416193404,6.60902000656401,8.88784913631665));
#58803=CARTESIAN_POINT('Ctrl Pts',(27.6407281524542,7.86873906498655,7.58017471786955));
#58804=CARTESIAN_POINT('Ctrl Pts',(27.6010401115045,9.12845812340909,6.27250029942246));
#58805=CARTESIAN_POINT('Ctrl Pts',(27.5613520705548,10.055154228726,4.64401562805519));
#58806=CARTESIAN_POINT('Ctrl Pts',(27.5216640296051,10.5359451467504,2.89308884947215));
#58807=CARTESIAN_POINT('Ctrl Pts',(27.4819759886554,11.0167360647748,1.14216207088907));
#58808=CARTESIAN_POINT('Ctrl Pts',(27.4422879477056,11.0516217955067,-0.731206814909807));
#58809=CARTESIAN_POINT('Ctrl Pts',(27.4025999067559,10.6363528560748,-2.49881995096567));
#58810=CARTESIAN_POINT('Ctrl Pts',(27.3629118658061,10.2210839166429,-4.26643308702153));
#58811=CARTESIAN_POINT('Ctrl Pts',(27.3232238248564,9.35566030704735,-5.92829047333437));
#58812=CARTESIAN_POINT('Ctrl Pts',(27.2835357839067,8.14550056742096,-7.28195878403737));
#58813=CARTESIAN_POINT('Ctrl Pts',(27.243847742957,6.93534082779465,-8.6356270947403));
#58814=CARTESIAN_POINT('Ctrl Pts',(27.2041597020072,5.38044495813755,-9.6811063298334));
#58815=CARTESIAN_POINT('Ctrl Pts',(27.1644716610575,3.67021714250521,-10.2910451049996));
#58816=CARTESIAN_POINT('Ctrl Pts',(27.1247836201077,1.95998932687278,-10.9009838801657));
#58817=CARTESIAN_POINT('Ctrl Pts',(27.085095579158,0.0944295652650959,-11.0753821954049));
#58818=CARTESIAN_POINT('Ctrl Pts',(27.0454075382083,-1.6992155264193,-10.7929963319298));
#58819=CARTESIAN_POINT('Ctrl Pts',(27.0057194972586,-3.49286061810369,-10.5106104684547));
#58820=CARTESIAN_POINT('Ctrl Pts',(26.9660314563088,-5.21459103986479,-9.77144042626522));
#58821=CARTESIAN_POINT('Ctrl Pts',(26.9263434153591,-6.65468024212393,-8.66552561021891));
#58822=CARTESIAN_POINT('Ctrl Pts',(26.8866553744094,-8.09476944438298,-7.55961079417266));
#58823=CARTESIAN_POINT('Ctrl Pts',(26.8469673334596,-9.2532174271401,-6.08695120426957));
#58824=CARTESIAN_POINT('Ctrl Pts',(26.8072792925099,-9.98891191450167,-4.42693370072344));
#58825=CARTESIAN_POINT('Ctrl Pts',(26.7740818034617,-10.604291487355,-3.03839419171485));
#58826=CARTESIAN_POINT('Ctrl Pts',(26.7408843144135,-10.9238845554525,-1.51876660651429));
#58827=CARTESIAN_POINT('Ctrl Pts',(26.7076868253652,-10.9253817421283,0.000250763240793613));
#58828=CARTESIAN_POINT('Ctrl Pts',(26.4923131746348,-10.9256477953395,-0.000188607126753371));
#58829=CARTESIAN_POINT('Ctrl Pts',(26.4966689032193,-10.9258091974962,-0.199479658210317));
#58830=CARTESIAN_POINT('Ctrl Pts',(26.5010246318038,-10.9204679558336,-0.398762060930637));
#58831=CARTESIAN_POINT('Ctrl Pts',(26.5053803603884,-10.9095658812786,-0.597739783237097));
#58832=CARTESIAN_POINT('Ctrl Pts',(26.5449820390484,-10.8104457352734,-2.40681756813896));
#58833=CARTESIAN_POINT('Ctrl Pts',(26.5845837177085,-10.2516563784108,-4.1907098802687));
#58834=CARTESIAN_POINT('Ctrl Pts',(26.6241853963686,-9.3009749990302,-5.73304322623142));
#58835=CARTESIAN_POINT('Ctrl Pts',(26.6637870750287,-8.35029361964961,-7.27537657219414));
#58836=CARTESIAN_POINT('Ctrl Pts',(26.7033887536887,-7.00772021775101,-8.57615095198983));
#58837=CARTESIAN_POINT('Ctrl Pts',(26.7429904323488,-5.43609943094654,-9.47759165311977));
#58838=CARTESIAN_POINT('Ctrl Pts',(26.7825921110089,-3.86447864414216,-10.3790323542497));
#58839=CARTESIAN_POINT('Ctrl Pts',(26.8221937896689,-2.06381047243195,-10.8811393767138));
#58840=CARTESIAN_POINT('Ctrl Pts',(26.861795468329,-0.252503202072115,-10.9230106975763));
#58841=CARTESIAN_POINT('Ctrl Pts',(26.9013971469891,1.55880406828783,-10.9648820184388));
#58842=CARTESIAN_POINT('Ctrl Pts',(26.9409988256492,3.38075043729737,-10.5465176376995));
#58843=CARTESIAN_POINT('Ctrl Pts',(26.9806005043093,4.99234672418582,-9.71866218941341));
#58844=CARTESIAN_POINT('Ctrl Pts',(27.0202021829694,6.60394301107418,-8.8908067411274));
#58845=CARTESIAN_POINT('Ctrl Pts',(27.0598038616294,8.00518921584144,-7.65346022529469));
#58846=CARTESIAN_POINT('Ctrl Pts',(27.0994055402895,9.02612410575502,-6.1567040040862));
#58847=CARTESIAN_POINT('Ctrl Pts',(27.1390072189496,10.0470589956686,-4.65994778287766));
#58848=CARTESIAN_POINT('Ctrl Pts',(27.1786088976096,10.6876825707285,-2.90378185629335));
#58849=CARTESIAN_POINT('Ctrl Pts',(27.2182105762697,10.8702917319615,-1.10121670368356));
#58850=CARTESIAN_POINT('Ctrl Pts',(27.2578122549298,11.0529008931945,0.701348448926171));
#58851=CARTESIAN_POINT('Ctrl Pts',(27.2974139335899,10.7774956406007,2.55031282756149));
#58852=CARTESIAN_POINT('Ctrl Pts',(27.3370156122499,10.0774806792723,4.22141015838503));
#58853=CARTESIAN_POINT('Ctrl Pts',(27.37661729091,9.37746571794387,5.89250748920862));
#58854=CARTESIAN_POINT('Ctrl Pts',(27.4162189695701,8.25284104788074,7.38573777222065));
#58855=CARTESIAN_POINT('Ctrl Pts',(27.4558206482302,6.84001567032436,8.51998275797199));
#58856=CARTESIAN_POINT('Ctrl Pts',(27.4954223268902,5.42719029276798,9.65422774372333));
#58857=CARTESIAN_POINT('Ctrl Pts',(27.5350240055503,3.72616420771845,10.429487432214));
#58858=CARTESIAN_POINT('Ctrl Pts',(27.5746256842104,1.94325982257379,10.7517283182004));
#58859=CARTESIAN_POINT('Ctrl Pts',(27.6142273628705,0.160355437429085,11.0739692041869));
#58860=CARTESIAN_POINT('Ctrl Pts',(27.6538290415305,-1.70442724781058,10.9431912876689));
#58861=CARTESIAN_POINT('Ctrl Pts',(27.6934307201906,-3.42490331083571,10.3752570029783));
#58862=CARTESIAN_POINT('Ctrl Pts',(27.7330323988507,-5.14537937386074,9.80732271828762));
#58863=CARTESIAN_POINT('Ctrl Pts',(27.7726340775108,-6.7215488146711,8.8022320654244));
#58864=CARTESIAN_POINT('Ctrl Pts',(27.8122357561709,-7.9622334518424,7.48189541658961));
#58865=CARTESIAN_POINT('Ctrl Pts',(27.8518374348309,-9.20291808901377,6.16155876775475));
#58866=CARTESIAN_POINT('Ctrl Pts',(27.891439113491,-10.108117922546,4.52597612294822));
#58867=CARTESIAN_POINT('Ctrl Pts',(27.9310407921511,-10.5680386286055,2.7735320641243));
#58868=CARTESIAN_POINT('Ctrl Pts',(27.9514649196457,-10.8052376427833,1.86972843519824));
#58869=CARTESIAN_POINT('Ctrl Pts',(27.9718890471402,-10.9239983548901,0.934841230600434));
#58870=CARTESIAN_POINT('Ctrl Pts',(27.9923131746348,-10.9240771448479,-2.63224792766081E-5));
#58871=CARTESIAN_POINT('Origin',(21.9,0.,0.));
#58872=CARTESIAN_POINT('',(29.7076868253652,-10.9243494180749,0.000211015426421293));
#58873=CARTESIAN_POINT('',(29.4923131746348,-10.9254954065067,0.000226940750081131));
#58874=CARTESIAN_POINT('',(21.9,-10.925,-1.33792662806848E-15));
#58875=CARTESIAN_POINT('Ctrl Pts',(29.7076868253652,-10.9243494180749,0.000211015426421293));
#58876=CARTESIAN_POINT('Ctrl Pts',(29.693397297207,-10.9248040475345,0.654234556655938));
#58877=CARTESIAN_POINT('Ctrl Pts',(29.6791077690488,-10.8670216803897,1.30817870004611));
#58878=CARTESIAN_POINT('Ctrl Pts',(29.6648182408905,-10.750259360702,1.95141664026735));
#58879=CARTESIAN_POINT('Ctrl Pts',(29.6251301999408,-10.4259611981712,3.73795944484631));
#58880=CARTESIAN_POINT('Ctrl Pts',(29.585442158991,-9.64668758285385,5.44191385414187));
#58881=CARTESIAN_POINT('Ctrl Pts',(29.5457541180413,-8.50736299563991,6.85571864115579));
#58882=CARTESIAN_POINT('Ctrl Pts',(29.5060660770916,-7.36803840842591,8.26952342816979));
#58883=CARTESIAN_POINT('Ctrl Pts',(29.4663780361419,-5.86866284931526,9.39317859290215));
#58884=CARTESIAN_POINT('Ctrl Pts',(29.4266899951921,-4.19187749056147,10.0898100244949));
#58885=CARTESIAN_POINT('Ctrl Pts',(29.3870019542424,-2.51509213180773,10.7864414560877));
#58886=CARTESIAN_POINT('Ctrl Pts',(29.3473139132927,-0.660896973410962,
11.0560491545409));
#58887=CARTESIAN_POINT('Ctrl Pts',(29.307625872343,1.144845707991,10.8657918041516));
#58888=CARTESIAN_POINT('Ctrl Pts',(29.2679378313932,2.95058838939292,10.6755344537624));
#58889=CARTESIAN_POINT('Ctrl Pts',(29.2282497904435,4.70787859379991,10.0254120545306));
#58890=CARTESIAN_POINT('Ctrl Pts',(29.1885617494937,6.20265818149363,8.99461698516531));
#58891=CARTESIAN_POINT('Ctrl Pts',(29.148873708544,7.69743776918753,7.96382191579986));
#58892=CARTESIAN_POINT('Ctrl Pts',(29.1091856675943,8.92970674016811,6.55235417630068));
#58893=CARTESIAN_POINT('Ctrl Pts',(29.0694976266446,9.74936057390753,4.93214675635386));
#58894=CARTESIAN_POINT('Ctrl Pts',(29.0298095856948,10.5690144076468,3.31193933640722));
#58895=CARTESIAN_POINT('Ctrl Pts',(28.9901215447451,10.9760531041451,1.48299223601295));
#58896=CARTESIAN_POINT('Ctrl Pts',(28.9504335037954,10.9208946729335,-0.331907771778112));
#58897=CARTESIAN_POINT('Ctrl Pts',(28.9107454628456,10.8657362417219,-2.14680777956927));
#58898=CARTESIAN_POINT('Ctrl Pts',(28.8710574218959,10.3483806828004,-3.94766069475726));
#58899=CARTESIAN_POINT('Ctrl Pts',(28.8313693809462,9.43184784811948,-5.51510193887641));
#58900=CARTESIAN_POINT('Ctrl Pts',(28.7916813399964,8.51531501343853,-7.08254318299556));
#58901=CARTESIAN_POINT('Ctrl Pts',(28.7519932990467,7.1996049029981,-8.4165727560459));
#58902=CARTESIAN_POINT('Ctrl Pts',(28.712305258097,5.64498612692489,-9.35469052684801));
#58903=CARTESIAN_POINT('Ctrl Pts',(28.6726172171472,4.09036735085176,-10.2928082976501));
#58904=CARTESIAN_POINT('Ctrl Pts',(28.6329291761975,2.29683990914585,-10.8350142662039));
#58905=CARTESIAN_POINT('Ctrl Pts',(28.5932411352478,0.482876053426483,-10.9152615151128));
#58906=CARTESIAN_POINT('Ctrl Pts',(28.5535530942981,-1.33108780229304,-10.9955087640216));
#58907=CARTESIAN_POINT('Ctrl Pts',(28.5138650533483,-3.16548807202591,-10.6137972932853));
#58908=CARTESIAN_POINT('Ctrl Pts',(28.4741770123986,-4.79687372403434,-9.81662394624258));
#58909=CARTESIAN_POINT('Ctrl Pts',(28.4344889714489,-6.42825937604272,-9.01945059919988));
#58910=CARTESIAN_POINT('Ctrl Pts',(28.3948009304991,-7.85663041032657,-7.80681537585078));
#58911=CARTESIAN_POINT('Ctrl Pts',(28.3551128895494,-8.90799482166121,-6.32643118065244));
#58912=CARTESIAN_POINT('Ctrl Pts',(28.3154248485997,-9.95935923299579,-4.84604698545418));
#58913=CARTESIAN_POINT('Ctrl Pts',(28.2757368076499,-10.6337170213812,-3.09791381840668));
#58914=CARTESIAN_POINT('Ctrl Pts',(28.2360487667002,-10.8489236592236,-1.29497438685545));
#58915=CARTESIAN_POINT('Ctrl Pts',(28.2265947862552,-10.9001874479396,-0.865501081509));
#58916=CARTESIAN_POINT('Ctrl Pts',(28.2171408058102,-10.9253977559879,-0.43291792017934));
#58917=CARTESIAN_POINT('Ctrl Pts',(28.2076868253652,-10.9249562302737,-0.000283622248641526));
#58918=CARTESIAN_POINT('Ctrl Pts',(27.9923131746348,-10.9240771448479,-2.63224792766081E-5));
#58919=CARTESIAN_POINT('Ctrl Pts',(28.0114907258003,-10.9241511259003,-0.877834705574352));
#58920=CARTESIAN_POINT('Ctrl Pts',(28.0306682769658,-10.8195884523745,-1.75562576278631));
#58921=CARTESIAN_POINT('Ctrl Pts',(28.0498458281313,-10.6101874446618,-2.60765085001121));
#58922=CARTESIAN_POINT('Ctrl Pts',(28.0894475067914,-10.1777739760717,-4.36708423248161));
#58923=CARTESIAN_POINT('Ctrl Pts',(28.1290491854515,-9.29830546030464,-6.01664552458103));
#58924=CARTESIAN_POINT('Ctrl Pts',(28.1686508641115,-8.07845519473027,-7.35625463351821));
#58925=CARTESIAN_POINT('Ctrl Pts',(28.2082525427716,-6.8586049291559,-8.6958637424554));
#58926=CARTESIAN_POINT('Ctrl Pts',(28.2478542214317,-5.29837291377423,-9.72552066823035));
#58927=CARTESIAN_POINT('Ctrl Pts',(28.2874559000918,-3.58700423326845,-10.3203353238612));
#58928=CARTESIAN_POINT('Ctrl Pts',(28.3270575787519,-1.87563555276267,-10.915149979492));
#58929=CARTESIAN_POINT('Ctrl Pts',(28.3666592574119,-0.0131302071327644,
-11.0751223649788));
#58930=CARTESIAN_POINT('Ctrl Pts',(28.406260936072,1.77460310646482,-10.7808489638316));
#58931=CARTESIAN_POINT('Ctrl Pts',(28.4458626147321,3.56233642006241,-10.4865755626844));
#58932=CARTESIAN_POINT('Ctrl Pts',(28.4854642933921,5.27529770162768,-9.73805637490325));
#58933=CARTESIAN_POINT('Ctrl Pts',(28.5250659720522,6.70571688902053,-8.62608147253013));
#58934=CARTESIAN_POINT('Ctrl Pts',(28.5646676507123,8.13613607641334,-7.51410657015704));
#58935=CARTESIAN_POINT('Ctrl Pts',(28.6042693293724,9.28401316963376,-6.03867595319197));
#58936=CARTESIAN_POINT('Ctrl Pts',(28.6438710080324,10.0101188133226,-4.37874889775477));
#58937=CARTESIAN_POINT('Ctrl Pts',(28.6834726866925,10.7362244570114,-2.71882184231747));
#58938=CARTESIAN_POINT('Ctrl Pts',(28.7230743653526,11.0405586511686,-0.874398348408018));
#58939=CARTESIAN_POINT('Ctrl Pts',(28.7626760440127,10.886207815136,0.930806087268328));
#58940=CARTESIAN_POINT('Ctrl Pts',(28.8022777226728,10.7318569791033,2.73601052294457));
#58941=CARTESIAN_POINT('Ctrl Pts',(28.8418794013328,10.1188211128809,4.50199590038771));
#58942=CARTESIAN_POINT('Ctrl Pts',(28.8814810799929,9.12145712189901,6.01456071045763));
#58943=CARTESIAN_POINT('Ctrl Pts',(28.921082758653,8.1240931309171,7.52712552052759));
#58944=CARTESIAN_POINT('Ctrl Pts',(28.9606844373131,6.7424010151757,8.78626976322431));
#58945=CARTESIAN_POINT('Ctrl Pts',(29.0002861159731,5.1439702350062,9.63926816660855));
#58946=CARTESIAN_POINT('Ctrl Pts',(29.0398877946332,3.5455394548367,10.4922665699928));
#58947=CARTESIAN_POINT('Ctrl Pts',(29.0794894732933,1.7303700102391,10.9391191340646));
#58948=CARTESIAN_POINT('Ctrl Pts',(29.1190911519534,-0.0813709109128266,
10.9256258100523));
#58949=CARTESIAN_POINT('Ctrl Pts',(29.1586928306134,-1.89311183206476,10.91213248604));
#58950=CARTESIAN_POINT('Ctrl Pts',(29.1982945092735,-3.70142422977101,10.4382932739436));
#58951=CARTESIAN_POINT('Ctrl Pts',(29.2378961879336,-5.28697262734363,9.56158151166123));
#58952=CARTESIAN_POINT('Ctrl Pts',(29.2774978665937,-6.87252102491625,8.68486974937887));
#58953=CARTESIAN_POINT('Ctrl Pts',(29.3170995452538,-8.23530542235523,7.40528543691051));
#58954=CARTESIAN_POINT('Ctrl Pts',(29.3567012239138,-9.21002973154307,5.87803308178132));
#58955=CARTESIAN_POINT('Ctrl Pts',(29.3963029025739,-10.1847540407309,4.3507807266521));
#58956=CARTESIAN_POINT('Ctrl Pts',(29.435904581234,-10.7714182616676,2.57586032886204));
#58957=CARTESIAN_POINT('Ctrl Pts',(29.475506259894,-10.8988641825762,0.76855715218877));
#58958=CARTESIAN_POINT('Ctrl Pts',(29.4811085648076,-10.9168934917641,0.512884569368697));
#58959=CARTESIAN_POINT('Ctrl Pts',(29.4867108697212,-10.9257325900039,0.256563918801746));
#58960=CARTESIAN_POINT('Ctrl Pts',(29.4923131746348,-10.9254954065067,0.000226940750081131));
#58961=CARTESIAN_POINT('Origin',(21.9,0.,0.));
#58962=CARTESIAN_POINT('',(31.2076868253652,-10.9258901478294,-7.91472659100149E-5));
#58963=CARTESIAN_POINT('',(30.9923131746348,-10.9249872058682,-0.000280213389727673));
#58964=CARTESIAN_POINT('',(21.9,-10.925,-1.33792662806848E-15));
#58965=CARTESIAN_POINT('Ctrl Pts',(31.2076868253652,-10.9258901478294,-7.91472659100149E-5));
#58966=CARTESIAN_POINT('Ctrl Pts',(31.1696537886038,-10.9252124665205,1.7399638103303));
#58967=CARTESIAN_POINT('Ctrl Pts',(31.1316207518423,-10.5019577581781,3.48032470201847));
#58968=CARTESIAN_POINT('Ctrl Pts',(31.0935877150808,-9.70163758884194,5.0253687746317));
#58969=CARTESIAN_POINT('Ctrl Pts',(31.0538996741311,-8.86649155901743,6.63764530168347));
#58970=CARTESIAN_POINT('Ctrl Pts',(31.0142116331814,-7.62075013733753,8.03723678022229));
#58971=CARTESIAN_POINT('Ctrl Pts',(30.9745235922316,-6.11615894363561,9.05365688561591));
#58972=CARTESIAN_POINT('Ctrl Pts',(30.9348355512819,-4.61156774993361,10.0700769910096));
#58973=CARTESIAN_POINT('Ctrl Pts',(30.8951475103322,-2.84812678420957,10.703325723258));
#58974=CARTESIAN_POINT('Ctrl Pts',(30.8554594693824,-1.04064341958794,10.8762661101843));
#58975=CARTESIAN_POINT('Ctrl Pts',(30.8157714284327,0.766839945033689,11.0492064971105));
#58976=CARTESIAN_POINT('Ctrl Pts',(30.776083387483,2.61836570855288,10.7618385387146));
#58977=CARTESIAN_POINT('Ctrl Pts',(30.7363953465332,4.28839675730136,10.0491669544416));
#58978=CARTESIAN_POINT('Ctrl Pts',(30.6967073055835,5.95842780604985,9.33649537016863));
#58979=CARTESIAN_POINT('Ctrl Pts',(30.6570192646338,7.4469641400276,8.1985201600186));
#58980=CARTESIAN_POINT('Ctrl Pts',(30.617331223684,8.57268492915469,6.77385978093128));
#58981=CARTESIAN_POINT('Ctrl Pts',(30.5776431827343,9.69840571828177,5.34919940184396));
#58982=CARTESIAN_POINT('Ctrl Pts',(30.5379551417846,10.4613109625582,3.6378538538194));
#58983=CARTESIAN_POINT('Ctrl Pts',(30.4982671008349,10.7684700367738,1.8482846894837));
#58984=CARTESIAN_POINT('Ctrl Pts',(30.4585790598852,11.0756291109893,0.0587155251481608));
#58985=CARTESIAN_POINT('Ctrl Pts',(30.4188910189354,10.9270420151442,-1.80907725549861));
#58986=CARTESIAN_POINT('Ctrl Pts',(30.3792029779857,10.3408083649096,-3.5275750291795));
#58987=CARTESIAN_POINT('Ctrl Pts',(30.3395149370359,9.75457471467492,-5.24607280286055));
#58988=CARTESIAN_POINT('Ctrl Pts',(30.2998268960862,8.73069451005082,-6.81527556957581));
#58989=CARTESIAN_POINT('Ctrl Pts',(30.2601388551365,7.39388812525126,-8.04403640080916));
#58990=CARTESIAN_POINT('Ctrl Pts',(30.2204508141867,6.0570817404517,-9.2727972320425));
#58991=CARTESIAN_POINT('Ctrl Pts',(30.180762773237,4.40734917547671,-10.1611161277939));
#58992=CARTESIAN_POINT('Ctrl Pts',(30.1410747322873,2.6456468136292,-10.6007856389896));
#58993=CARTESIAN_POINT('Ctrl Pts',(30.1013866913376,0.883944451781801,-11.0404551501853));
#58994=CARTESIAN_POINT('Ctrl Pts',(30.0616986503878,-0.98972770693807,-11.0314752768253));
#58995=CARTESIAN_POINT('Ctrl Pts',(30.0220106094381,-2.74713486344501,-10.5749398706716));
#58996=CARTESIAN_POINT('Ctrl Pts',(29.9823225684883,-4.50454201995206,-10.1184044645178));
#58997=CARTESIAN_POINT('Ctrl Pts',(29.9426345275386,-6.14568417424614,-9.21431352557036));
#58998=CARTESIAN_POINT('Ctrl Pts',(29.9029464865889,-7.47065135375669,-7.97279571899892));
#58999=CARTESIAN_POINT('Ctrl Pts',(29.8632584456392,-8.79561853326725,-6.73127791242747));
#59000=CARTESIAN_POINT('Ctrl Pts',(29.8235704046894,-9.80441073799426,-5.1523332382321));
#59001=CARTESIAN_POINT('Ctrl Pts',(29.7838823637397,-10.3741454854857,-3.42829530120315));
#59002=CARTESIAN_POINT('Ctrl Pts',(29.7584838509482,-10.7387494045919,-2.3249906646221));
#59003=CARTESIAN_POINT('Ctrl Pts',(29.7330853381567,-10.9235413499556,-1.16226440670903));
#59004=CARTESIAN_POINT('Ctrl Pts',(29.7076868253652,-10.9243494180749,0.000211015426421293));
#59005=CARTESIAN_POINT('Ctrl Pts',(29.4923131746348,-10.9254954065067,0.000226940750081131));
#59006=CARTESIAN_POINT('Ctrl Pts',(29.5263125483813,-10.9240559828247,-1.55543574741824));
#59007=CARTESIAN_POINT('Ctrl Pts',(29.5603119221278,-10.5883319981353,-3.11169978603138));
#59008=CARTESIAN_POINT('Ctrl Pts',(29.5943112958743,-9.94378868323232,-4.52735984759813));
#59009=CARTESIAN_POINT('Ctrl Pts',(29.6339129745344,-9.19303964209939,-6.17628771515557));
#59010=CARTESIAN_POINT('Ctrl Pts',(29.6735146531944,-8.02331393895306,-7.63445749471393));
#59011=CARTESIAN_POINT('Ctrl Pts',(29.7131163318545,-6.57649101067561,-8.72500352738757));
#59012=CARTESIAN_POINT('Ctrl Pts',(29.7527180105146,-5.12966808239816,-9.81554956006121));
#59013=CARTESIAN_POINT('Ctrl Pts',(29.7923196891746,-3.40574792898961,-10.5384718458501));
#59014=CARTESIAN_POINT('Ctrl Pts',(29.8319213678347,-1.61382984606914,-10.8060850354955));
#59015=CARTESIAN_POINT('Ctrl Pts',(29.8715230464948,0.178088236851231,-11.0736982251408));
#59016=CARTESIAN_POINT('Ctrl Pts',(29.9111247251549,2.03800424928348,-10.8860023186427));
#59017=CARTESIAN_POINT('Ctrl Pts',(29.950726403815,3.74032356183513,-10.2657634990878));
#59018=CARTESIAN_POINT('Ctrl Pts',(29.990328082475,5.44264287438678,-9.64552467953292));
#59019=CARTESIAN_POINT('Ctrl Pts',(30.0299297611351,6.98736548705781,-8.59274294692128));
#59020=CARTESIAN_POINT('Ctrl Pts',(30.0695314397952,8.18712749578463,-7.23511326339747));
#59021=CARTESIAN_POINT('Ctrl Pts',(30.1091331184553,9.38688950451153,-5.87748357987359));
#59022=CARTESIAN_POINT('Ctrl Pts',(30.1487347971154,10.2416909092942,-4.21500594543754));
#59023=CARTESIAN_POINT('Ctrl Pts',(30.1883364757754,10.647850358487,-2.44932711365614));
#59024=CARTESIAN_POINT('Ctrl Pts',(30.2279381544355,11.0540098076798,-0.68364828187479));
#59025=CARTESIAN_POINT('Ctrl Pts',(30.2675398330956,11.0115273012829,1.18523174725202));
#59026=CARTESIAN_POINT('Ctrl Pts',(30.3071415117556,10.52555566621,2.93063107264261));
#59027=CARTESIAN_POINT('Ctrl Pts',(30.3467431904157,10.039584031137,4.67603039803314));
#59028=CARTESIAN_POINT('Ctrl Pts',(30.3863448690758,9.11012326738821,6.29794901968758));
#59029=CARTESIAN_POINT('Ctrl Pts',(30.4259465477359,7.84991037767281,7.59965970481095));
#59030=CARTESIAN_POINT('Ctrl Pts',(30.465548226396,6.58969748795742,8.90137038993432));
#59031=CARTESIAN_POINT('Ctrl Pts',(30.505149905056,4.99873247227549,9.8828731385266));
#59032=CARTESIAN_POINT('Ctrl Pts',(30.5447515837161,3.26998811041387,10.4251186239858));
#59033=CARTESIAN_POINT('Ctrl Pts',(30.5843532623762,1.54124374855216,10.967364109445));
#59034=CARTESIAN_POINT('Ctrl Pts',(30.6239549410362,-0.32527995948923,11.070352331771));
#59035=CARTESIAN_POINT('Ctrl Pts',(30.6635566196963,-2.10318691767515,10.7215915495668));
#59036=CARTESIAN_POINT('Ctrl Pts',(30.7031582983564,-3.88109387586107,10.3728307673627));
#59037=CARTESIAN_POINT('Ctrl Pts',(30.7427599770165,-5.57038408419148,9.57232098062839));
#59038=CARTESIAN_POINT('Ctrl Pts',(30.7823616556766,-6.96615861393129,8.41715835255424));
#59039=CARTESIAN_POINT('Ctrl Pts',(30.8219633343366,-8.36193314367101,7.26199572448016));
#59040=CARTESIAN_POINT('Ctrl Pts',(30.8615650129967,-9.46419199482014,5.75218025506628));
#59041=CARTESIAN_POINT('Ctrl Pts',(30.9011666916568,-10.1392389814448,4.07084185931777));
#59042=CARTESIAN_POINT('Ctrl Pts',(30.9315488526494,-10.6571308213666,2.78092952349759));
#59043=CARTESIAN_POINT('Ctrl Pts',(30.9619310136421,-10.923571621462,1.39006114744922));
#59044=CARTESIAN_POINT('Ctrl Pts',(30.9923131746348,-10.9249872058682,-0.000280213389727673));
#59045=CARTESIAN_POINT('Origin',(21.9,0.,0.));
#59046=CARTESIAN_POINT('',(32.7076868253652,-10.9241131192016,-9.40179992833195E-5));
#59047=CARTESIAN_POINT('',(32.4923131746348,-10.9242412661389,0.000167712051415234));
#59048=CARTESIAN_POINT('',(21.9,-10.925,-1.33792662806848E-15));
#59049=CARTESIAN_POINT('Ctrl Pts',(32.7076868253652,-10.9241131192016,-9.40179992833195E-5));
#59050=CARTESIAN_POINT('Ctrl Pts',(32.6855983209502,-10.9238085823814,1.01094682114356));
#59051=CARTESIAN_POINT('Ctrl Pts',(32.6635098165353,-10.7846445350471,2.02206980807412));
#59052=CARTESIAN_POINT('Ctrl Pts',(32.6414213121203,-10.5077306005317,2.99394402969129));
#59053=CARTESIAN_POINT('Ctrl Pts',(32.6017332711706,-10.010178961628,4.7401819451649));
#59054=CARTESIAN_POINT('Ctrl Pts',(32.5620452302209,-9.06791623926789,6.35970933256459));
#59055=CARTESIAN_POINT('Ctrl Pts',(32.5223571892711,-7.79572086046838,7.65524914630036));
#59056=CARTESIAN_POINT('Ctrl Pts',(32.4826691483214,-6.52352548166872,8.95078896003628));
#59057=CARTESIAN_POINT('Ctrl Pts',(32.4429811073717,-4.92139744642959,9.9223412001082));
#59058=CARTESIAN_POINT('Ctrl Pts',(32.4032930664219,-3.18449435931388,10.4515596396792));
#59059=CARTESIAN_POINT('Ctrl Pts',(32.3636050254722,-1.44759127219827,10.9807780792503));
#59060=CARTESIAN_POINT('Ctrl Pts',(32.3239169845225,0.424086866793903,11.0676627183205));
#59061=CARTESIAN_POINT('Ctrl Pts',(32.2842289435727,2.20254815309311,10.7016300094696));
#59062=CARTESIAN_POINT('Ctrl Pts',(32.244540902623,3.98100943939252,10.3355973006187));
#59063=CARTESIAN_POINT('Ctrl Pts',(32.2048528616733,5.66625387299894,9.51664724384661));
#59064=CARTESIAN_POINT('Ctrl Pts',(32.1651648207236,7.05299931694725,8.34453736653003));
#59065=CARTESIAN_POINT('Ctrl Pts',(32.1254767797738,8.43974476089548,7.17242748921352));
#59066=CARTESIAN_POINT('Ctrl Pts',(32.0857887388241,9.52799121518563,5.64715779135255));
#59067=CARTESIAN_POINT('Ctrl Pts',(32.0461006978744,10.1851777567691,3.95452364884696));
#59068=CARTESIAN_POINT('Ctrl Pts',(32.0064126569246,10.8423642983526,2.26188950634136));
#59069=CARTESIAN_POINT('Ctrl Pts',(31.9667246159749,11.0684909272294,0.401890919191144));
#59070=CARTESIAN_POINT('Ctrl Pts',(31.9270365750252,10.836012821607,-1.39890291165689));
#59071=CARTESIAN_POINT('Ctrl Pts',(31.8873485340754,10.6035347159847,-3.19969674250482));
#59072=CARTESIAN_POINT('Ctrl Pts',(31.8476604931257,9.91245187586315,-4.94128581705056));
#59073=CARTESIAN_POINT('Ctrl Pts',(31.807972452176,8.84694613232347,-6.41152457361281));
#59074=CARTESIAN_POINT('Ctrl Pts',(31.7682844112262,7.7814403887838,-7.88176333017505));
#59075=CARTESIAN_POINT('Ctrl Pts',(31.7285963702765,6.34151174182597,-9.0806517687538));
#59076=CARTESIAN_POINT('Ctrl Pts',(31.6889083293268,4.7025600467055,-9.86215150123965));
#59077=CARTESIAN_POINT('Ctrl Pts',(31.649220288377,3.06360835158493,-10.6436512337256));
#59078=CARTESIAN_POINT('Ctrl Pts',(31.6095322474273,1.22563360830171,-11.0077622601185));
#59079=CARTESIAN_POINT('Ctrl Pts',(31.5698442064776,-0.587477739453859,
-10.9101316734456));
#59080=CARTESIAN_POINT('Ctrl Pts',(31.5301561655279,-2.40058908720943,-10.8125010867726));
#59081=CARTESIAN_POINT('Ctrl Pts',(31.4904681245781,-4.18883703943733,-10.2531288870338));
#59082=CARTESIAN_POINT('Ctrl Pts',(31.4507800836284,-5.73439244700268,-9.3001530358394));
#59083=CARTESIAN_POINT('Ctrl Pts',(31.4110920426787,-7.27994785456802,-8.34717718464504));
#59084=CARTESIAN_POINT('Ctrl Pts',(31.3714040017289,-8.58281071747081,-7.0005976819952));
#59085=CARTESIAN_POINT('Ctrl Pts',(31.3317159607792,-9.48427736796073,-5.42444338470429));
#59086=CARTESIAN_POINT('Ctrl Pts',(31.2920279198295,-10.3857440184507,-3.84828908741338));
#59087=CARTESIAN_POINT('Ctrl Pts',(31.2523398788798,-10.8858144565277,-2.04255999548141));
#59088=CARTESIAN_POINT('Ctrl Pts',(31.21265183793,-10.9235743565816,-0.227214661733031));
#59089=CARTESIAN_POINT('Ctrl Pts',(31.2109968337418,-10.9251489566688,-0.151514172149763));
#59090=CARTESIAN_POINT('Ctrl Pts',(31.2093418295535,-10.9259196370709,-0.075796960719478));
#59091=CARTESIAN_POINT('Ctrl Pts',(31.2076868253652,-10.9258901478294,-7.91472659100149E-5));
#59092=CARTESIAN_POINT('Ctrl Pts',(30.9923131746348,-10.9249872058682,-0.000280213389727673));
#59093=CARTESIAN_POINT('Ctrl Pts',(31.0015326923022,-10.9254167673285,-0.42218162925807));
#59094=CARTESIAN_POINT('Ctrl Pts',(31.0107522099696,-10.9014420331763,-0.844034516027294));
#59095=CARTESIAN_POINT('Ctrl Pts',(31.019971727637,-10.8526837040672,-1.26300316147548));
#59096=CARTESIAN_POINT('Ctrl Pts',(31.0595734062971,-10.6432463179649,-3.06264846443718));
#59097=CARTESIAN_POINT('Ctrl Pts',(31.0991750849572,-9.97653642366005,-4.80907774827739));
#59098=CARTESIAN_POINT('Ctrl Pts',(31.1387767636172,-8.93342120575284,-6.29046151939811));
#59099=CARTESIAN_POINT('Ctrl Pts',(31.1783784422773,-7.8903059878456,-7.77184529051888));
#59100=CARTESIAN_POINT('Ctrl Pts',(31.2179801209374,-6.47078544633602,-8.98818354892013));
#59101=CARTESIAN_POINT('Ctrl Pts',(31.2575817995975,-4.8470373614766,-9.79194308515285));
#59102=CARTESIAN_POINT('Ctrl Pts',(31.2971834782575,-3.22328927661732,-10.5957026213855));
#59103=CARTESIAN_POINT('Ctrl Pts',(31.3367851569176,-1.39531364840828,-10.9868834354496));
#59104=CARTESIAN_POINT('Ctrl Pts',(31.3763868355777,0.415169035973717,-10.9180380672533));
#59105=CARTESIAN_POINT('Ctrl Pts',(31.4159885142378,2.22565172035571,-10.8491926990569));
#59106=CARTESIAN_POINT('Ctrl Pts',(31.4555901928978,4.01864146091071,-10.3203211486));
#59107=CARTESIAN_POINT('Ctrl Pts',(31.4951918715579,5.57666131065755,-9.39557178635968));
#59108=CARTESIAN_POINT('Ctrl Pts',(31.534793550218,7.13468116040447,-8.47082242411927));
#59109=CARTESIAN_POINT('Ctrl Pts',(31.5743952288781,8.45773111934326,-7.15019525009526));
#59110=CARTESIAN_POINT('Ctrl Pts',(31.6139969075382,9.38533460511235,-5.59387298001155));
#59111=CARTESIAN_POINT('Ctrl Pts',(31.6535985861982,10.3129380908814,-4.03755070992784));
#59112=CARTESIAN_POINT('Ctrl Pts',(31.6932002648583,10.8450951034809,-2.24553334378436));
#59113=CARTESIAN_POINT('Ctrl Pts',(31.7328019435184,10.9172587691628,-0.435179886438303));
#59114=CARTESIAN_POINT('Ctrl Pts',(31.7724036221784,10.9894224348447,1.37517357090765));
#59115=CARTESIAN_POINT('Ctrl Pts',(31.8120053008385,10.6015927536092,3.20386311945626));
#59116=CARTESIAN_POINT('Ctrl Pts',(31.8516069794986,9.80081071688866,4.8290816785537));
#59117=CARTESIAN_POINT('Ctrl Pts',(31.8912086581587,9.00002868016809,6.45430023765115));
#59118=CARTESIAN_POINT('Ctrl Pts',(31.9308103368187,7.78629428796244,7.87604780729748));
#59119=CARTESIAN_POINT('Ctrl Pts',(31.9704120154788,6.30682491920728,8.92187648451203));
#59120=CARTESIAN_POINT('Ctrl Pts',(32.0100136941389,4.82735555045204,9.96770516172665));
#59121=CARTESIAN_POINT('Ctrl Pts',(32.049615372799,3.08215120514753,10.6376149465094));
#59122=CARTESIAN_POINT('Ctrl Pts',(32.089217051459,1.28289280052904,10.8503505302259));
#59123=CARTESIAN_POINT('Ctrl Pts',(32.1288187301191,-0.516365604089548,
11.0630861139424));
#59124=CARTESIAN_POINT('Ctrl Pts',(32.1684204087792,-2.36967806802192,10.8186474965926));
#59125=CARTESIAN_POINT('Ctrl Pts',(32.2080220874393,-4.05225092550314,10.1466833499022));
#59126=CARTESIAN_POINT('Ctrl Pts',(32.2476237660994,-5.73482378298416,9.47471920321183));
#59127=CARTESIAN_POINT('Ctrl Pts',(32.2872254447594,-7.24665703401413,8.37522952718105));
#59128=CARTESIAN_POINT('Ctrl Pts',(32.3268271234195,-8.40437602097965,6.98157462642956));
#59129=CARTESIAN_POINT('Ctrl Pts',(32.3664288020796,-9.56209500794516,5.58791972567807));
#59130=CARTESIAN_POINT('Ctrl Pts',(32.4060304807397,-10.3656997308463,3.90009960020581));
#59131=CARTESIAN_POINT('Ctrl Pts',(32.4456321593997,-10.7177186326722,2.1228348681171));
#59132=CARTESIAN_POINT('Ctrl Pts',(32.4611924978114,-10.856034315872,1.42450990780789));
#59133=CARTESIAN_POINT('Ctrl Pts',(32.4767528362231,-10.9246309937472,0.712375858032335));
#59134=CARTESIAN_POINT('Ctrl Pts',(32.4923131746348,-10.9242412661389,0.000167712051415234));
#59135=CARTESIAN_POINT('Origin',(21.9,0.,0.));
#59136=CARTESIAN_POINT('',(34.2076868253652,-10.9254292740963,0.000242939848954564));
#59137=CARTESIAN_POINT('',(33.9923131746348,-10.9259190602418,3.54640925768045E-5));
#59138=CARTESIAN_POINT('',(21.9,-10.925,-1.33792662806848E-15));
#59139=CARTESIAN_POINT('Ctrl Pts',(34.2076868253652,-10.9254292740963,0.000242939848954564));
#59140=CARTESIAN_POINT('Ctrl Pts',(34.2015428532967,-10.9257010658152,0.281369112382754));
#59141=CARTESIAN_POINT('Ctrl Pts',(34.1953988812283,-10.9150692154409,0.5624747774018));
#59142=CARTESIAN_POINT('Ctrl Pts',(34.1892549091598,-10.8933886655163,0.842725701681572));
#59143=CARTESIAN_POINT('Ctrl Pts',(34.1495668682101,-10.7533394361855,2.65305459560608));
#59144=CARTESIAN_POINT('Ctrl Pts',(34.1098788272603,-10.1522571960055,4.42771741908218));
#59145=CARTESIAN_POINT('Ctrl Pts',(34.0701907863106,-9.16336066879775,5.95053984776211));
#59146=CARTESIAN_POINT('Ctrl Pts',(34.0305027453609,-8.1744641415901,7.47336227644196));
#59147=CARTESIAN_POINT('Ctrl Pts',(33.9908147044112,-6.7977533273548,8.74434431032566));
#59148=CARTESIAN_POINT('Ctrl Pts',(33.9511266634614,-5.20092742289286,9.60866573297642));
#59149=CARTESIAN_POINT('Ctrl Pts',(33.9114386225117,-3.60410151843092,10.4729871556272));
#59150=CARTESIAN_POINT('Ctrl Pts',(33.871750581562,-1.78716052374233,10.930647967045));
#59151=CARTESIAN_POINT('Ctrl Pts',(33.8320625406122,0.0285712697578326,
10.9258998214709));
#59152=CARTESIAN_POINT('Ctrl Pts',(33.7923744996625,1.8443030632581,10.9211516758969));
#59153=CARTESIAN_POINT('Ctrl Pts',(33.7526864587128,3.65882565556995,10.4539945733309));
#59154=CARTESIAN_POINT('Ctrl Pts',(33.712998417763,5.25110934447738,9.58133361691454));
#59155=CARTESIAN_POINT('Ctrl Pts',(33.6733103768133,6.8433930333848,8.7086726604982));
#59156=CARTESIAN_POINT('Ctrl Pts',(33.6336223358636,8.21343781888779,7.43050785023152));
#59157=CARTESIAN_POINT('Ctrl Pts',(33.5939342949138,9.1943565030835,5.90253434725122));
#59158=CARTESIAN_POINT('Ctrl Pts',(33.5542462539641,10.1752751872792,4.37456084427093));
#59159=CARTESIAN_POINT('Ctrl Pts',(33.5145582130144,10.7670677701676,2.59677864857703));
#59160=CARTESIAN_POINT('Ctrl Pts',(33.4748701720647,10.8976471149318,0.785742059897758));
#59161=CARTESIAN_POINT('Ctrl Pts',(33.4351821311149,11.028226459696,-1.02529452878152));
#59162=CARTESIAN_POINT('Ctrl Pts',(33.3954940901652,10.6975925663359,-2.86958551044617));
#59163=CARTESIAN_POINT('Ctrl Pts',(33.3558060492155,9.94602044233928,-4.52247505099183));
#59164=CARTESIAN_POINT('Ctrl Pts',(33.3161180082657,9.19444831834266,-6.1753645915374));
#59165=CARTESIAN_POINT('Ctrl Pts',(33.276429967316,8.0219379637095,-7.636852690964));
#59166=CARTESIAN_POINT('Ctrl Pts',(33.2367419263663,6.57131461281705,-8.72891330496823));
#59167=CARTESIAN_POINT('Ctrl Pts',(33.1970538854166,5.12069126192459,-9.82097391897245));
#59168=CARTESIAN_POINT('Ctrl Pts',(33.1573658444668,3.39195491477284,-10.5436070475543));
#59169=CARTESIAN_POINT('Ctrl Pts',(33.1176778035171,1.5956855231573,-10.8087876719575));
#59170=CARTESIAN_POINT('Ctrl Pts',(33.0779897625674,-0.200583868458334,
-11.0739682963607));
#59171=CARTESIAN_POINT('Ctrl Pts',(33.0383017216176,-2.06438630453777,-10.8816964165853));
#59172=CARTESIAN_POINT('Ctrl Pts',(32.9986136806679,-3.768689231625,-10.2553929569621));
#59173=CARTESIAN_POINT('Ctrl Pts',(32.9589256397182,-5.47299215871224,-9.62908949733891));
#59174=CARTESIAN_POINT('Ctrl Pts',(32.9192375987684,-7.01779557680729,-8.56875445786798));
#59175=CARTESIAN_POINT('Ctrl Pts',(32.8795495578187,-8.21492467842605,-7.20354883054602));
#59176=CARTESIAN_POINT('Ctrl Pts',(32.839861516869,-9.41205378004481,-5.83834320322405));
#59177=CARTESIAN_POINT('Ctrl Pts',(32.8001734759192,-10.2615085651873,-4.16826698805105));
#59178=CARTESIAN_POINT('Ctrl Pts',(32.7604854349695,-10.6598156800349,-2.39675465869067));
#59179=CARTESIAN_POINT('Ctrl Pts',(32.7428858984347,-10.8364437133686,-1.6111831057423));
#59180=CARTESIAN_POINT('Ctrl Pts',(32.7252863619,-10.9243557660912,-0.805664637555209));
#59181=CARTESIAN_POINT('Ctrl Pts',(32.7076868253652,-10.9241131192016,-9.40179992833195E-5));
#59182=CARTESIAN_POINT('Ctrl Pts',(32.4923131746348,-10.9242412661389,0.000167712051415234));
#59183=CARTESIAN_POINT('Ctrl Pts',(32.5163545148832,-10.9236391215206,-1.1002221324473));
#59184=CARTESIAN_POINT('Ctrl Pts',(32.5403958551316,-10.7583562441758,-2.20078885552534));
#59185=CARTESIAN_POINT('Ctrl Pts',(32.56443719538,-10.4310946365082,-3.25087453627992));
#59186=CARTESIAN_POINT('Ctrl Pts',(32.60403887404,-9.89201865776741,-4.98060986988279));
#59187=CARTESIAN_POINT('Ctrl Pts',(32.6436405527001,-8.91343361953511,-6.57337119838318));
#59188=CARTESIAN_POINT('Ctrl Pts',(32.6832422313602,-7.61403495082711,-7.83596786198144));
#59189=CARTESIAN_POINT('Ctrl Pts',(32.7228439100203,-6.31463628211919,-9.09856452557962));
#59190=CARTESIAN_POINT('Ctrl Pts',(32.7624455886804,-4.69442398293564,-10.0309965242757));
#59191=CARTESIAN_POINT('Ctrl Pts',(32.8020472673404,-2.94991832124996,-10.520166465621));
#59192=CARTESIAN_POINT('Ctrl Pts',(32.8416489460005,-1.20541265956428,-11.0093364069663));
#59193=CARTESIAN_POINT('Ctrl Pts',(32.8812506246606,0.663386364623482,-11.0552442909609));
#59194=CARTESIAN_POINT('Ctrl Pts',(32.9208523033206,2.42980667555691,-10.6523218166671));
#59195=CARTESIAN_POINT('Ctrl Pts',(32.9604539819807,4.19622698649044,-10.2493993423733));
#59196=CARTESIAN_POINT('Ctrl Pts',(33.0000556606408,5.86026858416957,-9.39764650979103));
#59197=CARTESIAN_POINT('Ctrl Pts',(33.0396573393009,7.22009501737135,-8.20037490036596));
#59198=CARTESIAN_POINT('Ctrl Pts',(33.079259017961,8.57992145057314,-7.0031032909409));
#59199=CARTESIAN_POINT('Ctrl Pts',(33.118860696621,9.63553271929753,-5.46031290467306));
#59200=CARTESIAN_POINT('Ctrl Pts',(33.1584623752811,10.2588906587249,-3.75913328025875));
#59201=CARTESIAN_POINT('Ctrl Pts',(33.1980640539412,10.8822485981523,-2.05795365584465));
#59202=CARTESIAN_POINT('Ctrl Pts',(33.2376657326012,11.0733532082827,-0.198384793283873));
#59203=CARTESIAN_POINT('Ctrl Pts',(33.2772674112613,10.8090248544395,1.59402078484943));
#59204=CARTESIAN_POINT('Ctrl Pts',(33.3168690899214,10.5446965005963,3.38642636298283));
#59205=CARTESIAN_POINT('Ctrl Pts',(33.3564707685815,9.82493518277935,5.11166865668897));
#59206=CARTESIAN_POINT('Ctrl Pts',(33.3960724472416,8.7370428472372,6.56048800410184));
#59207=CARTESIAN_POINT('Ctrl Pts',(33.4356741259016,7.64915051169498,8.00930735151479));
#59208=CARTESIAN_POINT('Ctrl Pts',(33.4752758045617,6.19312715842752,9.18170375263436));
#59209=CARTESIAN_POINT('Ctrl Pts',(33.5148774832218,4.545578100025,9.93547383384385));
#59210=CARTESIAN_POINT('Ctrl Pts',(33.5544791618819,2.89802904162249,10.6892439150533));
#59211=CARTESIAN_POINT('Ctrl Pts',(33.5940808405419,1.05895427808499,11.0243876763527));
#59212=CARTESIAN_POINT('Ctrl Pts',(33.633682519202,-0.748579456965083,10.9002545549649));
#59213=CARTESIAN_POINT('Ctrl Pts',(33.6732841978621,-2.55611319201506,10.776121433577));
#59214=CARTESIAN_POINT('Ctrl Pts',(33.7128858765222,-4.33210589857755,10.192711429502));
#59215=CARTESIAN_POINT('Ctrl Pts',(33.7524875551822,-5.86114224942137,9.2207880410771));
#59216=CARTESIAN_POINT('Ctrl Pts',(33.7920892338423,-7.39017860026528,8.24886465265211));
#59217=CARTESIAN_POINT('Ctrl Pts',(33.8316909125024,-8.67225859539043,6.88842787987717));
#59218=CARTESIAN_POINT('Ctrl Pts',(33.8712925911625,-9.55187501865457,5.30448906063775));
#59219=CARTESIAN_POINT('Ctrl Pts',(33.9108942698226,-10.4314914419187,3.72055024139843));
#59220=CARTESIAN_POINT('Ctrl Pts',(33.9504959484826,-10.9086442933217,1.91310937569469));
#59221=CARTESIAN_POINT('Ctrl Pts',(33.9900976271427,-10.9254583140047,0.101396229559884));
#59222=CARTESIAN_POINT('Ctrl Pts',(33.9908361429734,-10.9257718719364,0.067610317336041));
#59223=CARTESIAN_POINT('Ctrl Pts',(33.9915746588041,-10.9259253377178,0.0338229193401644));
#59224=CARTESIAN_POINT('Ctrl Pts',(33.9923131746348,-10.9259190602418,3.54640925768045E-5));
#59225=CARTESIAN_POINT('Origin',(21.9,0.,0.));
#59226=CARTESIAN_POINT('',(35.7076868253652,-10.924906646948,-0.000283429730867565));
#59227=CARTESIAN_POINT('',(35.4923131746348,-10.9243725253197,-0.000213636941074988));
#59228=CARTESIAN_POINT('',(21.9,-10.925,-1.33792662806848E-15));
#59229=CARTESIAN_POINT('Ctrl Pts',(35.7076868253652,-10.924906646948,-0.000283429730867565));
#59230=CARTESIAN_POINT('Ctrl Pts',(35.6777993446935,-10.9235234982586,1.3674492491528));
#59231=CARTESIAN_POINT('Ctrl Pts',(35.6479118640218,-10.6659170279025,2.73568824768952));
#59232=CARTESIAN_POINT('Ctrl Pts',(35.6180243833501,-10.164356412782,4.00773775841331));
#59233=CARTESIAN_POINT('Ctrl Pts',(35.5783363424004,-9.49832643018392,5.69691168465494));
#59234=CARTESIAN_POINT('Ctrl Pts',(35.5386483014506,-8.40211774156364,7.21646902397496));
#59235=CARTESIAN_POINT('Ctrl Pts',(35.4989602605009,-7.00926116160424,8.38131023138392));
#59236=CARTESIAN_POINT('Ctrl Pts',(35.4592722195512,-5.61640458164493,9.54615143879281));
#59237=CARTESIAN_POINT('Ctrl Pts',(35.4195841786014,-3.92690011034658,10.3562765142906));
#59238=CARTESIAN_POINT('Ctrl Pts',(35.3798961376517,-2.14654880621671,10.7130029146269));
#59239=CARTESIAN_POINT('Ctrl Pts',(35.340208096702,-0.366197502086839,11.0697293149631));
#59240=CARTESIAN_POINT('Ctrl Pts',(35.3005200557523,1.50500063487449,10.9730570401377));
#59241=CARTESIAN_POINT('Ctrl Pts',(35.2608320148025,3.23911216986083,10.4347618840745));
#59242=CARTESIAN_POINT('Ctrl Pts',(35.2211439738528,4.97322370484726,9.89646672801125));
#59243=CARTESIAN_POINT('Ctrl Pts',(35.1814559329031,6.57024863785862,8.91654869071018));
#59244=CARTESIAN_POINT('Ctrl Pts',(35.1417678919533,7.83565098082257,7.61437304924106));
#59245=CARTESIAN_POINT('Ctrl Pts',(35.1020798510036,9.10105332378652,6.31219740777195));
#59246=CARTESIAN_POINT('Ctrl Pts',(35.0623918100539,10.034833076703,4.68776416213484));
#59247=CARTESIAN_POINT('Ctrl Pts',(35.0227037691042,10.5232451357101,2.93894794782568));
#59248=CARTESIAN_POINT('Ctrl Pts',(34.9830157281544,11.0116571947171,1.19013173351651));
#59249=CARTESIAN_POINT('Ctrl Pts',(34.9433276872047,11.0547015598147,-0.683067449464948));
#59250=CARTESIAN_POINT('Ctrl Pts',(34.9036396462549,10.647134932716,-2.45247241591259));
#59251=CARTESIAN_POINT('Ctrl Pts',(34.8639516053052,10.2395683056174,-4.22187738236013));
#59252=CARTESIAN_POINT('Ctrl Pts',(34.8242635643555,9.38139068632257,-5.88748813227409));
#59253=CARTESIAN_POINT('Ctrl Pts',(34.7845755234058,8.17713797008293,-7.24641413697163));
#59254=CARTESIAN_POINT('Ctrl Pts',(34.744887482456,6.97288525384329,-8.60534014166917));
#59255=CARTESIAN_POINT('Ctrl Pts',(34.7051994415063,5.42255744065888,-9.65758140115024));
#59256=CARTESIAN_POINT('Ctrl Pts',(34.6655114005566,3.71500227281579,-10.2749628388256));
#59257=CARTESIAN_POINT('Ctrl Pts',(34.6258233596068,2.0074471049727,-10.892344276501));
#59258=CARTESIAN_POINT('Ctrl Pts',(34.5861353186571,0.142664582471003,-11.0748658923707));
#59259=CARTESIAN_POINT('Ctrl Pts',(34.5464472777074,-1.65219335544512,-10.8002944562867));
#59260=CARTESIAN_POINT('Ctrl Pts',(34.5067592367577,-3.44705129336145,-10.5257230202026));
#59261=CARTESIAN_POINT('Ctrl Pts',(34.4670711958079,-5.17198464669214,-9.79405853216478));
#59262=CARTESIAN_POINT('Ctrl Pts',(34.4273831548582,-6.61687671198883,-8.69442613428939));
#59263=CARTESIAN_POINT('Ctrl Pts',(34.3876951139085,-8.06176877728535,-7.59479373641412));
#59264=CARTESIAN_POINT('Ctrl Pts',(34.3480070729587,-9.22661955454791,-6.12719342870145));
#59265=CARTESIAN_POINT('Ctrl Pts',(34.308319032009,-9.96953683393836,-4.4703957926587));
#59266=CARTESIAN_POINT('Ctrl Pts',(34.2747749631277,-10.5974455892362,-3.07008142349836));
#59267=CARTESIAN_POINT('Ctrl Pts',(34.2412308942465,-10.9239453806084,-1.53461359769846));
#59268=CARTESIAN_POINT('Ctrl Pts',(34.2076868253652,-10.9254292740963,0.000242939848954564));
#59269=CARTESIAN_POINT('Ctrl Pts',(33.9923131746348,-10.9259190602418,3.54640925768045E-5));
#59270=CARTESIAN_POINT('Ctrl Pts',(34.0311763374642,-10.9255887185459,-1.77797296886743));
#59271=CARTESIAN_POINT('Ctrl Pts',(34.0700395002936,-10.4828949617276,-3.55613994411971));
#59272=CARTESIAN_POINT('Ctrl Pts',(34.1089026631229,-9.64868029968667,-5.12629388943526));
#59273=CARTESIAN_POINT('Ctrl Pts',(34.148504341783,-8.79861307472322,-6.72628543572909));
#59274=CARTESIAN_POINT('Ctrl Pts',(34.1881060204431,-7.54200343483366,-8.11028310175106));
#59275=CARTESIAN_POINT('Ctrl Pts',(34.2277076991032,-6.03126922260175,-9.11041778026231));
#59276=CARTESIAN_POINT('Ctrl Pts',(34.2673093777632,-4.52053501036975,-10.1105524587736));
#59277=CARTESIAN_POINT('Ctrl Pts',(34.3069110564233,-2.75567622579537,-10.7268241497742));
#59278=CARTESIAN_POINT('Ctrl Pts',(34.3465127350834,-0.950757730288914,
-10.8844834652233));
#59279=CARTESIAN_POINT('Ctrl Pts',(34.3861144137435,0.854160765217641,-11.0421427806724));
#59280=CARTESIAN_POINT('Ctrl Pts',(34.4257160924035,2.69913897165627,-10.74118972057));
#59281=CARTESIAN_POINT('Ctrl Pts',(34.4653177710636,4.36039410962366,-10.0181277579786));
#59282=CARTESIAN_POINT('Ctrl Pts',(34.5049194497237,6.02164924759105,-9.29506579538727));
#59283=CARTESIAN_POINT('Ctrl Pts',(34.5445211283838,7.49918131708721,-8.14989493030692));
#59284=CARTESIAN_POINT('Ctrl Pts',(34.5841228070438,8.61377615069515,-6.72151627180491));
#59285=CARTESIAN_POINT('Ctrl Pts',(34.6237244857039,9.72837098430303,-5.29313761330298));
#59286=CARTESIAN_POINT('Ctrl Pts',(34.663326164364,10.4800285820227,-3.58155116137942));
#59287=CARTESIAN_POINT('Ctrl Pts',(34.7029278430241,10.7775782049316,-1.79436022108346));
#59288=CARTESIAN_POINT('Ctrl Pts',(34.7425295216841,11.0751278278404,-0.00716928078749735));
#59289=CARTESIAN_POINT('Ctrl Pts',(34.7821312003442,10.9185694759384,1.85562614788087));
#59290=CARTESIAN_POINT('Ctrl Pts',(34.8217328790043,10.3268925676398,3.56808218274874));
#59291=CARTESIAN_POINT('Ctrl Pts',(34.8613345576644,9.73521565934121,5.28053821761661));
#59292=CARTESIAN_POINT('Ctrl Pts',(34.9009362363244,8.70842019464612,6.84265485868399));
#59293=CARTESIAN_POINT('Ctrl Pts',(34.9405379149845,7.37104918558915,8.06495842953008));
#59294=CARTESIAN_POINT('Ctrl Pts',(34.9801395936446,6.03367817653203,9.28726200037632));
#59295=CARTESIAN_POINT('Ctrl Pts',(35.0197412723047,4.38573162311296,10.1697525010012));
#59296=CARTESIAN_POINT('Ctrl Pts',(35.0593429509648,2.62709376176644,10.6053900886913));
#59297=CARTESIAN_POINT('Ctrl Pts',(35.0989446296248,0.868455900420114,11.0410276763813));
#59298=CARTESIAN_POINT('Ctrl Pts',(35.1385463082849,-1.00087326885364,11.0298123511366));
#59299=CARTESIAN_POINT('Ctrl Pts',(35.178147986945,-2.75415736745706,10.5731044524163));
#59300=CARTESIAN_POINT('Ctrl Pts',(35.217749665605,-4.50744146606047,10.1163965536959));
#59301=CARTESIAN_POINT('Ctrl Pts',(35.2573513442651,-6.14468049399354,9.21419608149985));
#59302=CARTESIAN_POINT('Ctrl Pts',(35.2969530229252,-7.46728896176932,7.97593355839057));
#59303=CARTESIAN_POINT('Ctrl Pts',(35.3365547015853,-8.78989742954518,6.73767103528122));
#59304=CARTESIAN_POINT('Ctrl Pts',(35.3761563802453,-9.7978753371637,5.1633464612586));
#59305=CARTESIAN_POINT('Ctrl Pts',(35.4157580589054,-10.3689621088865,3.44391424848231));
#59306=CARTESIAN_POINT('Ctrl Pts',(35.4412764308152,-10.7369567274651,2.3359533699566));
#59307=CARTESIAN_POINT('Ctrl Pts',(35.466794802725,-10.9235452121697,1.16774083242684));
#59308=CARTESIAN_POINT('Ctrl Pts',(35.4923131746348,-10.9243725253197,-0.000213636941074988));
#59309=CARTESIAN_POINT('Origin',(21.9,0.,0.));
#59310=CARTESIAN_POINT('',(37.2076868253652,-10.9243842806946,0.000220727624482799));
#59311=CARTESIAN_POINT('',(36.9923131746348,-10.9247798688888,0.000275851758545804));
#59312=CARTESIAN_POINT('',(21.9,-10.925,-1.33792662806848E-15));
#59313=CARTESIAN_POINT('Ctrl Pts',(37.2076868253652,-10.9243842806946,0.000220727624482799));
#59314=CARTESIAN_POINT('Ctrl Pts',(37.19374387704,-10.9248503212398,0.638375672713467));
#59315=CARTESIAN_POINT('Ctrl Pts',(37.1798009287148,-10.8698520517992,1.27645119149048));
#59316=CARTESIAN_POINT('Ctrl Pts',(37.1658579803896,-10.7586562859676,1.90457820702777));
#59317=CARTESIAN_POINT('Ctrl Pts',(37.1261699394398,-10.4421420161852,3.69251646318714));
#59318=CARTESIAN_POINT('Ctrl Pts',(37.0864818984901,-9.6702969166205,5.39984863320152));
#59319=CARTESIAN_POINT('Ctrl Pts',(37.0467938575404,-8.53714058958459,6.81860204000362));
#59320=CARTESIAN_POINT('Ctrl Pts',(37.0071058165907,-7.40398426254868,8.23735544680572));
#59321=CARTESIAN_POINT('Ctrl Pts',(36.967417775641,-5.90951670804152,9.36753009039557));
#59322=CARTESIAN_POINT('Ctrl Pts',(36.9277297346912,-4.23578124695858,10.0714577124758));
#59323=CARTESIAN_POINT('Ctrl Pts',(36.8880416937415,-2.56204578587573,10.775385334556));
#59324=CARTESIAN_POINT('Ctrl Pts',(36.8483536527917,-0.709042418217058,
11.0530659351266));
#59325=CARTESIAN_POINT('Ctrl Pts',(36.808665611842,1.09751175318593,10.8706748262421));
#59326=CARTESIAN_POINT('Ctrl Pts',(36.7689775708923,2.90406592458893,10.6882837173575));
#59327=CARTESIAN_POINT('Ctrl Pts',(36.7292895299426,4.6641708997363,10.0458208990177));
#59328=CARTESIAN_POINT('Ctrl Pts',(36.6896014889928,6.16342566748929,9.02154572496358));
#59329=CARTESIAN_POINT('Ctrl Pts',(36.6499134480431,7.66268043524244,7.99727055090932));
#59330=CARTESIAN_POINT('Ctrl Pts',(36.6102254070934,8.9010849956012,6.59118302114059));
#59331=CARTESIAN_POINT('Ctrl Pts',(36.5705373661436,9.72778744274805,4.97456075397493));
#59332=CARTESIAN_POINT('Ctrl Pts',(36.5308493251939,10.5544898898948,3.35793848680945));
#59333=CARTESIAN_POINT('Ctrl Pts',(36.4911612842442,10.9694902238298,1.53078148224705));
#59334=CARTESIAN_POINT('Ctrl Pts',(36.4514732432944,10.9222366351582,-0.284341540903556));
#59335=CARTESIAN_POINT('Ctrl Pts',(36.4117852023447,10.8749830464865,-2.09946456405426));
#59336=CARTESIAN_POINT('Ctrl Pts',(36.372097161395,10.3654755352083,-3.90255360579289));
#59337=CARTESIAN_POINT('Ctrl Pts',(36.3324091204453,9.45577797088979,-5.47397170174542));
#59338=CARTESIAN_POINT('Ctrl Pts',(36.2927210794955,8.54608040657125,-7.04538979769804));
#59339=CARTESIAN_POINT('Ctrl Pts',(36.2530330385458,7.23619278921244,-8.38513694786428));
#59340=CARTESIAN_POINT('Ctrl Pts',(36.2133449975961,5.68567448237713,-9.33001655447191));
#59341=CARTESIAN_POINT('Ctrl Pts',(36.1736569566463,4.13515617554199,-10.2748961610794));
#59342=CARTESIAN_POINT('Ctrl Pts',(36.1339689156966,2.34400717923035,-10.8249082241285));
#59343=CARTESIAN_POINT('Ctrl Pts',(36.0942808747469,0.530410023082115,-10.9130549542137));
#59344=CARTESIAN_POINT('Ctrl Pts',(36.0545928337971,-1.28318713306612,-11.0012016842989));
#59345=CARTESIAN_POINT('Ctrl Pts',(36.0149047928474,-3.11923244905102,-10.6274830814203));
#59346=CARTESIAN_POINT('Ctrl Pts',(35.9752167518977,-4.754074507598,-9.83742236576641));
#59347=CARTESIAN_POINT('Ctrl Pts',(35.935528710948,-6.38891656614507,-9.04736165011245));
#59348=CARTESIAN_POINT('Ctrl Pts',(35.8958406699982,-7.82255536725425,-7.84095882168311));
#59349=CARTESIAN_POINT('Ctrl Pts',(35.8561526290485,-8.88035723117022,-6.3651676076186));
#59350=CARTESIAN_POINT('Ctrl Pts',(35.8164645880988,-9.93815909508618,-4.8893763935541));
#59351=CARTESIAN_POINT('Ctrl Pts',(35.776776547149,-10.620124021809,-3.14419679385439));
#59352=CARTESIAN_POINT('Ctrl Pts',(35.7370885061993,-10.8431808468824,-1.34221173742295));
#59353=CARTESIAN_POINT('Ctrl Pts',(35.7272879459213,-10.8982624736709,-0.897229754360836));
#59354=CARTESIAN_POINT('Ctrl Pts',(35.7174873856432,-10.9253602024769,-0.448783813917448));
#59355=CARTESIAN_POINT('Ctrl Pts',(35.7076868253652,-10.924906646948,-0.000283429730867565));
#59356=CARTESIAN_POINT('Ctrl Pts',(35.4923131746348,-10.9243725253197,-0.000213636941074988));
#59357=CARTESIAN_POINT('Ctrl Pts',(35.5063964813851,-10.9248291102817,-0.644794769335064));
#59358=CARTESIAN_POINT('Ctrl Pts',(35.5204797881354,-10.8687063009618,-1.28929729897177));
#59359=CARTESIAN_POINT('Ctrl Pts',(35.5345630948857,-10.7552720369082,-1.92354983780591));
#59360=CARTESIAN_POINT('Ctrl Pts',(35.5741647735457,-10.4362995573802,-3.70704185978775));
#59361=CARTESIAN_POINT('Ctrl Pts',(35.6137664522058,-9.66415896249705,-5.40948605222157));
#59362=CARTESIAN_POINT('Ctrl Pts',(35.6533681308659,-8.53250543355592,-6.82438800133473));
#59363=CARTESIAN_POINT('Ctrl Pts',(35.6929698095259,-7.40085190461478,-8.23928995044789));
#59364=CARTESIAN_POINT('Ctrl Pts',(35.732571488186,-5.90968544161561,-9.3666496562404));
#59365=CARTESIAN_POINT('Ctrl Pts',(35.7721731668461,-4.23987396726792,-10.0697263770227));
#59366=CARTESIAN_POINT('Ctrl Pts',(35.8117748455062,-2.57006249292015,-10.772803097805));
#59367=CARTESIAN_POINT('Ctrl Pts',(35.8513765241663,-0.721606007223839,
-11.0515968335771));
#59368=CARTESIAN_POINT('Ctrl Pts',(35.8909782028264,1.08129081979746,-10.8722918802543));
#59369=CARTESIAN_POINT('Ctrl Pts',(35.9305798814864,2.88418764681875,-10.6929869269316));
#59370=CARTESIAN_POINT('Ctrl Pts',(35.9701815601465,4.64152481516504,-10.0555832845141));
#59371=CARTESIAN_POINT('Ctrl Pts',(36.0097832388066,6.14014978216192,-9.03739349696801));
#59372=CARTESIAN_POINT('Ctrl Pts',(36.0493849174666,7.6387747491587,-8.01920370942198));
#59373=CARTESIAN_POINT('Ctrl Pts',(36.0889865961267,8.87868751480611,-6.62022777674742));
#59374=CARTESIAN_POINT('Ctrl Pts',(36.1285882747868,9.70949544902,-5.01015156376358));
#59375=CARTESIAN_POINT('Ctrl Pts',(36.1681899534469,10.5403033832339,-3.40007535077974));
#59376=CARTESIAN_POINT('Ctrl Pts',(36.2077916321069,10.9620064860143,-1.57889885748661));
#59377=CARTESIAN_POINT('Ctrl Pts',(36.247393310767,10.9234551599872,0.232482115812686));
#59378=CARTESIAN_POINT('Ctrl Pts',(36.2869949894271,10.88490383396,2.04386308911198));
#59379=CARTESIAN_POINT('Ctrl Pts',(36.3265966680872,10.3860980791254,3.84544854241745));
#59380=CARTESIAN_POINT('Ctrl Pts',(36.3661983467473,9.48753949805479,5.41871892971697));
#59381=CARTESIAN_POINT('Ctrl Pts',(36.4058000254073,8.58898091698422,6.9919893170165));
#59382=CARTESIAN_POINT('Ctrl Pts',(36.4454017040674,7.29066950967774,8.33694463831008));
#59383=CARTESIAN_POINT('Ctrl Pts',(36.4850033827274,5.75008124752846,9.2904513460458));
#59384=CARTESIAN_POINT('Ctrl Pts',(36.5246050613875,4.20949298537909,10.2439580537816));
#59385=CARTESIAN_POINT('Ctrl Pts',(36.5642067400476,2.42662786838689,10.8060161479594));
#59386=CARTESIAN_POINT('Ctrl Pts',(36.6038084187077,0.617734798457242,10.9084519655723));
#59387=CARTESIAN_POINT('Ctrl Pts',(36.6434100973678,-1.19115827147241,11.0108877831851));
#59388=CARTESIAN_POINT('Ctrl Pts',(36.6830117760279,-3.02607929433952,10.6537013242329));
#59389=CARTESIAN_POINT('Ctrl Pts',(36.7226134546879,-4.66446535582359,9.88021677448143));
#59390=CARTESIAN_POINT('Ctrl Pts',(36.762215133348,-6.30285141730757,9.10673222473001));
#59391=CARTESIAN_POINT('Ctrl Pts',(36.8018168120081,-7.74470251740853,7.91694958417936));
#59392=CARTESIAN_POINT('Ctrl Pts',(36.8414184906681,-8.81513233739371,6.45518105405715));
#59393=CARTESIAN_POINT('Ctrl Pts',(36.8810201693282,-9.88556215737889,4.99341252393494));
#59394=CARTESIAN_POINT('Ctrl Pts',(36.9206218479883,-10.5845706972483,3.25965810424116));
#59395=CARTESIAN_POINT('Ctrl Pts',(36.9602235266484,-10.8273731756247,1.46420991739102));
#59396=CARTESIAN_POINT('Ctrl Pts',(36.9709200759772,-10.8929549583921,0.979253199701995));
#59397=CARTESIAN_POINT('Ctrl Pts',(36.981616625306,-10.9252538337305,0.489795559919792));
#59398=CARTESIAN_POINT('Ctrl Pts',(36.9923131746348,-10.9247798688888,0.000275851758545804));
#59399=CARTESIAN_POINT('Origin',(21.9,0.,0.));
#59400=CARTESIAN_POINT('',(38.7076868253652,-10.9258695923078,-9.50230565660546E-5));
#59401=CARTESIAN_POINT('',(38.4923131746348,-10.9256735326657,-0.000180534162333964));
#59402=CARTESIAN_POINT('',(21.9,-10.925,-1.33792662806848E-15));
#59403=CARTESIAN_POINT('Ctrl Pts',(38.7076868253652,-10.9258695923078,-9.50230565660546E-5));
#59404=CARTESIAN_POINT('Ctrl Pts',(38.6700003684368,-10.9250797367911,1.72410105657515));
#59405=CARTESIAN_POINT('Ctrl Pts',(38.6323139115083,-10.5097841860533,3.44866417786596));
#59406=CARTESIAN_POINT('Ctrl Pts',(38.5946274545799,-9.72343224897335,4.98306818395048));
#59407=CARTESIAN_POINT('Ctrl Pts',(38.5549394136302,-8.8953159859084,6.5989666788014));
#59408=CARTESIAN_POINT('Ctrl Pts',(38.5152513726804,-7.65568193134823,8.00397038244873));
#59409=CARTESIAN_POINT('Ctrl Pts',(38.4755633317307,-6.15553175763203,9.02693369905073));
#59410=CARTESIAN_POINT('Ctrl Pts',(38.435875290781,-4.65538158391583,10.0498970156527));
#59411=CARTESIAN_POINT('Ctrl Pts',(38.3961872498312,-2.89471529104359,10.6908199452094));
#59412=CARTESIAN_POINT('Ctrl Pts',(38.3564992088815,-1.08800226510296,10.8716307101283));
#59413=CARTESIAN_POINT('Ctrl Pts',(38.3168111679318,0.718710760837562,11.0524414750472));
#59414=CARTESIAN_POINT('Ctrl Pts',(38.277123126982,2.57147051984646,10.7731400753285));
#59415=CARTESIAN_POINT('Ctrl Pts',(38.2374350860323,4.24458958342512,10.0677486308784));
#59416=CARTESIAN_POINT('Ctrl Pts',(38.1977470450826,5.91770864700377,9.36235718642825));
#59417=CARTESIAN_POINT('Ctrl Pts',(38.1580590041329,7.41118701515218,8.23087569724678));
#59418=CARTESIAN_POINT('Ctrl Pts',(38.1183709631831,8.54310186124007,6.81113161044115));
#59419=CARTESIAN_POINT('Ctrl Pts',(38.0786829222334,9.67501670732803,5.39138752363544));
#59420=CARTESIAN_POINT('Ctrl Pts',(38.0389948812837,10.4453680313554,3.68338083920554));
#59421=CARTESIAN_POINT('Ctrl Pts',(37.9993068403339,10.7603181900364,1.89516639782527));
#59422=CARTESIAN_POINT('Ctrl Pts',(37.9596187993842,11.0752683487174,0.106951956445004));
#59423=CARTESIAN_POINT('Ctrl Pts',(37.9199307584345,10.9348173420519,-1.76147024188562));
#59424=CARTESIAN_POINT('Ctrl Pts',(37.8802427174847,10.3560737165584,-3.48250490358328));
#59425=CARTESIAN_POINT('Ctrl Pts',(37.840554676535,9.77733009106496,-5.20353956528093));
#59426=CARTESIAN_POINT('Ctrl Pts',(37.8008666355853,8.76029384674342,-6.77718669034561));
#59427=CARTESIAN_POINT('Ctrl Pts',(37.7611785946356,7.42885168479985,-8.01175797634456));
#59428=CARTESIAN_POINT('Ctrl Pts',(37.7214905536858,6.09740952285627,-9.24632926234352));
#59429=CARTESIAN_POINT('Ctrl Pts',(37.6818025127361,4.45156144329064,-10.1418247092768));
#59430=CARTESIAN_POINT('Ctrl Pts',(37.6421144717864,2.69179065444689,-10.5891626816716));
#59431=CARTESIAN_POINT('Ctrl Pts',(37.6024264308366,0.932019865603235,-11.0365006540664));
#59432=CARTESIAN_POINT('Ctrl Pts',(37.5627383898869,-0.941673632518532,
-11.0356811519229));
#59433=CARTESIAN_POINT('Ctrl Pts',(37.5230503489372,-2.70105244144865,-10.586804000019));
#59434=CARTESIAN_POINT('Ctrl Pts',(37.4833623079875,-4.46043125037876,-10.1379268481151));
#59435=CARTESIAN_POINT('Ctrl Pts',(37.4436742670377,-6.10549537011722,-9.24099204645071));
#59436=CARTESIAN_POINT('Ctrl Pts',(37.403986226088,-7.43585708763547,-8.00525656044425));
#59437=CARTESIAN_POINT('Ctrl Pts',(37.3642981851382,-8.76621880515379,-6.76952107443772));
#59438=CARTESIAN_POINT('Ctrl Pts',(37.3246101441885,-9.78187812045187,-5.19498490408906));
#59439=CARTESIAN_POINT('Ctrl Pts',(37.2849221032388,-10.3591160581009,-3.47344464776253));
#59440=CARTESIAN_POINT('Ctrl Pts',(37.2591770106143,-10.7335624609856,-2.3567048869836));
#59441=CARTESIAN_POINT('Ctrl Pts',(37.2334319179897,-10.9235237555946,-1.17810668110777));
#59442=CARTESIAN_POINT('Ctrl Pts',(37.2076868253652,-10.9243842806946,0.000220727624482799));
#59443=CARTESIAN_POINT('Ctrl Pts',(36.9923131746348,-10.9247798688888,0.000275851758545804));
#59444=CARTESIAN_POINT('Ctrl Pts',(37.0212183039661,-10.923499080606,-1.32254612004258));
#59445=CARTESIAN_POINT('Ctrl Pts',(37.0501234332973,-10.6828996572383,-2.64582133665475));
#59446=CARTESIAN_POINT('Ctrl Pts',(37.0790285626286,-10.2130467683216,-3.88195778886101));
#59447=CARTESIAN_POINT('Ctrl Pts',(37.1186302412887,-9.56932146575876,-5.57553535425621));
#59448=CARTESIAN_POINT('Ctrl Pts',(37.1582319199488,-8.49527444374974,-7.10554853104));
#59449=CARTESIAN_POINT('Ctrl Pts',(37.1978335986089,-7.12117999331664,-8.28641756546274));
#59450=CARTESIAN_POINT('Ctrl Pts',(37.2374352772689,-5.74708554288363,-9.46728659988541));
#59451=CARTESIAN_POINT('Ctrl Pts',(37.277036955929,-4.07294366402656,-10.2990114919471));
#59452=CARTESIAN_POINT('Ctrl Pts',(37.316638634589,-2.30181590048543,-10.680709907431));
#59453=CARTESIAN_POINT('Ctrl Pts',(37.3562403132491,-0.530688136944307,
-11.062408322915));
#59454=CARTESIAN_POINT('Ctrl Pts',(37.3958419919092,1.33742551128088,-10.9940802618212));
#59455=CARTESIAN_POINT('Ctrl Pts',(37.4354436705693,3.07593609968004,-10.4840134336574));
#59456=CARTESIAN_POINT('Ctrl Pts',(37.4750453492294,4.81444668807931,-9.97394660549346));
#59457=CARTESIAN_POINT('Ctrl Pts',(37.5146470278894,6.42335421665253,-9.02214101025939));
#59458=CARTESIAN_POINT('Ctrl Pts',(37.5542487065495,7.707509605974,-7.74404392034558));
#59459=CARTESIAN_POINT('Ctrl Pts',(37.5938503852096,8.99166499529546,-6.46594683043176));
#59460=CARTESIAN_POINT('Ctrl Pts',(37.6334520638697,9.95106824536517,-4.86155824583819));
#59461=CARTESIAN_POINT('Ctrl Pts',(37.6730537425298,10.4693505421126,-3.12547913011572));
#59462=CARTESIAN_POINT('Ctrl Pts',(37.7126554211898,10.98763283886,-1.38940001439336));
#59463=CARTESIAN_POINT('Ctrl Pts',(37.7522570998499,11.0647941822853,0.478369632457899));
#59464=CARTESIAN_POINT('Ctrl Pts',(37.79185877851,10.6914754483434,2.25128259085636));
#59465=CARTESIAN_POINT('Ctrl Pts',(37.83146045717,10.3181567144015,4.02419554925483));
#59466=CARTESIAN_POINT('Ctrl Pts',(37.8710621358301,9.49435790309258,5.70225181920051));
#59467=CARTESIAN_POINT('Ctrl Pts',(37.9106638144902,8.31999997121725,7.0819150690592));
#59468=CARTESIAN_POINT('Ctrl Pts',(37.9502654931503,7.14564203934185,8.46157831891798));
#59469=CARTESIAN_POINT('Ctrl Pts',(37.9898671718103,5.62072498690005,9.54284854868973));
#59470=CARTESIAN_POINT('Ctrl Pts',(38.0294688504704,3.93021044387967,10.1945753434482));
#59471=CARTESIAN_POINT('Ctrl Pts',(38.0690705291305,2.23969590085929,10.8463021382067));
#59472=CARTESIAN_POINT('Ctrl Pts',(38.1086722077906,0.383583867260352,11.0684854979518));
#59473=CARTESIAN_POINT('Ctrl Pts',(38.1482738864507,-1.41299242319487,10.8341761559621));
#59474=CARTESIAN_POINT('Ctrl Pts',(38.1878755651108,-3.20956871364999,10.5998668139723));
#59475=CARTESIAN_POINT('Ctrl Pts',(38.2274772437708,-4.9466092609614,9.90906477024764));
#59476=CARTESIAN_POINT('Ctrl Pts',(38.2670789224309,-6.41342335872562,8.84555941634984));
#59477=CARTESIAN_POINT('Ctrl Pts',(38.3066806010909,-7.88023745648985,7.78205406245204));
#59478=CARTESIAN_POINT('Ctrl Pts',(38.346282279751,-9.07682510470689,6.3458453983811));
#59479=CARTESIAN_POINT('Ctrl Pts',(38.3858839584111,-9.85804870295246,4.71113535537244));
#59480=CARTESIAN_POINT('Ctrl Pts',(38.421360363819,-10.5578929020702,3.24671167000465));
#59481=CARTESIAN_POINT('Ctrl Pts',(38.4568367692269,-10.9244020888775,1.62298806545424));
#59482=CARTESIAN_POINT('Ctrl Pts',(38.4923131746348,-10.9256735326657,-0.000180534162333964));
#59483=CARTESIAN_POINT('Origin',(21.9,0.,0.));
#59484=CARTESIAN_POINT('',(40.2076868253652,-10.924099487304,-7.99206701906295E-5));
#59485=CARTESIAN_POINT('',(39.9923131746348,-10.9240803938544,-3.60100876796591E-5));
#59486=CARTESIAN_POINT('',(21.9,-10.925,-1.33792662806848E-15));
#59487=CARTESIAN_POINT('Ctrl Pts',(40.2076868253652,-10.924099487304,-7.99206701906296E-5));
#59488=CARTESIAN_POINT('Ctrl Pts',(40.1859449007833,-10.923845062671,0.995100727968876));
#59489=CARTESIAN_POINT('Ctrl Pts',(40.1642029762013,-10.7890703805151,1.99034892697116));
#59490=CARTESIAN_POINT('Ctrl Pts',(40.1424610516194,-10.5206702796323,2.9481519792102));
#59491=CARTESIAN_POINT('Ctrl Pts',(40.1027730106697,-10.0307286392497,4.69654028843235));
#59492=CARTESIAN_POINT('Ctrl Pts',(40.0630849697199,-9.09552827885365,6.32015609346061));
#59493=CARTESIAN_POINT('Ctrl Pts',(40.0233969287702,-7.82898734844028,7.62122433239644));
#59494=CARTESIAN_POINT('Ctrl Pts',(39.9837088878205,-6.56244641802691,8.92229257133226));
#59495=CARTESIAN_POINT('Ctrl Pts',(39.9440208468707,-4.96456491759617,9.90081324417566));
#59496=CARTESIAN_POINT('Ctrl Pts',(39.904332805921,-3.22998317506861,10.4375912889367));
#59497=CARTESIAN_POINT('Ctrl Pts',(39.8646447649713,-1.49540143254105,10.9743693336978));
#59498=CARTESIAN_POINT('Ctrl Pts',(39.8249567240215,0.375880552083347,11.0694047503765));
#59499=CARTESIAN_POINT('Ctrl Pts',(39.7852686830718,2.15591913043771,10.7111211331637));
#59500=CARTESIAN_POINT('Ctrl Pts',(39.7455806421221,3.93595770879198,10.3528375159509));
#59501=CARTESIAN_POINT('Ctrl Pts',(39.7058926011724,5.62475288087622,9.54123486484658));
#59502=CARTESIAN_POINT('Ctrl Pts',(39.6662045602226,7.01658998895251,8.37517570879751));
#59503=CARTESIAN_POINT('Ctrl Pts',(39.6265165192729,8.4084270970288,7.20911655274844));
#59504=CARTESIAN_POINT('Ctrl Pts',(39.5868284783232,9.50330614109714,5.68860089175459));
#59505=CARTESIAN_POINT('Ctrl Pts',(39.5471404373734,10.1678582724726,3.9988450053928));
#59506=CARTESIAN_POINT('Ctrl Pts',(39.5074523964237,10.8324104038481,2.30908911903102));
#59507=CARTESIAN_POINT('Ctrl Pts',(39.467764355474,11.0666356225308,0.450093007301302));
#59508=CARTESIAN_POINT('Ctrl Pts',(39.4280763145242,10.8420026054231,-1.35169624187281));
#59509=CARTESIAN_POINT('Ctrl Pts',(39.3883882735745,10.6173695883153,-3.15348549104712));
#59510=CARTESIAN_POINT('Ctrl Pts',(39.3487002326248,9.93387833541694,-4.89806787766581));
#59511=CARTESIAN_POINT('Ctrl Pts',(39.309012191675,8.87478593525474,-6.37293322024241));
#59512=CARTESIAN_POINT('Ctrl Pts',(39.2693241507253,7.81569353509258,-7.84779856281892));
#59513=CARTESIAN_POINT('Ctrl Pts',(39.2296361097756,6.3809999876666,-9.05294686135336));
#59514=CARTESIAN_POINT('Ctrl Pts',(39.1899480688258,4.74546745295158,-9.84157720486179));
#59515=CARTESIAN_POINT('Ctrl Pts',(39.1502600278761,3.10993491823648,-10.6302075483703));
#59516=CARTESIAN_POINT('Ctrl Pts',(39.1105719869264,1.27356339623232,-11.0023199368527));
#59517=CARTESIAN_POINT('Ctrl Pts',(39.0708839459766,-0.539955960143817,
-10.9125868054911));
#59518=CARTESIAN_POINT('Ctrl Pts',(39.0311959050269,-2.35347531651965,-10.8228536741296));
#59519=CARTESIAN_POINT('Ctrl Pts',(38.9915078640772,-4.14414250726747,-10.2712750229242));
#59520=CARTESIAN_POINT('Ctrl Pts',(38.9518198231275,-5.69383369220201,-9.3250394697191));
#59521=CARTESIAN_POINT('Ctrl Pts',(38.9121317821777,-7.24352487713663,-8.37880391651396));
#59522=CARTESIAN_POINT('Ctrl Pts',(38.872443741228,-8.55224005625793,-7.03791146130905));
#59523=CARTESIAN_POINT('Ctrl Pts',(38.8327557002783,-9.46056268245166,-5.46569821319086));
#59524=CARTESIAN_POINT('Ctrl Pts',(38.7930676593286,-10.3688853086454,-3.89348496507267));
#59525=CARTESIAN_POINT('Ctrl Pts',(38.7533796183788,-10.8768153819115,-2.08995092404121));
#59526=CARTESIAN_POINT('Ctrl Pts',(38.7136915774291,-10.9224811827598,-0.274787260498275));
#59527=CARTESIAN_POINT('Ctrl Pts',(38.7116899934078,-10.924784242702,-0.183243246279994));
#59528=CARTESIAN_POINT('Ctrl Pts',(38.7096884093865,-10.9259115427141,-0.0916696523494821));
#59529=CARTESIAN_POINT('Ctrl Pts',(38.7076868253652,-10.9258695923078,-9.50230565660546E-5));
#59530=CARTESIAN_POINT('Ctrl Pts',(38.4923131746348,-10.9256735326657,-0.000180534162333964));
#59531=CARTESIAN_POINT('Ctrl Pts',(38.496438447887,-10.925821378903,-0.188926094226459));
#59532=CARTESIAN_POINT('Ctrl Pts',(38.5005637211392,-10.921030647636,-0.377664149768027));
#59533=CARTESIAN_POINT('Ctrl Pts',(38.5046889943913,-10.9112511777482,-0.566143358620799));
#59534=CARTESIAN_POINT('Ctrl Pts',(38.5442906730514,-10.8173705060243,-2.37550060765876));
#59535=CARTESIAN_POINT('Ctrl Pts',(38.5838923517115,-10.2637496143025,-4.16100368378816));
#59536=CARTESIAN_POINT('Ctrl Pts',(38.6234940303716,-9.31753879273393,-5.70608371935788));
#59537=CARTESIAN_POINT('Ctrl Pts',(38.6630957090316,-8.37132797116547,-7.25116375492752));
#59538=CARTESIAN_POINT('Ctrl Pts',(38.7026973876917,-7.03252721975041,-8.55582074993752));
#59539=CARTESIAN_POINT('Ctrl Pts',(38.7422990663518,-5.46352358033745,-9.46180905818329));
#59540=CARTESIAN_POINT('Ctrl Pts',(38.7819007450119,-3.89451994092449,-10.3677973664291));
#59541=CARTESIAN_POINT('Ctrl Pts',(38.821502423672,-2.09531341351361,-10.8751169879106));
#59542=CARTESIAN_POINT('Ctrl Pts',(38.861104102332,-0.284134997267554,-10.9222336483775));
#59543=CARTESIAN_POINT('Ctrl Pts',(38.9007057809921,1.52704341897861,-10.9693503088445));
#59544=CARTESIAN_POINT('Ctrl Pts',(38.9403074596522,3.35019372405997,-10.5562640082968));
#59545=CARTESIAN_POINT('Ctrl Pts',(38.9799091383122,4.96418070829368,-9.73307918707269));
#59546=CARTESIAN_POINT('Ctrl Pts',(39.0195108169723,6.5781676925274,-8.90989436584862));
#59547=CARTESIAN_POINT('Ctrl Pts',(39.0591124956324,7.98299135591348,-7.67661102394822));
#59548=CARTESIAN_POINT('Ctrl Pts',(39.0987141742925,9.00825654534549,-6.18281768934385));
#59549=CARTESIAN_POINT('Ctrl Pts',(39.1383158529526,10.0335217347774,-4.68902435473955));
#59550=CARTESIAN_POINT('Ctrl Pts',(39.1779175316126,10.6792284502554,-2.93472102743131));
#59551=CARTESIAN_POINT('Ctrl Pts',(39.2175192102727,10.8670570439023,-1.13269226667921));
#59552=CARTESIAN_POINT('Ctrl Pts',(39.2571208889328,11.0548856375493,0.669336494072881));
#59553=CARTESIAN_POINT('Ctrl Pts',(39.2967225675929,10.7848361093653,2.51909068826883));
#59554=CARTESIAN_POINT('Ctrl Pts',(39.3363242462529,10.0896635530325,4.19220824304222));
#59555=CARTESIAN_POINT('Ctrl Pts',(39.375925924913,9.3944909966996,5.86532579781571));
#59556=CARTESIAN_POINT('Ctrl Pts',(39.4155276035731,8.27419541221781,7.36180671316662));
#59557=CARTESIAN_POINT('Ctrl Pts',(39.4551292822332,6.86466071343179,8.50013846098337));
#59558=CARTESIAN_POINT('Ctrl Pts',(39.4947309608932,5.45512601464576,9.63847020880011));
#59559=CARTESIAN_POINT('Ctrl Pts',(39.5343326395533,3.75635220155551,10.4186527890827));
#59560=CARTESIAN_POINT('Ctrl Pts',(39.5739343182134,1.97438849693418,10.7460555847062));
#59561=CARTESIAN_POINT('Ctrl Pts',(39.6135359968735,0.192424792312943,11.0734583803297));
#59562=CARTESIAN_POINT('Ctrl Pts',(39.6531376755336,-1.67272880383937,10.9480813912943));
#59563=CARTESIAN_POINT('Ctrl Pts',(39.6927393541936,-3.39484238034768,10.3851319577087));
#59564=CARTESIAN_POINT('Ctrl Pts',(39.7323410328537,-5.116955956856,9.82218252412305));
#59565=CARTESIAN_POINT('Ctrl Pts',(39.7719427115138,-6.69602951372031,8.82166064598729));
#59566=CARTESIAN_POINT('Ctrl Pts',(39.8115443901738,-7.94053262082439,7.50492253551207));
#59567=CARTESIAN_POINT('Ctrl Pts',(39.8511460688339,-9.1850357279286,6.1881844250367));
#59568=CARTESIAN_POINT('Ctrl Pts',(39.890747747494,-10.0949683852725,4.5552300822218));
#59569=CARTESIAN_POINT('Ctrl Pts',(39.9303494261541,-10.559962211037,2.80412529461728));
#59570=CARTESIAN_POINT('Ctrl Pts',(39.951004008981,-10.8024835842012,1.89082211914788));
#59571=CARTESIAN_POINT('Ctrl Pts',(39.9716585918079,-10.9239713508352,0.945379302381534));
#59572=CARTESIAN_POINT('Ctrl Pts',(39.9923131746348,-10.9240803938544,-3.60100876796591E-5));
#59573=CARTESIAN_POINT('Origin',(21.9,0.,0.));
#59574=CARTESIAN_POINT('',(41.7076868253652,-10.925475895313,0.000234354564822142));
#59575=CARTESIAN_POINT('',(41.4923131746348,-10.9254652068462,0.000232978935392233));
#59576=CARTESIAN_POINT('',(21.9,-10.925,-1.33792662806848E-15));
#59577=CARTESIAN_POINT('Ctrl Pts',(41.7076868253652,-10.925475895313,0.000234354564822142));
#59578=CARTESIAN_POINT('Ctrl Pts',(41.7018894331298,-10.9257265140813,0.265499028847266));
#59579=CARTESIAN_POINT('Ctrl Pts',(41.6960920408943,-10.916261474432,0.530745855595144));
#59580=CARTESIAN_POINT('Ctrl Pts',(41.6902946486589,-10.8969558508505,0.795274499577191));
#59581=CARTESIAN_POINT('Ctrl Pts',(41.6506066077092,-10.7647925698189,2.60619624307596));
#59582=CARTESIAN_POINT('Ctrl Pts',(41.6109185667594,-10.1714446587326,4.38345993788012));
#59583=CARTESIAN_POINT('Ctrl Pts',(41.5712305258097,-9.18918965451365,5.91057476565502));
#59584=CARTESIAN_POINT('Ctrl Pts',(41.53154248486,-8.2069346502947,7.43768959342991));
#59585=CARTESIAN_POINT('Ctrl Pts',(41.4918544439102,-6.83577255294314,8.71465555417555));
#59586=CARTESIAN_POINT('Ctrl Pts',(41.4521664029605,-5.24272617344018,9.58592335368283));
#59587=CARTESIAN_POINT('Ctrl Pts',(41.4124783620108,-3.64967979393722,10.4571911531901));
#59588=CARTESIAN_POINT('Ctrl Pts',(41.372790321061,-1.83474913228286,10.9227607914591));
#59589=CARTESIAN_POINT('Ctrl Pts',(41.3331022801113,-0.0190138510533336,
10.925920623055));
#59590=CARTESIAN_POINT('Ctrl Pts',(41.2934142391616,1.79672143017619,10.9290804546509));
#59591=CARTESIAN_POINT('Ctrl Pts',(41.2537261982118,3.61326133098088,10.4698304795739));
#59592=CARTESIAN_POINT('Ctrl Pts',(41.2140381572621,5.20933054868226,9.60411257729075));
#59593=CARTESIAN_POINT('Ctrl Pts',(41.1743501163124,6.80539976638355,8.7383946750077));
#59594=CARTESIAN_POINT('Ctrl Pts',(41.1346620753627,8.18099830098156,7.46620884551866));
#59595=CARTESIAN_POINT('Ctrl Pts',(41.0949740344129,9.16856237635048,5.94252196453297));
#59596=CARTESIAN_POINT('Ctrl Pts',(41.0552859934632,10.1561264517194,4.41883508354728));
#59597=CARTESIAN_POINT('Ctrl Pts',(41.0155979525134,10.7556560678592,2.64364715106494));
#59598=CARTESIAN_POINT('Ctrl Pts',(40.9759099115637,10.8941216634813,0.833196443767102));
#59599=CARTESIAN_POINT('Ctrl Pts',(40.936221870614,11.0325872591033,-0.977254263530841));
#59600=CARTESIAN_POINT('Ctrl Pts',(40.8965338296643,10.7099888342075,-2.8229677456443));
#59601=CARTESIAN_POINT('Ctrl Pts',(40.8568457887146,9.96562256572442,-4.47911488536744));
#59602=CARTESIAN_POINT('Ctrl Pts',(40.8171577477648,9.22125629724133,-6.13526202509059));
#59603=CARTESIAN_POINT('Ctrl Pts',(40.7774697068151,8.05512218517096,-7.60184282242343));
#59604=CARTESIAN_POINT('Ctrl Pts',(40.7377816658653,6.60926877368134,-8.70021088714832));
#59605=CARTESIAN_POINT('Ctrl Pts',(40.6980936249156,5.16341536219173,-9.7985789518732));
#59606=CARTESIAN_POINT('Ctrl Pts',(40.6584055839659,3.43784265128285,-10.5287342839901));
#59607=CARTESIAN_POINT('Ctrl Pts',(40.6187175430162,1.64274522063448,-10.8017355722534));
#59608=CARTESIAN_POINT('Ctrl Pts',(40.5790295020665,-0.152352210013903,
-11.0747368605167));
#59609=CARTESIAN_POINT('Ctrl Pts',(40.5393414611167,-2.01697436040179,-10.8905841049264));
#59610=CARTESIAN_POINT('Ctrl Pts',(40.499653420167,-3.7239888239307,-10.2717092280521));
#59611=CARTESIAN_POINT('Ctrl Pts',(40.4599653792172,-5.43100328745952,-9.65283435117792));
#59612=CARTESIAN_POINT('Ctrl Pts',(40.4202773382675,-6.98041006412938,-8.59923735301986));
#59613=CARTESIAN_POINT('Ctrl Pts',(40.3805892973178,-8.18347360579004,-7.23925845427119));
#59614=CARTESIAN_POINT('Ctrl Pts',(40.340901256368,-9.38653714745063,-5.8792795555226));
#59615=CARTESIAN_POINT('Ctrl Pts',(40.3012132154183,-10.2432574541021,-4.21291875618345));
#59616=CARTESIAN_POINT('Ctrl Pts',(40.2615251744686,-10.6492761472432,-2.44315794980597));
#59617=CARTESIAN_POINT('Ctrl Pts',(40.2435790581008,-10.8328694549563,-1.64290848890024));
#59618=CARTESIAN_POINT('Ctrl Pts',(40.225632941733,-10.9243094932789,-0.821517216166159));
#59619=CARTESIAN_POINT('Ctrl Pts',(40.2076868253652,-10.924099487304,-7.99206701906296E-5));
#59620=CARTESIAN_POINT('Ctrl Pts',(39.9923131746348,-10.9240803938544,-3.60100876796591E-5));
#59621=CARTESIAN_POINT('Ctrl Pts',(40.011260270468,-10.9241804224316,-0.867295091407158));
#59622=CARTESIAN_POINT('Ctrl Pts',(40.0302073663011,-10.8221406483617,-1.73453102794972));
#59623=CARTESIAN_POINT('Ctrl Pts',(40.0491544621343,-10.6176946649518,-2.57691299198288));
#59624=CARTESIAN_POINT('Ctrl Pts',(40.0887561407944,-10.190378298917,-4.33759125858477));
#59625=CARTESIAN_POINT('Ctrl Pts',(40.1283578194545,-9.3156905726624,-5.98969255939464));
#59626=CARTESIAN_POINT('Ctrl Pts',(40.1679594981146,-8.09972490766372,-7.33282871657441));
#59627=CARTESIAN_POINT('Ctrl Pts',(40.2075611767746,-6.8837592426651,-8.67596487375412));
#59628=CARTESIAN_POINT('Ctrl Pts',(40.2471628554347,-5.32651563892247,-9.71013588730377));
#59629=CARTESIAN_POINT('Ctrl Pts',(40.2867645340947,-3.6168767079916,-10.3099041433775));
#59630=CARTESIAN_POINT('Ctrl Pts',(40.3263662127548,-1.90723777706044,-10.9096723994513));
#59631=CARTESIAN_POINT('Ctrl Pts',(40.3659678914149,-0.0452035189409916,
-11.0750378980491));
#59632=CARTESIAN_POINT('Ctrl Pts',(40.405569570075,1.74337450883045,-10.7859429763104));
#59633=CARTESIAN_POINT('Ctrl Pts',(40.4451712487351,3.53195253660178,-10.4968480545718));
#59634=CARTESIAN_POINT('Ctrl Pts',(40.4847729273951,5.24707433402511,-9.75329271249677));
#59635=CARTESIAN_POINT('Ctrl Pts',(40.5243746060552,6.68070778361492,-8.64546494278017));
#59636=CARTESIAN_POINT('Ctrl Pts',(40.5639762847153,8.11434123320465,-7.53763717306364));
#59637=CARTESIAN_POINT('Ctrl Pts',(40.6035779633754,9.26648633496089,-6.06553697570556));
#59638=CARTESIAN_POINT('Ctrl Pts',(40.6431796420355,9.99739605450524,-4.40771967062263));
#59639=CARTESIAN_POINT('Ctrl Pts',(40.6827813206955,10.7283057740496,-2.74990236553969));
#59640=CARTESIAN_POINT('Ctrl Pts',(40.7223829993556,11.037980111382,-0.906367952731887));
#59641=CARTESIAN_POINT('Ctrl Pts',(40.7619846780157,10.888857764009,0.899275910504303));
#59642=CARTESIAN_POINT('Ctrl Pts',(40.8015863566757,10.7397354166359,2.7049197737407));
#59643=CARTESIAN_POINT('Ctrl Pts',(40.8411880353358,10.1318163845573,4.47267308740548));
#59644=CARTESIAN_POINT('Ctrl Pts',(40.8807897139959,9.13883693810524,5.98811990389173));
#59645=CARTESIAN_POINT('Ctrl Pts',(40.920391392656,8.1458574916533,7.5035667203778));
#59646=CARTESIAN_POINT('Ctrl Pts',(40.9599930713161,6.76781763082806,8.76670703968541));
#59647=CARTESIAN_POINT('Ctrl Pts',(40.9995947499761,5.17186382213639,9.62433089475168));
#59648=CARTESIAN_POINT('Ctrl Pts',(41.0391964286362,3.57591001344472,10.481954749818));
#59649=CARTESIAN_POINT('Ctrl Pts',(41.0787981072963,1.76204225688662,10.9340621406429));
#59650=CARTESIAN_POINT('Ctrl Pts',(41.1183997859564,-0.0497301428976236,
10.9258156439683));
#59651=CARTESIAN_POINT('Ctrl Pts',(41.1580014646164,-1.86150254268187,10.9175691472937));
#59652=CARTESIAN_POINT('Ctrl Pts',(41.1976031432765,-3.67117958569226,10.4489687631197));
#59653=CARTESIAN_POINT('Ctrl Pts',(41.2372048219366,-5.25926027788115,9.57685239905937));
#59654=CARTESIAN_POINT('Ctrl Pts',(41.2768065005967,-6.84734097007014,8.70473603499902));
#59655=CARTESIAN_POINT('Ctrl Pts',(41.3164081792568,-8.2138253114376,7.42910369105241));
#59656=CARTESIAN_POINT('Ctrl Pts',(41.3560098579168,-9.19296842830681,5.90468052431769));
#59657=CARTESIAN_POINT('Ctrl Pts',(41.3956115365769,-10.172111545176,4.38025735758297));
#59658=CARTESIAN_POINT('Ctrl Pts',(41.435213215237,-10.763913437547,2.60704336806013));
#59659=CARTESIAN_POINT('Ctrl Pts',(41.474814893897,-10.8965927471028,0.800116853296611));
#59660=CARTESIAN_POINT('Ctrl Pts',(41.4806476541429,-10.916134509685,0.533982449422622));
#59661=CARTESIAN_POINT('Ctrl Pts',(41.4864804143889,-10.9257164929786,0.267116717308136));
#59662=CARTESIAN_POINT('Ctrl Pts',(41.4923131746348,-10.9254652068462,0.000232978935392233));
#59663=CARTESIAN_POINT('Origin',(21.9,0.,0.));
#59664=CARTESIAN_POINT('',(43.,-10.925,-1.33792662806848E-15));
#59665=CARTESIAN_POINT('',(42.9923131746348,-10.9250461896976,-0.000265489735796583));
#59666=CARTESIAN_POINT('',(21.9,-10.925,-1.33792662806848E-15));
#59667=CARTESIAN_POINT('',(43.,-7.04509292776794,8.3499874634106));
#59668=CARTESIAN_POINT('Origin',(43.,0.,0.));
#59669=CARTESIAN_POINT('Ctrl Pts',(43.,-7.04509292776818,8.3499874634104));
#59670=CARTESIAN_POINT('Ctrl Pts',(42.9603119590503,-5.65695028748072,9.52119807189056));
#59671=CARTESIAN_POINT('Ctrl Pts',(42.9206239181005,-3.97182972959699,10.3390008126884));
#59672=CARTESIAN_POINT('Ctrl Pts',(42.8809358771508,-2.19329530207865,10.7035797581239));
#59673=CARTESIAN_POINT('Ctrl Pts',(42.8412478362011,-0.414760874560405,
11.0681587035593));
#59674=CARTESIAN_POINT('Ctrl Pts',(42.8015597952514,1.45718742259244,10.9795138536324));
#59675=CARTESIAN_POINT('Ctrl Pts',(42.7618717543016,3.19371524349622,10.4487440616195));
#59676=CARTESIAN_POINT('Ctrl Pts',(42.7221837133519,4.93024306440009,9.9179742696066));
#59677=CARTESIAN_POINT('Ctrl Pts',(42.6824956724022,6.53135040905488,8.94507953550763));
#59678=CARTESIAN_POINT('Ctrl Pts',(42.6428076314524,7.80237050218005,7.64844176312899));
#59679=CARTESIAN_POINT('Ctrl Pts',(42.6031195905027,9.07339059530523,6.35180399075036));
#59680=CARTESIAN_POINT('Ctrl Pts',(42.5634315495529,10.0143234369008,4.73142318009206));
#59681=CARTESIAN_POINT('Ctrl Pts',(42.5237435086032,10.5103684390786,2.98474348774657));
#59682=CARTESIAN_POINT('Ctrl Pts',(42.4840554676535,11.0064134412565,1.23806379540118));
#59683=CARTESIAN_POINT('Ctrl Pts',(42.4443674267038,11.0575706040167,-0.634914778631374));
#59684=CARTESIAN_POINT('Ctrl Pts',(42.4046793857541,10.657703158648,-2.40607430272475));
#59685=CARTESIAN_POINT('Ctrl Pts',(42.3649913448043,10.2578357132793,-4.17723382681823));
#59686=CARTESIAN_POINT('Ctrl Pts',(42.3253033038546,9.40694365978164,-5.84657430097252));
#59687=CARTESIAN_POINT('Ctrl Pts',(42.2856152629048,8.20862642789346,-7.21073414169468));
#59688=CARTESIAN_POINT('Ctrl Pts',(42.2459272219551,7.01030919600528,-8.57489398241685));
#59689=CARTESIAN_POINT('Ctrl Pts',(42.2062391810054,5.46456678572653,-9.6338731897069));
#59690=CARTESIAN_POINT('Ctrl Pts',(42.1665511400557,3.75971374656667,-10.2586845863707));
#59691=CARTESIAN_POINT('Ctrl Pts',(42.126863099106,2.0548607074068,-10.8834959830345));
#59692=CARTESIAN_POINT('Ctrl Pts',(42.0871750581562,0.190897039365813,-11.0741395690722));
#59693=CARTESIAN_POINT('Ctrl Pts',(42.0474870172065,-1.60513819395432,-10.807388282526));
#59694=CARTESIAN_POINT('Ctrl Pts',(42.0077989762567,-3.40117342727445,-10.5406369959798));
#59695=CARTESIAN_POINT('Ctrl Pts',(41.968110935307,-5.12928022587372,-9.81649083684975));
#59696=CARTESIAN_POINT('Ctrl Pts',(41.9284228943573,-6.57894852673386,-8.72316144904941));
#59697=CARTESIAN_POINT('Ctrl Pts',(41.8887348534075,-8.02861682759391,-7.62983206124914));
#59698=CARTESIAN_POINT('Ctrl Pts',(41.8490468124578,-9.19984663071486,-6.16731944477856));
#59699=CARTESIAN_POINT('Ctrl Pts',(41.8093587715081,-9.94997220678691,-4.51377324044664));
#59700=CARTESIAN_POINT('Ctrl Pts',(41.7754681227938,-10.5905239141001,-3.1017672002681));
#59701=CARTESIAN_POINT('Ctrl Pts',(41.7415774740795,-10.9240108171721,-1.55046146302586));
#59702=CARTESIAN_POINT('Ctrl Pts',(41.7076868253652,-10.925475895313,0.000234354564822142));
#59703=CARTESIAN_POINT('Ctrl Pts',(41.4923131746348,-10.9254652068462,0.000232978935392233));
#59704=CARTESIAN_POINT('Ctrl Pts',(41.5260820930489,-10.9240103791924,-1.54489742368667));
#59705=CARTESIAN_POINT('Ctrl Pts',(41.5598510114631,-10.592957990056,-3.09063137112752));
#59706=CARTESIAN_POINT('Ctrl Pts',(41.5936199298773,-9.95685815051506,-4.49854381483149));
#59707=CARTESIAN_POINT('Ctrl Pts',(41.6332216085373,-9.21088751763084,-6.14963892819208));
#59708=CARTESIAN_POINT('Ctrl Pts',(41.6728232871974,-8.0453895251219,-7.61119011490895));
#59709=CARTESIAN_POINT('Ctrl Pts',(41.7124249658575,-6.60173088047647,-8.70592154178067));
#59710=CARTESIAN_POINT('Ctrl Pts',(41.7520266445176,-5.15807223583097,-9.80065296865245));
#59711=CARTESIAN_POINT('Ctrl Pts',(41.7916283231776,-3.43625293904881,-10.5285646356789));
#59712=CARTESIAN_POINT('Ctrl Pts',(41.8312300018377,-1.64511734704432,-10.8013660819361));
#59713=CARTESIAN_POINT('Ctrl Pts',(41.8708316804978,0.146018244960175,-11.0741675281932));
#59714=CARTESIAN_POINT('Ctrl Pts',(41.9104333591579,2.00647013218733,-10.8918587536813));
#59715=CARTESIAN_POINT('Ctrl Pts',(41.950035037818,3.71057845616067,-10.2765523951267));
#59716=CARTESIAN_POINT('Ctrl Pts',(41.9896367164781,5.41468678013393,-9.66124603657213));
#59717=CARTESIAN_POINT('Ctrl Pts',(42.0292383951381,6.96245154085346,-8.61294209397497));
#59718=CARTESIAN_POINT('Ctrl Pts',(42.0688400737981,8.1661402901371,-7.25879264766247));
#59719=CARTESIAN_POINT('Ctrl Pts',(42.1084417524582,9.36982903942075,-5.90464320134997));
#59720=CARTESIAN_POINT('Ctrl Pts',(42.1480434311184,10.2294417772686,-4.24464825132207));
#59721=CARTESIAN_POINT('Ctrl Pts',(42.1876451097784,10.6407127079445,-2.48015295079122));
#59722=CARTESIAN_POINT('Ctrl Pts',(42.2272467884385,11.0519836386205,-0.715657650260262));
#59723=CARTESIAN_POINT('Ctrl Pts',(42.2668484670986,11.0149127621247,1.15333800077373));
#59724=CARTESIAN_POINT('Ctrl Pts',(42.3064501457586,10.5339981815288,2.90013717216149));
#59725=CARTESIAN_POINT('Ctrl Pts',(42.3460518244187,10.053083600933,4.64693634354925));
#59726=CARTESIAN_POINT('Ctrl Pts',(42.3856535030788,9.12832531623736,6.27153903529053));
#59727=CARTESIAN_POINT('Ctrl Pts',(42.4252551817389,7.87188672874755,7.57689420453102));
#59728=CARTESIAN_POINT('Ctrl Pts',(42.4648568603989,6.61544814125781,8.88224937377143));
#59729=CARTESIAN_POINT('Ctrl Pts',(42.504458539059,5.02732925097376,9.86835702051096));
#59730=CARTESIAN_POINT('Ctrl Pts',(42.5440602177191,3.3001638525746,10.4156058978145));
#59731=CARTESIAN_POINT('Ctrl Pts',(42.5836618963792,1.57299845417534,10.962854775118));
#59732=CARTESIAN_POINT('Ctrl Pts',(42.6232635750392,-0.293213452338988,
11.0712448829856));
#59733=CARTESIAN_POINT('Ctrl Pts',(42.6628652536993,-2.0721256279404,10.7276357985186));
#59734=CARTESIAN_POINT('Ctrl Pts',(42.7024669323594,-3.85103780354181,10.3840267140515));
#59735=CARTESIAN_POINT('Ctrl Pts',(42.7420686110195,-5.54265024823005,9.58841843724966));
#59736=CARTESIAN_POINT('Ctrl Pts',(42.7816702896796,-6.94175910118757,8.43729999632218));
#59737=CARTESIAN_POINT('Ctrl Pts',(42.8212719683396,-8.34086795414502,7.28618155539477));
#59738=CARTESIAN_POINT('Ctrl Pts',(42.8608736469997,-9.44747321537185,5.77955295034171));
#59739=CARTESIAN_POINT('Ctrl Pts',(42.9004753256598,-10.127396467996,4.10018193913994));
#59740=CARTESIAN_POINT('Ctrl Pts',(42.9310879419848,-10.6529860482179,2.80200615031686));
#59741=CARTESIAN_POINT('Ctrl Pts',(42.9617005583098,-10.923612114048,1.40060826619046));
#59742=CARTESIAN_POINT('Ctrl Pts',(42.9923131746348,-10.9250461896976,-0.000265489735796583));
#59743=CARTESIAN_POINT('Origin',(-2.04781266907391,0.,0.));
#59744=CARTESIAN_POINT('',(42.2021873309261,-10.0689385859916,0.000215981596605526));
#59745=CARTESIAN_POINT('',(42.4978126690739,-10.0685425685098,-0.000244675825605278));
#59746=CARTESIAN_POINT('',(-2.04781266907391,-10.0685,8.88799240754737E-13));
#59747=CARTESIAN_POINT('',(43.,9.86762259782016,2.00332725038358));
#59748=CARTESIAN_POINT('Ctrl Pts',(42.2021873309266,-10.0689385859908,0.000215981596605394));
#59749=CARTESIAN_POINT('Ctrl Pts',(42.2360779796409,-10.0675883672941,-1.42890812269744));
#59750=CARTESIAN_POINT('Ctrl Pts',(42.3096566693049,-9.40032961524582,-4.5328451011598));
#59751=CARTESIAN_POINT('Ctrl Pts',(42.4229233999187,-6.31978043532264,-8.37952150001038));
#59752=CARTESIAN_POINT('Ctrl Pts',(42.5419875227679,-1.54190126780919,-10.3816447777769));
#59753=CARTESIAN_POINT('Ctrl Pts',(42.6610516456171,3.61159571846151,-9.85455234408739));
#59754=CARTESIAN_POINT('Ctrl Pts',(42.7801157684663,7.88527282360298,-6.92668081586803));
#59755=CARTESIAN_POINT('Ctrl Pts',(42.8930985532607,10.1176645764172,-2.54701609597499));
#59756=CARTESIAN_POINT('Ctrl Pts',(42.9663932971055,10.1482197730519,0.614217294036058));
#59757=CARTESIAN_POINT('Ctrl Pts',(43.0000000000005,9.86762259781931,2.0033272503834));
#59758=CARTESIAN_POINT('',(43.,5.1139286979658,-8.67308627433867));
#59759=CARTESIAN_POINT('Origin',(43.,0.,0.));
#59760=CARTESIAN_POINT('Ctrl Pts',(42.4978126690739,-10.0685425685098,-0.000244675825604758));
#59761=CARTESIAN_POINT('Ctrl Pts',(42.5068017314089,-10.0689306557233,-0.379346846978384));
#59762=CARTESIAN_POINT('Ctrl Pts',(42.5553924724041,-9.95539795674085,-2.42837386975631));
#59763=CARTESIAN_POINT('Ctrl Pts',(42.6435848920593,-8.59726759665103,-6.01677379735012));
#59764=CARTESIAN_POINT('Ctrl Pts',(42.7623899280396,-4.68275676202098,-9.39082860495563));
#59765=CARTESIAN_POINT('Ctrl Pts',(42.8811949640197,0.368965693322309,-10.4874893880972));
#59766=CARTESIAN_POINT('Ctrl Pts',(42.9603983213399,3.6752100549675,-9.52140074095435));
#59767=CARTESIAN_POINT('Ctrl Pts',(43.,5.1139286979658,-8.67308627433867));
#59768=CARTESIAN_POINT('Origin',(-2.04781266907391,0.,0.));
#59769=CARTESIAN_POINT('',(40.7021873309261,-10.0676700858508,-7.36550355973785E-5));
#59770=CARTESIAN_POINT('',(40.9978126690739,-10.0689287354811,0.000214713814004203));
#59771=CARTESIAN_POINT('',(-2.04781266907391,-10.0685,8.88799240754737E-13));
#59772=CARTESIAN_POINT('Ctrl Pts',(40.7021873309266,-10.0676700858499,-7.36550355971699E-5));
#59773=CARTESIAN_POINT('Ctrl Pts',(40.7201334472944,-10.0678636277409,-0.757111770339985));
#59774=CARTESIAN_POINT('Ctrl Pts',(40.7777676046119,-9.79722536545769,-3.18821209340595));
#59775=CARTESIAN_POINT('Ctrl Pts',(40.8750898028791,-7.86109481570529,-6.95407596456924));
#59776=CARTESIAN_POINT('Ctrl Pts',(40.9941539257284,-3.57728645024092,-9.86706673142152));
#59777=CARTESIAN_POINT('Ctrl Pts',(41.1132180485776,1.57803111163873,-10.376213281443));
#59778=CARTESIAN_POINT('Ctrl Pts',(41.2322821714268,6.34890401958871,-8.35747580919987));
#59779=CARTESIAN_POINT('Ctrl Pts',(41.351346294276,9.57303801703849,-4.30266516628609));
#59780=CARTESIAN_POINT('Ctrl Pts',(41.4704104171251,10.4649599138979,0.80037360570219));
#59781=CARTESIAN_POINT('Ctrl Pts',(41.5894745399744,8.80737713858352,5.70842295074491));
#59782=CARTESIAN_POINT('Ctrl Pts',(41.7085386628235,5.00411475535267,9.22576931894892));
#59783=CARTESIAN_POINT('Ctrl Pts',(41.8276027856728,-0.0182647388121033,
10.4955061722386));
#59784=CARTESIAN_POINT('Ctrl Pts',(41.9466669085219,-5.03619499973622,9.20829667944856));
#59785=CARTESIAN_POINT('Ctrl Pts',(42.0657310313711,-8.82719149690324,5.67773417809401));
#59786=CARTESIAN_POINT('Ctrl Pts',(42.150904505506,-10.000730279081,2.16261626322584));
#59787=CARTESIAN_POINT('Ctrl Pts',(42.1963899386912,-10.0691695567064,0.244684391025481));
#59788=CARTESIAN_POINT('Ctrl Pts',(42.2021873309266,-10.0689385859908,0.000215981596605394));
#59789=CARTESIAN_POINT('Ctrl Pts',(40.9978126690739,-10.0689287354811,0.000214713814003717));
#59790=CARTESIAN_POINT('Ctrl Pts',(41.031581587488,-10.0675879636521,-1.4237802938567));
#59791=CARTESIAN_POINT('Ctrl Pts',(41.1049521845622,-9.40469263644049,-4.51893938195157));
#59792=CARTESIAN_POINT('Ctrl Pts',(41.2179244602966,-6.34052063122281,-8.36145499271618));
#59793=CARTESIAN_POINT('Ctrl Pts',(41.3367294962768,-1.58002518326458,-10.3739891673947));
#59794=CARTESIAN_POINT('Ctrl Pts',(41.4555345322571,3.56376241212563,-9.86994086638596));
#59795=CARTESIAN_POINT('Ctrl Pts',(41.5743395682372,7.84303092287294,-6.97158436861771));
#59796=CARTESIAN_POINT('Ctrl Pts',(41.6931446042175,10.2196929414599,-2.38202121410348));
#59797=CARTESIAN_POINT('Ctrl Pts',(41.8119496401977,10.1171991785312,2.78538822638215));
#59798=CARTESIAN_POINT('Ctrl Pts',(41.9307546761779,7.56042239424033,7.27709867081222));
#59799=CARTESIAN_POINT('Ctrl Pts',(42.0495597121582,3.16958256444921,10.0034945082114));
#59800=CARTESIAN_POINT('Ctrl Pts',(42.1683647481384,-1.99013036390094,10.3031720737214));
#59801=CARTESIAN_POINT('Ctrl Pts',(42.2871697841186,-6.6671097412949,8.10346994054641));
#59802=CARTESIAN_POINT('Ctrl Pts',(42.3969857577638,-9.49516558180456,4.25310886303304));
#59803=CARTESIAN_POINT('Ctrl Pts',(42.4672000527489,-10.0672209217658,1.29080314216428));
#59804=CARTESIAN_POINT('Ctrl Pts',(42.4978126690739,-10.0685425685098,-0.000244675825604758));
#59805=CARTESIAN_POINT('Origin',(-2.04781266907391,0.,0.));
#59806=CARTESIAN_POINT('',(39.2021873309261,-10.0693014178628,-8.75734228172276E-5));
#59807=CARTESIAN_POINT('',(39.4978126690739,-10.0676524892927,-3.3186962086762E-5));
#59808=CARTESIAN_POINT('',(-2.04781266907391,-10.0685,8.88799240754737E-13));
#59809=CARTESIAN_POINT('Ctrl Pts',(39.2021873309266,-10.0693014178619,-8.75734228174448E-5));
#59810=CARTESIAN_POINT('Ctrl Pts',(39.2041889149479,-10.0693400794332,-0.0844829194214082));
#59811=CARTESIAN_POINT('Ctrl Pts',(39.245878539919,-10.0477010885783,-1.84227600061968));
#59812=CARTESIAN_POINT('Ctrl Pts',(39.3272562058397,-9.0878743970168,-5.25038314535039));
#59813=CARTESIAN_POINT('Ctrl Pts',(39.4463203286889,-5.46953148233069,-8.9576899696698));
#59814=CARTESIAN_POINT('Ctrl Pts',(39.5653844515381,-0.518684999023309,
-10.4826976537873));
#59815=CARTESIAN_POINT('Ctrl Pts',(39.6844485743872,4.55852507034851,-9.45387927847339));
#59816=CARTESIAN_POINT('Ctrl Pts',(39.8035126972365,8.52517366959541,-6.12187864402225));
#59817=CARTESIAN_POINT('Ctrl Pts',(39.9225768200856,10.4148940393362,-1.29844768026914));
#59818=CARTESIAN_POINT('Ctrl Pts',(40.0416409429349,9.76730686835976,3.84131497903059));
#59819=CARTESIAN_POINT('Ctrl Pts',(40.160705065784,6.74017927425415,8.04524502920423));
#59820=CARTESIAN_POINT('Ctrl Pts',(40.2797691886333,2.07098910762834,10.2891684962916));
#59821=CARTESIAN_POINT('Ctrl Pts',(40.3988333114824,-3.10274160052417,10.0264140543247));
#59822=CARTESIAN_POINT('Ctrl Pts',(40.5178974343316,-7.52057314846527,7.32099472402093));
#59823=CARTESIAN_POINT('Ctrl Pts',(40.619015440813,-9.71649475108489,3.50862127807146));
#59824=CARTESIAN_POINT('Ctrl Pts',(40.6804454063447,-10.0674356076424,0.917086652590996));
#59825=CARTESIAN_POINT('Ctrl Pts',(40.7021873309266,-10.0676700858499,-7.36550355971699E-5));
#59826=CARTESIAN_POINT('Ctrl Pts',(39.4978126690739,-10.0676524892927,-3.31869620865538E-5));
#59827=CARTESIAN_POINT('Ctrl Pts',(39.516759764907,-10.0677446758126,-0.799300743965954));
#59828=CARTESIAN_POINT('Ctrl Pts',(39.5753085394002,-9.77714978491082,-3.26906642762086));
#59829=CARTESIAN_POINT('Ctrl Pts',(39.6734589925537,-7.77924367588624,-7.04269121111839));
#59830=CARTESIAN_POINT('Ctrl Pts',(39.7922640285338,-3.47376800789063,-9.90197290903841));
#59831=CARTESIAN_POINT('Ctrl Pts',(39.9110690645141,1.67439453523271,-10.3591763477472));
#59832=CARTESIAN_POINT('Ctrl Pts',(40.0298741004943,6.41637270018189,-8.30339045437917));
#59833=CARTESIAN_POINT('Ctrl Pts',(40.1486791364745,9.60182980508796,-4.23331974396269));
#59834=CARTESIAN_POINT('Ctrl Pts',(40.2674841724548,10.4580191136734,0.863694325242524));
#59835=CARTESIAN_POINT('Ctrl Pts',(40.386289208435,8.77724123509683,5.75118839534756));
#59836=CARTESIAN_POINT('Ctrl Pts',(40.5050942444152,4.96722905970481,9.24352568732455));
#59837=CARTESIAN_POINT('Ctrl Pts',(40.6238992803954,-0.0477624753722201,
10.493514684447));
#59838=CARTESIAN_POINT('Ctrl Pts',(40.7427043163757,-5.0511675026172,9.19792576873352));
#59839=CARTESIAN_POINT('Ctrl Pts',(40.8615093523559,-8.82923091434941,5.67105045842888));
#59840=CARTESIAN_POINT('Ctrl Pts',(40.946545469922,-10.0003727806755,2.16196208298385));
#59841=CARTESIAN_POINT('Ctrl Pts',(40.991979908828,-10.0691603212407,0.246175255672483));
#59842=CARTESIAN_POINT('Ctrl Pts',(40.9978126690739,-10.0689287354811,0.000214713814003717));
#59843=CARTESIAN_POINT('Origin',(-2.04781266907391,0.,0.));
#59844=CARTESIAN_POINT('',(37.7021873309261,-10.067932551961,0.000203422982869468));
#59845=CARTESIAN_POINT('',(37.9978126690739,-10.0691207289378,-0.000166380613864647));
#59846=CARTESIAN_POINT('',(-2.04781266907391,-10.0685,8.88799240754737E-13));
#59847=CARTESIAN_POINT('Ctrl Pts',(37.7021873309266,-10.0679325519601,0.000203422982869433));
#59848=CARTESIAN_POINT('Ctrl Pts',(37.7279324235511,-10.0671394904526,-1.08574527402579));
#59849=CARTESIAN_POINT('Ctrl Pts',(37.7933655571254,-9.62218897948878,-3.84640172777887));
#59850=CARTESIAN_POINT('Ctrl Pts',(37.8984867316494,-7.14292981451776,-7.68989843195632));
#59851=CARTESIAN_POINT('Ctrl Pts',(38.0175508544986,-2.59464750158812,-10.1697486975556));
#59852=CARTESIAN_POINT('Ctrl Pts',(38.1366149773478,2.58575057232614,-10.1720144615826));
#59853=CARTESIAN_POINT('Ctrl Pts',(38.255679100197,7.13620038169131,-7.69614373184913));
#59854=CARTESIAN_POINT('Ctrl Pts',(38.3747432230462,9.948107775545,-3.34531551801509));
#59855=CARTESIAN_POINT('Ctrl Pts',(38.4938073458954,10.3364274901293,1.82050843728659));
#59856=CARTESIAN_POINT('Ctrl Pts',(38.6128714687446,8.20655591869616,6.54281469875498));
#59857=CARTESIAN_POINT('Ctrl Pts',(38.7319355915937,4.07737872427021,9.6711409341297));
#59858=CARTESIAN_POINT('Ctrl Pts',(38.8509997144429,-1.04514163277688,10.4433549779928));
#59859=CARTESIAN_POINT('Ctrl Pts',(38.9700638372921,-5.91304146887271,8.67132774241194));
#59860=CARTESIAN_POINT('Ctrl Pts',(39.08712637612,-9.28277146471235,4.85206906116672));
#59861=CARTESIAN_POINT('Ctrl Pts',(39.1645008739982,-10.0685734855718,1.58893468998866));
#59862=CARTESIAN_POINT('Ctrl Pts',(39.2021873309266,-10.0693014178619,-8.75734228174448E-5));
#59863=CARTESIAN_POINT('Ctrl Pts',(37.9978126690739,-10.0691207289378,-0.000166380613864248));
#59864=CARTESIAN_POINT('Ctrl Pts',(38.0019379423261,-10.0692569843007,-0.174114634298781));
#59865=CARTESIAN_POINT('Ctrl Pts',(38.0456648942383,-10.0224574401508,-2.01785298460805));
#59866=CARTESIAN_POINT('Ctrl Pts',(38.1289935248106,-8.94887240670967,-5.48031151599342));
#59867=CARTESIAN_POINT('Ctrl Pts',(38.2477985607909,-5.24734873651581,-9.08743434096145));
#59868=CARTESIAN_POINT('Ctrl Pts',(38.3666035967711,-0.27289264830437,-10.4900744166284));
#59869=CARTESIAN_POINT('Ctrl Pts',(38.4854086327514,4.76776332790926,-9.34797114420792));
#59870=CARTESIAN_POINT('Ctrl Pts',(38.6042136687316,8.65182750771774,-5.93818258734095));
#59871=CARTESIAN_POINT('Ctrl Pts',(38.7230187047118,10.4370809808865,-1.08787511338123));
#59872=CARTESIAN_POINT('Ctrl Pts',(38.841823740692,9.69044656225397,4.02633544156494));
#59873=CARTESIAN_POINT('Ctrl Pts',(38.9606287766723,6.59304717762569,8.16381409498656));
#59874=CARTESIAN_POINT('Ctrl Pts',(39.0794338126525,1.89626800954364,10.3208671777074));
#59875=CARTESIAN_POINT('Ctrl Pts',(39.1982388486327,-3.26051889650485,9.9742241898529));
#59876=CARTESIAN_POINT('Ctrl Pts',(39.3170438846129,-7.62635013878093,7.20797580632616));
#59877=CARTESIAN_POINT('Ctrl Pts',(39.4169018247601,-9.74091781227908,3.4131977667139));
#59878=CARTESIAN_POINT('Ctrl Pts',(39.477158086247,-10.0675519950466,0.871263295746859));
#59879=CARTESIAN_POINT('Ctrl Pts',(39.4978126690739,-10.0676524892927,-3.31869620865538E-5));
#59880=CARTESIAN_POINT('Origin',(-2.04781266907391,0.,0.));
#59881=CARTESIAN_POINT('',(36.2021873309261,-10.0684139656564,-0.000261209358190219));
#59882=CARTESIAN_POINT('',(36.4978126690739,-10.0682971267649,0.000254225486309434));
#59883=CARTESIAN_POINT('',(-2.04781266907391,-10.0685,8.88799240754737E-13));
#59884=CARTESIAN_POINT('Ctrl Pts',(36.2021873309266,-10.0684139656555,-0.000261209358190344));
#59885=CARTESIAN_POINT('Ctrl Pts',(36.2119878912047,-10.0688319632613,-0.413599984478035));
#59886=CARTESIAN_POINT('Ctrl Pts',(36.2614764924324,-9.94272748910106,-2.50052911104218));
#59887=CARTESIAN_POINT('Ctrl Pts',(36.3506531346099,-8.53052549054089,-6.11441894902236));
#59888=CARTESIAN_POINT('Ctrl Pts',(36.4697172574591,-4.56679305970356,-9.44988811461674));
#59889=CARTESIAN_POINT('Ctrl Pts',(36.5887813803082,0.509515113475162,-10.4831473603146));
#59890=CARTESIAN_POINT('Ctrl Pts',(36.7078455031575,5.46169369545109,-8.96247098773554));
#59891=CARTESIAN_POINT('Ctrl Pts',(36.8269096260067,9.08327817381496,-5.25833070907757));
#59892=CARTESIAN_POINT('Ctrl Pts',(36.9459737488559,10.4919673392078,-0.273140223929764));
#59893=CARTESIAN_POINT('Ctrl Pts',(37.0650378717051,9.34457213676633,4.77859349701376));
#59894=CARTESIAN_POINT('Ctrl Pts',(37.1841019945542,5.92062440698051,8.66615202153747));
#59895=CARTESIAN_POINT('Ctrl Pts',(37.3031661174034,1.05427650521303,10.4424367500831));
#59896=CARTESIAN_POINT('Ctrl Pts',(37.4222302402527,-4.06891738236679,9.67470390060619));
#59897=CARTESIAN_POINT('Ctrl Pts',(37.5412943631018,-8.20082948466987,6.54999083910055));
#59898=CARTESIAN_POINT('Ctrl Pts',(37.6346133933265,-9.87339845227709,2.85024485823725));
#59899=CARTESIAN_POINT('Ctrl Pts',(37.6882443826014,-10.0683620557797,0.588328188623868));
#59900=CARTESIAN_POINT('Ctrl Pts',(37.7021873309266,-10.0679325519601,0.000203422982869433));
#59901=CARTESIAN_POINT('Ctrl Pts',(36.4978126690739,-10.0682971267649,0.000254225486309226));
#59902=CARTESIAN_POINT('Ctrl Pts',(36.5267177984052,-10.0671167499389,-1.21886092536785));
#59903=CARTESIAN_POINT('Ctrl Pts',(36.5952246063965,-9.54158770153698,-4.10922348578581));
#59904=CARTESIAN_POINT('Ctrl Pts',(36.7033330930479,-6.83941677764739,-7.9585494787389));
#59905=CARTESIAN_POINT('Ctrl Pts',(36.8221381290282,-2.21074011661143,-10.2581070281365));
#59906=CARTESIAN_POINT('Ctrl Pts',(36.9409431650084,2.95423075766473,-10.0691932295675));
#59907=CARTESIAN_POINT('Ctrl Pts',(37.0597482009886,7.40254712876932,-7.43763589255681));
#59908=CARTESIAN_POINT('Ctrl Pts',(37.1785532369688,10.0551105035959,-3.00181352258519));
#59909=CARTESIAN_POINT('Ctrl Pts',(37.2973582729491,10.2684466096674,2.16220625480307));
#59910=CARTESIAN_POINT('Ctrl Pts',(37.4161633089293,7.99080313186483,6.80170544581863));
#59911=CARTESIAN_POINT('Ctrl Pts',(37.5349683449095,3.77470409044336,9.79120731541779));
#59912=CARTESIAN_POINT('Ctrl Pts',(37.6537733808897,-1.35708465380123,10.4055010886702));
#59913=CARTESIAN_POINT('Ctrl Pts',(37.77257841687,-6.15966389881867,8.49556780430181));
#59914=CARTESIAN_POINT('Ctrl Pts',(37.887258179598,-9.35312061795756,4.66260979642269));
#59915=CARTESIAN_POINT('Ctrl Pts',(37.962336263666,-10.0679489640148,1.49574877226827));
#59916=CARTESIAN_POINT('Ctrl Pts',(37.9978126690739,-10.0691207289378,-0.000166380613864248));
#59917=CARTESIAN_POINT('Origin',(-2.04781266907391,0.,0.));
#59918=CARTESIAN_POINT('',(34.7021873309261,-10.068895619793,0.000223893809893075));
#59919=CARTESIAN_POINT('',(34.9978126690739,-10.0679217181859,-0.000196888195062583));
#59920=CARTESIAN_POINT('',(-2.04781266907391,-10.0685,8.88799240754737E-13));
#59921=CARTESIAN_POINT('Ctrl Pts',(34.7021873309266,-10.0688956197921,0.000223893809892864));
#59922=CARTESIAN_POINT('Ctrl Pts',(34.7357313998079,-10.0675280608373,-1.41430270099979));
#59923=CARTESIAN_POINT('Ctrl Pts',(34.8089635096389,-9.41060872960074,-4.503672201116));
#59924=CARTESIAN_POINT('Ctrl Pts',(34.9218836604196,-6.35621225475712,-8.35191894126176));
#59925=CARTESIAN_POINT('Ctrl Pts',(35.0409477832688,-1.58710704615101,-10.3748289360832));
#59926=CARTESIAN_POINT('Ctrl Pts',(35.160011906118,3.56865391342995,-9.87019217011967));
#59927=CARTESIAN_POINT('Ctrl Pts',(35.2790760289672,7.85500876570816,-6.96094975700724));
#59928=CARTESIAN_POINT('Ctrl Pts',(35.3981401518164,10.227702960638,-2.35586000812625));
#59929=CARTESIAN_POINT('Ctrl Pts',(35.5172042746655,10.1086936636169,2.82317138057241));
#59930=CARTESIAN_POINT('Ctrl Pts',(35.6362683975148,7.52697427444376,7.3144133394821));
#59931=CARTESIAN_POINT('Ctrl Pts',(35.755332520364,3.11151096880807,10.0236961107128));
#59932=CARTESIAN_POINT('Ctrl Pts',(35.8743966432131,-2.06198791686537,10.2909761470733));
#59933=CARTESIAN_POINT('Ctrl Pts',(35.9934607660623,-6.73313915785387,8.05113788913754));
#59934=CARTESIAN_POINT('Ctrl Pts',(36.1027243286335,-9.51446751276782,4.19567865163804));
#59935=CARTESIAN_POINT('Ctrl Pts',(36.1722998502549,-10.0671392532912,1.26024373135914));
#59936=CARTESIAN_POINT('Ctrl Pts',(36.2021873309266,-10.0684139656555,-0.000261209358190344));
#59937=CARTESIAN_POINT('Ctrl Pts',(34.9978126690739,-10.0679217181859,-0.000196888195062028));
#59938=CARTESIAN_POINT('Ctrl Pts',(35.0118959758242,-10.0683425077228,-0.594244039820875));
#59939=CARTESIAN_POINT('Ctrl Pts',(35.0655809612345,-9.87117700447691,-2.85845118017994));
#59940=CARTESIAN_POINT('Ctrl Pts',(35.158867625305,-8.19490040588757,-6.55436793302628));
#59941=CARTESIAN_POINT('Ctrl Pts',(35.2776726612852,-4.07211517951482,-9.67129823905069));
#59942=CARTESIAN_POINT('Ctrl Pts',(35.3964776972655,1.03850746384432,-10.4421086908459));
#59943=CARTESIAN_POINT('Ctrl Pts',(35.5152827332456,5.89720291816771,-8.67981159967508));
#59944=CARTESIAN_POINT('Ctrl Pts',(35.6340877692259,9.3253205422193,-4.81191525785339));
#59945=CARTESIAN_POINT('Ctrl Pts',(35.7528928052061,10.4912475967761,0.223283512688066));
#59946=CARTESIAN_POINT('Ctrl Pts',(35.8716978411863,9.11214670637266,5.20431686827785));
#59947=CARTESIAN_POINT('Ctrl Pts',(35.9905028771666,5.5225681971373,8.92285672707276));
#59948=CARTESIAN_POINT('Ctrl Pts',(36.1093079131468,0.593292930198467,10.4768380326736));
#59949=CARTESIAN_POINT('Ctrl Pts',(36.2281129491271,-4.47990679119387,9.48928694929787));
#59950=CARTESIAN_POINT('Ctrl Pts',(36.3469179851072,-8.46634463138618,6.19976937042805));
#59951=CARTESIAN_POINT('Ctrl Pts',(36.4368178917562,-9.92876240170465,2.57252717221098));
#59952=CARTESIAN_POINT('Ctrl Pts',(36.4871161197451,-10.0687339336306,0.451396484673442));
#59953=CARTESIAN_POINT('Ctrl Pts',(36.4978126690739,-10.0682971267649,0.000254225486309226));
#59954=CARTESIAN_POINT('Origin',(-2.04781266907391,0.,0.));
#59955=CARTESIAN_POINT('',(33.2021873309261,-10.0676826490326,-8.66471596138184E-5));
#59956=CARTESIAN_POINT('',(33.4978126690739,-10.0693470076013,3.26837738548989E-5));
#59957=CARTESIAN_POINT('',(-2.04781266907391,-10.0685,8.88799240754737E-13));
#59958=CARTESIAN_POINT('Ctrl Pts',(33.2021873309266,-10.0676826490317,-8.66471596133733E-5));
#59959=CARTESIAN_POINT('Ctrl Pts',(33.2197868674614,-10.0679062728494,-0.742502004871305));
#59960=CARTESIAN_POINT('Ctrl Pts',(33.2770744449459,-9.80418147022253,-3.158953361154));
#59961=CARTESIAN_POINT('Ctrl Pts',(33.3740500633801,-7.89130690893979,-6.9197730813843));
#59962=CARTESIAN_POINT('Ctrl Pts',(33.4931141862293,-3.62022593454477,-9.85139322186365));
#59963=CARTESIAN_POINT('Ctrl Pts',(33.6121783090785,1.53282527671301,-10.3829875710222));
#59964=CARTESIAN_POINT('Ctrl Pts',(33.7312424319277,6.31244502352206,-8.38504752842475));
#59965=CARTESIAN_POINT('Ctrl Pts',(33.8503065547769,9.55420809142776,-4.34431720465111));
#59966=CARTESIAN_POINT('Ctrl Pts',(33.9693706776261,10.4683464956279,0.754788630283966));
#59967=CARTESIAN_POINT('Ctrl Pts',(34.0884348004753,8.83215511233873,5.67001060850159));
#59968=CARTESIAN_POINT('Ctrl Pts',(34.2074989233245,5.044247765107,9.20388769559607));
#59969=CARTESIAN_POINT('Ctrl Pts',(34.3265630461737,0.0274457365422501,
10.495486218393));
#59970=CARTESIAN_POINT('Ctrl Pts',(34.4456271690228,-4.99604270419572,9.23014309351612));
#59971=CARTESIAN_POINT('Ctrl Pts',(34.5646912918721,-8.80238032427643,5.71612498601302));
#59972=CARTESIAN_POINT('Ctrl Pts',(34.6502113458399,-9.99605376034515,2.19186868835956));
#59973=CARTESIAN_POINT('Ctrl Pts',(34.6960433588581,-10.0691461035379,0.25931028906438));
#59974=CARTESIAN_POINT('Ctrl Pts',(34.7021873309266,-10.0688956197921,0.000223893809892864));
#59975=CARTESIAN_POINT('Ctrl Pts',(33.4978126690739,-10.0693470076013,3.26837738548599E-5));
#59976=CARTESIAN_POINT('Ctrl Pts',(33.5366758319033,-10.0690425640898,-1.63858314297772));
#59977=CARTESIAN_POINT('Ctrl Pts',(33.6151406733927,-9.24531483550623,-4.94724837940332));
#59978=CARTESIAN_POINT('Ctrl Pts',(33.7332071935423,-5.79263042786231,-8.74994653641399));
#59979=CARTESIAN_POINT('Ctrl Pts',(33.8520122295224,-0.913139167682674,
-10.4538178922508));
#59980=CARTESIAN_POINT('Ctrl Pts',(33.9708172655027,4.18786671008217,-9.62174121884839));
#59981=CARTESIAN_POINT('Ctrl Pts',(34.0896223014829,8.27295549041769,-6.45556652180641));
#59982=CARTESIAN_POINT('Ctrl Pts',(34.2084273374631,10.3511425446899,-1.72336289951095));
#59983=CARTESIAN_POINT('Ctrl Pts',(34.3272323734434,9.91828915353406,3.42690413212689));
#59984=CARTESIAN_POINT('Ctrl Pts',(34.4460374094236,7.07939941359363,7.74585280048044));
#59985=CARTESIAN_POINT('Ctrl Pts',(34.5648424454038,2.52314773219355,10.1857673832376));
#59986=CARTESIAN_POINT('Ctrl Pts',(34.6836474813841,-2.64518382135331,10.1547591904067));
#59987=CARTESIAN_POINT('Ctrl Pts',(34.8024525173643,-7.17183127748453,7.6603503700023));
#59988=CARTESIAN_POINT('Ctrl Pts',(34.9071742465942,-9.62833570822918,3.82362412601771));
#59989=CARTESIAN_POINT('Ctrl Pts',(34.9722942971641,-10.0671592648723,1.07619208890588));
#59990=CARTESIAN_POINT('Ctrl Pts',(34.9978126690739,-10.0679217181859,-0.000196888195062028));
#59991=CARTESIAN_POINT('Origin',(-2.04781266907391,0.,0.));
#59992=CARTESIAN_POINT('',(31.7021873309261,-10.0693203618692,-7.29422645144902E-5));
#59993=CARTESIAN_POINT('',(31.9978126690739,-10.0678007494847,0.000154563734536262));
#59994=CARTESIAN_POINT('',(-2.04781266907391,-10.0685,8.88799240754737E-13));
#59995=CARTESIAN_POINT('Ctrl Pts',(31.7021873309266,-10.0693203618683,-7.29422645155079E-5));
#59996=CARTESIAN_POINT('Ctrl Pts',(31.7038423351149,-10.0693475392072,-0.0698546177573546));
#59997=CARTESIAN_POINT('Ctrl Pts',(31.7451853802529,-10.0516047861332,-1.81303088400049));
#59998=CARTESIAN_POINT('Ctrl Pts',(31.8262164663406,-9.1106548690145,-5.21075350468951));
#59999=CARTESIAN_POINT('Ctrl Pts',(31.9452805891898,-5.50849247035029,-8.93378390901784));
#60000=CARTESIAN_POINT('Ctrl Pts',(32.064344712039,-0.564334710989629,-10.4803392389227));
#60001=CARTESIAN_POINT('Ctrl Pts',(32.1834088348883,4.51730795337978,-9.47364307345718));
#60002=CARTESIAN_POINT('Ctrl Pts',(32.3024729577373,8.49843058456348,-6.1589497341906));
#60003=CARTESIAN_POINT('Ctrl Pts',(32.4215370805866,10.409140216352,-1.34379469609559));
#60004=CARTESIAN_POINT('Ctrl Pts',(32.5406012034357,9.7839440709481,3.79873961275201));
#60005=CARTESIAN_POINT('Ctrl Pts',(32.659665326285,6.7751542974874,8.01581365016488));
#60006=CARTESIAN_POINT('Ctrl Pts',(32.7787294491341,2.1157812321061,10.2800512647943));
#60007=CARTESIAN_POINT('Ctrl Pts',(32.8977935719833,-3.05904476581843,10.0398321375235));
#60008=CARTESIAN_POINT('Ctrl Pts',(33.0168576948326,-7.48861715651959,7.35367916841708));
#60009=CARTESIAN_POINT('Ctrl Pts',(33.1183222811469,-9.70870503508644,3.53787171211958));
#60010=CARTESIAN_POINT('Ctrl Pts',(33.1800988265117,-10.0674019873407,0.931690441069841));
#60011=CARTESIAN_POINT('Ctrl Pts',(33.2021873309266,-10.0676826490317,-8.66471596133733E-5));
#60012=CARTESIAN_POINT('Ctrl Pts',(31.9978126690739,-10.0678007494847,0.00015456373453536));
#60013=CARTESIAN_POINT('Ctrl Pts',(32.0218540093223,-10.0672458119022,-1.01396673139942));
#60014=CARTESIAN_POINT('Ctrl Pts',(32.0854970282308,-9.66400610463595,-3.69901318249289));
#60015=CARTESIAN_POINT('Ctrl Pts',(32.1887417257993,-7.31277097856737,-7.52592268621747));
#60016=CARTESIAN_POINT('Ctrl Pts',(32.3075467617795,-2.83319911559344,-10.1039157971204));
#60017=CARTESIAN_POINT('Ctrl Pts',(32.4263517977597,2.33366668990814,-10.2308421669144));
#60018=CARTESIAN_POINT('Ctrl Pts',(32.5451568337399,6.93441803807263,-7.87591125757227));
#60019=CARTESIAN_POINT('Ctrl Pts',(32.6639618697202,9.85297787124923,-3.61039592462831));
#60020=CARTESIAN_POINT('Ctrl Pts',(32.7827669057004,10.3813449468827,1.53095027931453));
#60021=CARTESIAN_POINT('Ctrl Pts',(32.9015719416806,8.39134490245989,6.30090964796831));
#60022=CARTESIAN_POINT('Ctrl Pts',(33.0203769776609,4.36572353887912,9.54235765657405));
#60023=CARTESIAN_POINT('Ctrl Pts',(33.1391820136411,-0.71896046753108,10.4689649684211));
#60024=CARTESIAN_POINT('Ctrl Pts',(33.2579870496213,-5.6292348563709,8.85594978507207));
#60025=CARTESIAN_POINT('Ctrl Pts',(33.3767920856015,-9.17393666806451,5.09460672419782));
#60026=CARTESIAN_POINT('Ctrl Pts',(33.4567339587524,-10.0616271779199,1.73206137024705));
#60027=CARTESIAN_POINT('Ctrl Pts',(33.4970741532432,-10.0693527929347,0.031171264383115));
#60028=CARTESIAN_POINT('Ctrl Pts',(33.4978126690739,-10.0693470076013,3.26837738548599E-5));
#60029=CARTESIAN_POINT('Origin',(-2.04781266907391,0.,0.));
#60030=CARTESIAN_POINT('',(30.2021873309261,-10.0679004225068,0.000194472203930257));
#60031=CARTESIAN_POINT('',(30.4978126690739,-10.0684882089047,-0.000258245171450011));
#60032=CARTESIAN_POINT('',(-2.04781266907391,-10.0685,8.88799240754737E-13));
#60033=CARTESIAN_POINT('Ctrl Pts',(30.2021873309266,-10.067900422506,0.000194472203929666));
#60034=CARTESIAN_POINT('Ctrl Pts',(30.2275858437181,-10.067155705448,-1.07114500493766));
#60035=CARTESIAN_POINT('Ctrl Pts',(30.2926723974594,-9.63073097165002,-3.81716565313784));
#60036=CARTESIAN_POINT('Ctrl Pts',(30.3974469921503,-7.17635339944174,-7.65871634905305));
#60037=CARTESIAN_POINT('Ctrl Pts',(30.5165111149995,-2.63891455811226,-10.158351942314));
#60038=CARTESIAN_POINT('Ctrl Pts',(30.6355752378487,2.54142451650656,-10.1831795454971));
#60039=CARTESIAN_POINT('Ctrl Pts',(30.7546393606979,7.10261417246512,-7.72715058388468));
#60040=CARTESIAN_POINT('Ctrl Pts',(30.8737034835471,9.9334437853503,-3.38861015642353));
#60041=CARTESIAN_POINT('Ctrl Pts',(30.9927676063963,10.3442582039821,1.77547358140902));
#60042=CARTESIAN_POINT('Ctrl Pts',(31.1118317292455,8.23497359473827,6.50701115128098));
#60043=CARTESIAN_POINT('Ctrl Pts',(31.2308958520947,4.11946016352903,9.65329126205301));
#60044=CARTESIAN_POINT('Ctrl Pts',(31.3499599749439,-0.99964843601095,10.4478077716482));
#60045=CARTESIAN_POINT('Ctrl Pts',(31.4690240977931,-5.87521970284595,8.69699819893175));
#60046=CARTESIAN_POINT('Ctrl Pts',(31.5864332164539,-9.27157721963363,4.88118782621643));
#60047=CARTESIAN_POINT('Ctrl Pts',(31.6641542941652,-10.0686958095333,1.60355383288915));
#60048=CARTESIAN_POINT('Ctrl Pts',(31.7021873309266,-10.0693203618683,-7.29422645155079E-5));
#60049=CARTESIAN_POINT('Ctrl Pts',(30.4978126690739,-10.0684882089047,-0.000258245171449525));
#60050=CARTESIAN_POINT('Ctrl Pts',(30.5070321867413,-10.068884093533,-0.389083362395765));
#60051=CARTESIAN_POINT('Ctrl Pts',(30.5558533830688,-9.95188099980351,-2.44783790530016));
#60052=CARTESIAN_POINT('Ctrl Pts',(30.6442762580563,-8.57995317261452,-6.04156728172768));
#60053=CARTESIAN_POINT('Ctrl Pts',(30.7630812940366,-4.65525498345498,-9.40450597867413));
#60054=CARTESIAN_POINT('Ctrl Pts',(30.8818863300168,0.398742072642834,-10.4860448417601));
#60055=CARTESIAN_POINT('Ctrl Pts',(31.000691365997,5.35600995441259,-9.0238178744993));
#60056=CARTESIAN_POINT('Ctrl Pts',(31.1194964019772,9.01398574706474,-5.37254061088553));
#60057=CARTESIAN_POINT('Ctrl Pts',(31.2383014379574,10.4852963781011,-0.417961155229236));
#60058=CARTESIAN_POINT('Ctrl Pts',(31.3571064739377,9.4130227454641,4.63800975174425));
#60059=CARTESIAN_POINT('Ctrl Pts',(31.4759115099179,6.05728323207572,8.56886524052714));
#60060=CARTESIAN_POINT('Ctrl Pts',(31.5947165458981,1.23213267353085,10.4210354926331));
#60061=CARTESIAN_POINT('Ctrl Pts',(31.7135215818784,-3.89191580512397,9.74521026092953));
#60062=CARTESIAN_POINT('Ctrl Pts',(31.8323266178586,-8.07184068054606,6.70533516625238));
#60063=CARTESIAN_POINT('Ctrl Pts',(31.9270903135904,-9.84404668401735,2.98315077148792));
#60064=CARTESIAN_POINT('Ctrl Pts',(31.9822523306622,-10.0681599231618,0.656526894883811));
#60065=CARTESIAN_POINT('Ctrl Pts',(31.9978126690739,-10.0678007494847,0.00015456373453536));
#60066=CARTESIAN_POINT('Origin',(-2.04781266907391,0.,0.));
#60067=CARTESIAN_POINT('',(28.7021873309261,-10.0684596617401,-0.000261386783779813));
#60068=CARTESIAN_POINT('',(28.9978126690739,-10.0689565675435,0.000209149011081849));
#60069=CARTESIAN_POINT('',(-2.04781266907391,-10.0685,8.88799240754737E-13));
#60070=CARTESIAN_POINT('Ctrl Pts',(28.7021873309266,-10.0684596617392,-0.000261386783779911));
#60071=CARTESIAN_POINT('Ctrl Pts',(28.7116413113716,-10.0688665726457,-0.398977947764452));
#60072=CARTESIAN_POINT('Ctrl Pts',(28.7607833327664,-9.94809636912126,-2.47127140545957));
#60073=CARTESIAN_POINT('Ctrl Pts',(28.8496133951108,-8.55707432906648,-6.07720850027072));
#60074=CARTESIAN_POINT('Ctrl Pts',(28.96867751796,-4.60790624887834,-9.42990902556751));
#60075=CARTESIAN_POINT('Ctrl Pts',(29.0877416408092,0.463853691388278,-10.4852669962151));
#60076=CARTESIAN_POINT('Ctrl Pts',(29.2068057636584,5.42260821225282,-8.98617295656719));
#60077=CARTESIAN_POINT('Ctrl Pts',(29.3258698865076,9.060290751466,-5.29784066651983));
#60078=CARTESIAN_POINT('Ctrl Pts',(29.4449340093568,10.490678242084,-0.318832636340938));
#60079=CARTESIAN_POINT('Ctrl Pts',(29.563998132206,9.36529541855293,4.73785035138961));
#60080=CARTESIAN_POINT('Ctrl Pts',(29.6830622550552,5.95831139997658,8.64028410932423));
#60081=CARTESIAN_POINT('Ctrl Pts',(29.8021263779044,1.09974579181068,10.4377460891864));
#60082=CARTESIAN_POINT('Ctrl Pts',(29.9211905007536,-4.02674316534753,9.69233324382));
#60083=CARTESIAN_POINT('Ctrl Pts',(30.0402546236027,-8.17222494573302,6.58564527326446));
#60084=CARTESIAN_POINT('Ctrl Pts',(30.1339202336604,-9.86716290004697,2.87950542203976));
#60085=CARTESIAN_POINT('Ctrl Pts',(30.1878978027684,-10.0683194098481,0.602943765097816));
#60086=CARTESIAN_POINT('Ctrl Pts',(30.2021873309266,-10.067900422506,0.000194472203929666));
#60087=CARTESIAN_POINT('Ctrl Pts',(28.9978126690739,-10.0689565675435,0.000209149011081503));
#60088=CARTESIAN_POINT('Ctrl Pts',(29.0318120428204,-10.0676299920431,-1.43349243230001));
#60089=CARTESIAN_POINT('Ctrl Pts',(29.105413095227,-9.39783976794824,-4.53833595468961));
#60090=CARTESIAN_POINT('Ctrl Pts',(29.2186158262936,-6.31627946473417,-8.37978194151124));
#60091=CARTESIAN_POINT('Ctrl Pts',(29.3374208622738,-1.54997555683656,-10.378521447543));
#60092=CARTESIAN_POINT('Ctrl Pts',(29.456225898254,3.59233044897795,-9.85957877443276));
#60093=CARTESIAN_POINT('Ctrl Pts',(29.5750309342343,7.8631880120934,-6.94884205824041));
#60094=CARTESIAN_POINT('Ctrl Pts',(29.6938359702145,10.2265476305979,-2.35241476423973));
#60095=CARTESIAN_POINT('Ctrl Pts',(29.8126410061947,10.1090917635981,2.81467500416174));
#60096=CARTESIAN_POINT('Ctrl Pts',(29.9314460421749,7.53931353939529,7.29896451687431));
#60097=CARTESIAN_POINT('Ctrl Pts',(30.0502510781552,3.14060472647248,10.0126287065864));
#60098=CARTESIAN_POINT('Ctrl Pts',(30.1690561141354,-2.01997027245138,10.2973711092838));
#60099=CARTESIAN_POINT('Ctrl Pts',(30.2878611501157,-6.69052911800965,8.08411725452847));
#60100=CARTESIAN_POINT('Ctrl Pts',(30.3974466684284,-9.50156567969192,4.23370908453169));
#60101=CARTESIAN_POINT('Ctrl Pts',(30.4674305080812,-10.0671836037243,1.28108289822459));
#60102=CARTESIAN_POINT('Ctrl Pts',(30.4978126690739,-10.0684882089047,-0.000258245171449525));
#60103=CARTESIAN_POINT('Origin',(-2.04781266907391,0.,0.));
#60104=CARTESIAN_POINT('',(27.2021873309261,-10.0688518142443,0.000231103861848507));
#60105=CARTESIAN_POINT('',(27.4978126690739,-10.0676494950024,-2.42588443044589E-5));
#60106=CARTESIAN_POINT('',(-2.04781266907391,-10.0685,8.88799240754737E-13));
#60107=CARTESIAN_POINT('Ctrl Pts',(27.2021873309266,-10.0688518142434,0.00023110386184827));
#60108=CARTESIAN_POINT('Ctrl Pts',(27.2353848199749,-10.0674720042622,-1.3996980849141));
#60109=CARTESIAN_POINT('Ctrl Pts',(27.3082703499728,-9.42081087010833,-4.47449599460339));
#60110=CARTESIAN_POINT('Ctrl Pts',(27.4208439209205,-6.39252655710521,-8.32415692101224));
#60111=CARTESIAN_POINT('Ctrl Pts',(27.5399080437697,-1.63227683129287,-10.3678183131726));
#60112=CARTESIAN_POINT('Ctrl Pts',(27.6589721666189,3.5256330432367,-9.88564089340539));
#60113=CARTESIAN_POINT('Ctrl Pts',(27.7780362894681,7.82461768313833,-6.99509416245773));
#60114=CARTESIAN_POINT('Ctrl Pts',(27.8971004123173,10.2173456318464,-2.40038173387489));
#60115=CARTESIAN_POINT('Ctrl Pts',(28.0161645351665,10.120893371927,2.77911885010604));
#60116=CARTESIAN_POINT('Ctrl Pts',(28.1352286580157,7.55875889054041,7.28156221312484));
#60117=CARTESIAN_POINT('Ctrl Pts',(28.2542927808649,3.1551370297433,10.0100496778225));
#60118=CARTESIAN_POINT('Ctrl Pts',(28.3733569037141,-2.01714872213973,10.2998589923213));
#60119=CARTESIAN_POINT('Ctrl Pts',(28.4924210265632,-6.69801068765711,8.08038594727766));
#60120=CARTESIAN_POINT('Ctrl Pts',(28.6020311689674,-9.50497954746825,4.2248857891727));
#60121=CARTESIAN_POINT('Ctrl Pts',(28.6719532704219,-10.0671583507159,1.27484391928936));
#60122=CARTESIAN_POINT('Ctrl Pts',(28.7021873309266,-10.0684596617392,-0.000261386783779911));
#60123=CARTESIAN_POINT('Ctrl Pts',(27.4978126690739,-10.0676494950024,-2.42588443043895E-5));
#60124=CARTESIAN_POINT('Ctrl Pts',(27.5169902202394,-10.0677176760758,-0.80901407167683));
#60125=CARTESIAN_POINT('Ctrl Pts',(27.5757694500649,-9.77235830881682,-3.28852040506986));
#60126=CARTESIAN_POINT('Ctrl Pts',(27.6741503585506,-7.75881554014436,-7.06519023649855));
#60127=CARTESIAN_POINT('Ctrl Pts',(27.7929553945308,-3.44507749523718,-9.91199135974755));
#60128=CARTESIAN_POINT('Ctrl Pts',(27.9117604305111,1.70438751322266,-10.3542838897082));
#60129=CARTESIAN_POINT('Ctrl Pts',(28.0305654664913,6.44039227206198,-8.28477392847046));
#60130=CARTESIAN_POINT('Ctrl Pts',(28.1493705024715,9.61404916352834,-4.20549525563395));
#60131=CARTESIAN_POINT('Ctrl Pts',(28.2681755384518,10.4554740149348,0.893976949883643));
#60132=CARTESIAN_POINT('Ctrl Pts',(28.386980574432,8.7605490852157,5.77658302021413));
#60133=CARTESIAN_POINT('Ctrl Pts',(28.5057856104122,4.94043913537346,9.25787193763072));
#60134=CARTESIAN_POINT('Ctrl Pts',(28.6245906463924,-0.0781513139439594,
10.4933323608865));
#60135=CARTESIAN_POINT('Ctrl Pts',(28.7433956823727,-5.07778336235737,9.18325910496195));
#60136=CARTESIAN_POINT('Ctrl Pts',(28.8622007183529,-8.84561714879615,5.64545737038407));
#60137=CARTESIAN_POINT('Ctrl Pts',(28.9470063805866,-10.0034455159759,2.14251119997342));
#60138=CARTESIAN_POINT('Ctrl Pts',(28.9922103641603,-10.0691751562887,0.236449777250179));
#60139=CARTESIAN_POINT('Ctrl Pts',(28.9978126690739,-10.0689565675435,0.000209149011081503));
#60140=CARTESIAN_POINT('Origin',(-2.04781266907391,0.,0.));
#60141=CARTESIAN_POINT('',(25.7021873309261,-10.0676972542269,-9.94107447664056E-5));
#60142=CARTESIAN_POINT('',(25.9978126690739,-10.0690970093708,-0.000173820672795255));
#60143=CARTESIAN_POINT('',(-2.04781266907391,-10.0685,8.88799240754737E-13));
#60144=CARTESIAN_POINT('Ctrl Pts',(25.7021873309266,-10.0676972542261,-9.94107447663956E-5));
#60145=CARTESIAN_POINT('Ctrl Pts',(25.7194402876284,-10.0679492143918,-0.727891692702293));
#60146=CARTESIAN_POINT('Ctrl Pts',(25.7763812852798,-9.81106868289854,-3.1296942575133));
#60147=CARTESIAN_POINT('Ctrl Pts',(25.873010323881,-7.92136931787451,-6.88533894291106));
#60148=CARTESIAN_POINT('Ctrl Pts',(25.9920744467302,-3.66309675088932,-9.83553284893887));
#60149=CARTESIAN_POINT('Ctrl Pts',(26.1111385695794,1.48759036906762,-10.3895649149899));
#60150=CARTESIAN_POINT('Ctrl Pts',(26.2302026924286,6.27586628765668,-8.41246019713529));
#60151=CARTESIAN_POINT('Ctrl Pts',(26.3492668152778,9.53519694804324,-4.38588684201477));
#60152=CARTESIAN_POINT('Ctrl Pts',(26.468330938127,10.4715344961624,0.709189343272753));
#60153=CARTESIAN_POINT('Ctrl Pts',(26.5873950609762,8.85676558659625,5.63149070611111));
#60154=CARTESIAN_POINT('Ctrl Pts',(26.7064591838254,5.08428503596618,9.18183151130437));
#60155=CARTESIAN_POINT('Ctrl Pts',(26.8255233066746,0.0731558046942684,
10.4952671455838));
#60156=CARTESIAN_POINT('Ctrl Pts',(26.9445874295238,-4.95579586185122,9.25181450336041));
#60157=CARTESIAN_POINT('Ctrl Pts',(27.063651552373,-8.77740176347816,5.75440722502514));
#60158=CARTESIAN_POINT('Ctrl Pts',(27.1495181861739,-9.99131250574906,2.22112183309714));
#60159=CARTESIAN_POINT('Ctrl Pts',(27.1956967790251,-10.0691215854989,0.273935932711093));
#60160=CARTESIAN_POINT('Ctrl Pts',(27.2021873309266,-10.0688518142434,0.00023110386184827));
#60161=CARTESIAN_POINT('Ctrl Pts',(25.9978126690739,-10.0690970093708,-0.000173820672795012));
#60162=CARTESIAN_POINT('Ctrl Pts',(26.0021683976584,-10.0692457578938,-0.183840818186473));
#60163=CARTESIAN_POINT('Ctrl Pts',(26.046125804903,-10.0195685915622,-2.03730218398405));
#60164=CARTESIAN_POINT('Ctrl Pts',(26.1296848908076,-8.93296399143784,-5.50620431800117));
#60165=CARTESIAN_POINT('Ctrl Pts',(26.2484899267879,-5.22100967646791,-9.10259246710126));
#60166=CARTESIAN_POINT('Ctrl Pts',(26.3672949627681,-0.242512426070257,
-10.4908207203775));
#60167=CARTESIAN_POINT('Ctrl Pts',(26.4860999987483,4.79481490108,-9.33412458285624));
#60168=CARTESIAN_POINT('Ctrl Pts',(26.6049050347286,8.66898810365204,-5.91310214038614));
#60169=CARTESIAN_POINT('Ctrl Pts',(26.7237100707088,10.4401876822764,-1.05764494171864));
#60170=CARTESIAN_POINT('Ctrl Pts',(26.842515106689,9.67874572738195,4.05438192682752));
#60171=CARTESIAN_POINT('Ctrl Pts',(26.9613201426693,6.56937726316331,8.18287321410596));
#60172=CARTESIAN_POINT('Ctrl Pts',(27.0801251786495,1.86637100119828,10.3263154585644));
#60173=CARTESIAN_POINT('Ctrl Pts',(27.1989302146297,-3.28939040832167,9.96473995674454));
#60174=CARTESIAN_POINT('Ctrl Pts',(27.3177352506099,-7.64719233458281,7.18585979975938));
#60175=CARTESIAN_POINT('Ctrl Pts',(27.4173627354247,-9.74590684403498,3.39374572626348));
#60176=CARTESIAN_POINT('Ctrl Pts',(27.4773885415793,-10.067576882033,0.861551389501777));
#60177=CARTESIAN_POINT('Ctrl Pts',(27.4978126690739,-10.0676494950024,-2.42588443043895E-5));
#60178=CARTESIAN_POINT('Origin',(-2.04781266907391,0.,0.));
#60179=CARTESIAN_POINT('',(24.2021873309261,-10.0693361365595,-5.80152907239285E-5));
#60180=CARTESIAN_POINT('',(24.4978126690739,-10.0683262561367,0.000255752892879269));
#60181=CARTESIAN_POINT('',(-2.04781266907391,-10.0685,8.88799240754737E-13));
#60182=CARTESIAN_POINT('Ctrl Pts',(24.2021873309266,-10.0693361365586,-5.80152907240453E-5));
#60183=CARTESIAN_POINT('Ctrl Pts',(24.2034957552819,-10.0693535941416,-0.0552262305921217));
#60184=CARTESIAN_POINT('Ctrl Pts',(24.2444922205868,-10.0554444077902,-1.7837864332911));
#60185=CARTESIAN_POINT('Ctrl Pts',(24.3251767268415,-9.13326252848837,-5.17102502552844));
#60186=CARTESIAN_POINT('Ctrl Pts',(24.4442408496907,-5.54734897230373,-8.90970839076184));
#60187=CARTESIAN_POINT('Ctrl Pts',(24.5633049725399,-0.609973718555534,
-10.4777820311172));
#60188=CARTESIAN_POINT('Ctrl Pts',(24.6823690953891,4.47600515130988,-9.49322717069275));
#60189=CARTESIAN_POINT('Ctrl Pts',(24.8014332182383,8.47152629978549,-6.19590400030329));
#60190=CARTESIAN_POINT('Ctrl Pts',(24.9204973410875,10.4031889509458,-1.38911622258575));
#60191=CARTESIAN_POINT('Ctrl Pts',(25.0395614639367,9.80039568993721,3.7560921913062));
#60192=CARTESIAN_POINT('Ctrl Pts',(25.1586255867859,6.81000080839887,7.98623022574092));
#60193=CARTESIAN_POINT('Ctrl Pts',(25.2776897096351,2.16053322404739,10.2707390394615));
#60194=CARTESIAN_POINT('Ctrl Pts',(25.3967538324842,-3.01528990656447,10.0530597833845));
#60195=CARTESIAN_POINT('Ctrl Pts',(25.5158179553335,-7.45651911923148,7.38622412694516));
#60196=CARTESIAN_POINT('Ctrl Pts',(25.6176291214809,-9.70084469419126,3.56712109339173));
#60197=CARTESIAN_POINT('Ctrl Pts',(25.6797522466786,-10.0673696148745,0.946293804228947));
#60198=CARTESIAN_POINT('Ctrl Pts',(25.7021873309266,-10.0676972542261,-9.94107447663956E-5));
#60199=CARTESIAN_POINT('Ctrl Pts',(24.4978126690739,-10.0683262561367,0.000255752892878991));
#60200=CARTESIAN_POINT('Ctrl Pts',(24.5269482537375,-10.0671233553105,-1.22856896434762));
#60201=CARTESIAN_POINT('Ctrl Pts',(24.5956855170611,-9.53543141724821,-4.1286496216628));
#60202=CARTESIAN_POINT('Ctrl Pts',(24.704024459045,-6.81634027291969,-7.97832294079858));
#60203=CARTESIAN_POINT('Ctrl Pts',(24.8228294950251,-2.18102354189972,-10.2644662780672));
#60204=CARTESIAN_POINT('Ctrl Pts',(24.9416345310054,2.98337858259214,-10.0605956034834));
#60205=CARTESIAN_POINT('Ctrl Pts',(25.0604395669856,7.42405535477923,-7.41616705266769));
#60206=CARTESIAN_POINT('Ctrl Pts',(25.1792446029658,10.063761539955,-2.9726815051098));
#60207=CARTESIAN_POINT('Ctrl Pts',(25.2980496389461,10.2621418375906,2.19193443539551));
#60208=CARTESIAN_POINT('Ctrl Pts',(25.4168546749263,7.97107199968254,6.82481815433765));
#60209=CARTESIAN_POINT('Ctrl Pts',(25.5356597109065,3.74633309111811,9.80209773641814));
#60210=CARTESIAN_POINT('Ctrl Pts',(25.6544647468867,-1.38721311801518,10.4015273603979));
#60211=CARTESIAN_POINT('Ctrl Pts',(25.773269782867,-6.18424108959879,8.47769389690486));
#60212=CARTESIAN_POINT('Ctrl Pts',(25.8877190902627,-9.36018914116762,4.64322485922857));
#60213=CARTESIAN_POINT('Ctrl Pts',(25.9625667189983,-10.0678933570043,1.48603398573513));
#60214=CARTESIAN_POINT('Ctrl Pts',(25.9978126690739,-10.0690970093708,-0.000173820672795012));
#60215=CARTESIAN_POINT('Origin',(-2.04781266907391,0.,0.));
#60216=CARTESIAN_POINT('',(22.7021873309261,-10.067869906259,0.000184994001410302));
#60217=CARTESIAN_POINT('',(22.9978126690739,-10.0679008419791,-0.000190872912599893));
#60218=CARTESIAN_POINT('',(-2.04781266907391,-10.0685,8.88799240754737E-13));
#60219=CARTESIAN_POINT('Ctrl Pts',(22.7021873309266,-10.0678699062581,0.000184994001410643));
#60220=CARTESIAN_POINT('Ctrl Pts',(22.7272392638851,-10.0671739860671,-1.05654450902642));
#60221=CARTESIAN_POINT('Ctrl Pts',(22.7919792377933,-9.63920097314283,-3.78792789189713));
#60222=CARTESIAN_POINT('Ctrl Pts',(22.8964072526512,-7.20964086201644,-7.62738899425446));
#60223=CARTESIAN_POINT('Ctrl Pts',(23.0154713755005,-2.68313155923512,-10.1467625016439));
#60224=CARTESIAN_POINT('Ctrl Pts',(23.1345354983496,2.49705025449416,-10.1941514730488));
#60225=CARTESIAN_POINT('Ctrl Pts',(23.2535996211988,7.06889323958863,-7.75801086595204));
#60226=CARTESIAN_POINT('Ctrl Pts',(23.372663744048,9.91859137582519,-3.43184051907101));
#60227=CARTESIAN_POINT('Ctrl Pts',(23.4917278668972,10.3518927061033,1.73040504803268));
#60228=CARTESIAN_POINT('Ctrl Pts',(23.6107919897464,8.26323506833476,6.47108417766095));
#60229=CARTESIAN_POINT('Ctrl Pts',(23.7298561125956,4.16146346413405,9.63525848462867));
#60230=CARTESIAN_POINT('Ctrl Pts',(23.8489202354448,-0.954136277735047,
10.4520623894254));
#60231=CARTESIAN_POINT('Ctrl Pts',(23.967984358294,-5.83728649460537,8.72250368924138));
#60232=CARTESIAN_POINT('Ctrl Pts',(24.0857400567879,-9.26030522340976,4.91030133265418));
#60233=CARTESIAN_POINT('Ctrl Pts',(24.1638077143321,-10.0688240585487,1.61817458867476));
#60234=CARTESIAN_POINT('Ctrl Pts',(24.2021873309266,-10.0693361365586,-5.80152907240453E-5));
#60235=CARTESIAN_POINT('Ctrl Pts',(22.9978126690739,-10.0679008419791,-0.000190872912600032));
#60236=CARTESIAN_POINT('Ctrl Pts',(23.0121264311565,-10.0683142775377,-0.603962435218835));
#60237=CARTESIAN_POINT('Ctrl Pts',(23.0660418718992,-9.86702508181923,-2.8779075948163));
#60238=CARTESIAN_POINT('Ctrl Pts',(23.159558991302,-8.17588470309968,-6.5780727409721));
#60239=CARTESIAN_POINT('Ctrl Pts',(23.2783640272822,-4.04409018769059,-9.68305046035207));
#60240=CARTESIAN_POINT('Ctrl Pts',(23.3971690632624,1.06874327896542,-10.4390574032125));
#60241=CARTESIAN_POINT('Ctrl Pts',(23.5159740992426,5.92231477645477,-8.66269700223236));
#60242=CARTESIAN_POINT('Ctrl Pts',(23.6347791352229,9.33921666283309,-4.78488910932746));
#60243=CARTESIAN_POINT('Ctrl Pts',(23.7535841712031,10.4905569778446,0.253665051782705));
#60244=CARTESIAN_POINT('Ctrl Pts',(23.8723892071833,9.09703688225833,5.23068366724002));
#60245=CARTESIAN_POINT('Ctrl Pts',(23.9911942431636,5.49670459697617,8.93881257424503));
#60246=CARTESIAN_POINT('Ctrl Pts',(24.1099992791438,0.562949696752003,10.4785122657192));
#60247=CARTESIAN_POINT('Ctrl Pts',(24.228804315124,-4.50736881963169,9.47627342301349));
#60248=CARTESIAN_POINT('Ctrl Pts',(24.3476093511042,-8.48426355601317,6.17522498181294));
#60249=CARTESIAN_POINT('Ctrl Pts',(24.4372788024209,-9.93244884747991,2.55307198566314));
#60250=CARTESIAN_POINT('Ctrl Pts',(24.4873465750774,-10.0687583625544,0.441674558944737));
#60251=CARTESIAN_POINT('Ctrl Pts',(24.4978126690739,-10.0683262561367,0.000255752892878991));
#60252=CARTESIAN_POINT('Origin',(-2.04781266907391,0.,0.));
#60253=CARTESIAN_POINT('',(21.2021873309261,-10.0685057068065,-0.000260789586672069));
#60254=CARTESIAN_POINT('',(21.4978126690739,-10.0693516963442,2.25242750905193E-5));
#60255=CARTESIAN_POINT('',(-2.04781266907391,-10.0685,8.88799240754737E-13));
#60256=CARTESIAN_POINT('Ctrl Pts',(21.2021873309266,-10.0685057068056,-0.000260789586671792));
#60257=CARTESIAN_POINT('Ctrl Pts',(21.2112947315386,-10.0689002652111,-0.384355477911598));
#60258=CARTESIAN_POINT('Ctrl Pts',(21.2600901731003,-9.95339909903588,-2.44201409800743));
#60259=CARTESIAN_POINT('Ctrl Pts',(21.3485736556117,-8.58346085548246,-6.03988277794626));
#60260=CARTESIAN_POINT('Ctrl Pts',(21.467637778461,-4.64893203446674,-9.40975106832484));
#60261=CARTESIAN_POINT('Ctrl Pts',(21.5867019013101,0.41818347084202,-10.4871877457041));
#60262=CARTESIAN_POINT('Ctrl Pts',(21.7057660241593,5.38341987205639,-9.00970447407017));
#60263=CARTESIAN_POINT('Ctrl Pts',(21.8248301470085,9.03713147190878,-5.33725013357698));
#60264=CARTESIAN_POINT('Ctrl Pts',(21.9438942698577,10.4891901559074,-0.364519001077752));
#60265=CARTESIAN_POINT('Ctrl Pts',(22.0629583927069,9.38584105774835,4.69701733737661));
#60266=CARTESIAN_POINT('Ctrl Pts',(22.1820225155561,5.99588537466088,8.6142523066636));
#60267=CARTESIAN_POINT('Ctrl Pts',(22.3010866384053,1.14519421823428,10.4328574432633));
#60268=CARTESIAN_POINT('Ctrl Pts',(22.4201507612545,-3.98449256834685,9.70977874113103));
#60269=CARTESIAN_POINT('Ctrl Pts',(22.5392148841037,-8.14346539457826,6.6211747897362));
#60270=CARTESIAN_POINT('Ctrl Pts',(22.6332270739944,-9.86085963586431,2.90876599529836));
#60271=CARTESIAN_POINT('Ctrl Pts',(22.6875512229354,-10.068276484189,0.61755879703295));
#60272=CARTESIAN_POINT('Ctrl Pts',(22.7021873309266,-10.0678699062581,0.000184994001410643));
#60273=CARTESIAN_POINT('Ctrl Pts',(21.4978126690739,-10.0693516963442,2.25242750904976E-5));
#60274=CARTESIAN_POINT('Ctrl Pts',(21.5369062872356,-10.0691372904009,-1.64830792016672));
#60275=CARTESIAN_POINT('Ctrl Pts',(21.6156015840574,-9.23770971868321,-4.96659892897904));
#60276=CARTESIAN_POINT('Ctrl Pts',(21.7338985595392,-5.76726644021558,-8.76668520430974));
#60277=CARTESIAN_POINT('Ctrl Pts',(21.8527035955195,-0.882861258940293,
-10.4564184911165));
#60278=CARTESIAN_POINT('Ctrl Pts',(21.9715086314997,4.21571354847328,-9.6095728802647));
#60279=CARTESIAN_POINT('Ctrl Pts',(22.0903136674799,8.29161601021562,-6.43158111221775));
#60280=CARTESIAN_POINT('Ctrl Pts',(22.2091187034601,10.3560899683198,-1.69337893927062));
#60281=CARTESIAN_POINT('Ctrl Pts',(22.3279237394404,9.90832330615713,3.45561295931176));
#60282=CARTESIAN_POINT('Ctrl Pts',(22.4467287754206,7.05693786850942,7.7663221401058));
#60283=CARTESIAN_POINT('Ctrl Pts',(22.5655338114008,2.4936393418288,10.19303166368));
#60284=CARTESIAN_POINT('Ctrl Pts',(22.6843388473811,-2.67458073980179,10.1470562002081));
#60285=CARTESIAN_POINT('Ctrl Pts',(22.8031438833613,-7.19398544832653,7.63954874538845));
#60286=CARTESIAN_POINT('Ctrl Pts',(22.9076351572589,-9.63398706426305,3.80418348672512));
#60287=CARTESIAN_POINT('Ctrl Pts',(22.9725247524964,-10.0671704313537,1.0664836191823));
#60288=CARTESIAN_POINT('Ctrl Pts',(22.9978126690739,-10.0679008419791,-0.000190872912600032));
#60289=CARTESIAN_POINT('Origin',(-2.04781266907391,0.,0.));
#60290=CARTESIAN_POINT('',(19.7021873309261,-10.0688072251698,0.000237565543711042));
#60291=CARTESIAN_POINT('',(19.9978126690739,-10.0678175549596,0.000161722309567902));
#60292=CARTESIAN_POINT('',(-2.04781266907391,-10.0685,8.88799240754737E-13));
#60293=CARTESIAN_POINT('Ctrl Pts',(19.7021873309266,-10.0688072251689,0.000237565543710905));
#60294=CARTESIAN_POINT('Ctrl Pts',(19.7350382401418,-10.0674202771142,-1.38509415302326));
#60295=CARTESIAN_POINT('Ctrl Pts',(19.8075771903068,-9.43093755098151,-4.44531612426048));
#60296=CARTESIAN_POINT('Ctrl Pts',(19.9198041814215,-6.42871960487108,-8.29623700667221));
#60297=CARTESIAN_POINT('Ctrl Pts',(20.0388683042706,-1.677415655117,-10.360611031638));
#60298=CARTESIAN_POINT('Ctrl Pts',(20.1579324271198,3.48254529820804,-9.90090210409437));
#60299=CARTESIAN_POINT('Ctrl Pts',(20.276996549969,7.79407818182693,-7.02910588371671));
#60300=CARTESIAN_POINT('Ctrl Pts',(20.3960606728182,10.2067944986236,-2.44485792875554));
#60301=CARTESIAN_POINT('Ctrl Pts',(20.5151247956674,10.1329011053296,2.73501360481841));
#60302=CARTESIAN_POINT('Ctrl Pts',(20.6341889185166,7.5904001307525,7.24857296879903));
#60303=CARTESIAN_POINT('Ctrl Pts',(20.7532530413658,3.19870324347748,9.99621337252753));
#60304=CARTESIAN_POINT('Ctrl Pts',(20.872317164215,-1.97227126577789,10.3085464680098));
#60305=CARTESIAN_POINT('Ctrl Pts',(20.9913812870642,-6.66275516840085,8.10948073521845));
#60306=CARTESIAN_POINT('Ctrl Pts',(21.1013380093014,-9.49541747792732,4.25409009765303));
#60307=CARTESIAN_POINT('Ctrl Pts',(21.1716066905889,-10.0671808667985,1.28944436556644));
#60308=CARTESIAN_POINT('Ctrl Pts',(21.2021873309266,-10.0685057068056,-0.000260789586671792));
#60309=CARTESIAN_POINT('Ctrl Pts',(19.9978126690739,-10.0678175549596,0.000161722309567555));
#60310=CARTESIAN_POINT('Ctrl Pts',(20.0220844646546,-10.0672300748146,-1.02367583636044));
#60311=CARTESIAN_POINT('Ctrl Pts',(20.0859579388954,-9.65852627294022,-3.71845755382397));
#60312=CARTESIAN_POINT('Ctrl Pts',(20.1894330917963,-7.29094536875751,-7.54706878819144));
#60313=CARTESIAN_POINT('Ctrl Pts',(20.3082381277765,-2.80392646587668,-10.1120783243533));
#60314=CARTESIAN_POINT('Ctrl Pts',(20.4270431637567,2.36328524967433,-10.2240410060099));
#60315=CARTESIAN_POINT('Ctrl Pts',(20.545848199737,6.95719746515613,-7.85579627375385));
#60316=CARTESIAN_POINT('Ctrl Pts',(20.6646532357172,9.86339219955671,-3.58184672782404));
#60317=CARTESIAN_POINT('Ctrl Pts',(20.7834582716974,10.3768678079984,1.56100805866827));
#60318=CARTESIAN_POINT('Ctrl Pts',(20.9022633076776,8.37306238680994,6.32518441869393));
#60319=CARTESIAN_POINT('Ctrl Pts',(21.0210683436579,4.33807072559066,9.55496070340811));
#60320=CARTESIAN_POINT('Ctrl Pts',(21.1398733796381,-0.74927539795548,10.4668389708602));
#60321=CARTESIAN_POINT('Ctrl Pts',(21.2586784156183,-5.65485793154934,8.83961047998685));
#60322=CARTESIAN_POINT('Ctrl Pts',(21.3774834515986,-9.18865209318669,5.06801779537876));
#60323=CARTESIAN_POINT('Ctrl Pts',(21.4571948694171,-10.0640700671677,1.71261667486192));
#60324=CARTESIAN_POINT('Ctrl Pts',(21.4973046085755,-10.0693544827629,0.0214442198474628));
#60325=CARTESIAN_POINT('Ctrl Pts',(21.4978126690739,-10.0693516963442,2.25242750904976E-5));
#60326=CARTESIAN_POINT('Origin',(-2.04781266907391,0.,0.));
#60327=CARTESIAN_POINT('',(18.2021873309261,-10.0677138734479,-0.00011191168250948));
#60328=CARTESIAN_POINT('',(18.4978126690739,-10.0684578404949,-0.000258528687929749));
#60329=CARTESIAN_POINT('',(-2.04781266907391,-10.0685,8.88799240754737E-13));
#60330=CARTESIAN_POINT('Ctrl Pts',(18.2021873309266,-10.067713873447,-0.000111911682509278));
#60331=CARTESIAN_POINT('Ctrl Pts',(18.2190937077954,-10.067992386815,-0.713280830752772));
#60332=CARTESIAN_POINT('Ctrl Pts',(18.2756881256138,-9.81788713094357,-3.10043482706846));
#60333=CARTESIAN_POINT('Ctrl Pts',(18.3719705843819,-7.95128147286543,-6.85077420210285));
#60334=CARTESIAN_POINT('Ctrl Pts',(18.4910347072312,-3.70589808496221,-9.81948591387579));
#60335=CARTESIAN_POINT('Ctrl Pts',(18.6100988300803,1.44232724454336,-10.3959451878403));
#60336=CARTESIAN_POINT('Ctrl Pts',(18.7291629529295,6.23916851004201,-8.43971329680288));
#60337=CARTESIAN_POINT('Ctrl Pts',(18.8482270757787,9.51600493934509,-4.427373287096));
#60338=CARTESIAN_POINT('Ctrl Pts',(18.9672911986279,10.4745238707661,0.663576604231755));
#60339=CARTESIAN_POINT('Ctrl Pts',(19.0863553214771,8.88120806414699,5.59286398460229));
#60340=CARTESIAN_POINT('Ctrl Pts',(19.2054194443263,5.12422586720129,9.15960116439776));
#60341=CARTESIAN_POINT('Ctrl Pts',(19.3244835671755,0.118864485213787,10.4948489966786));
#60342=CARTESIAN_POINT('Ctrl Pts',(19.4435476900247,-4.91545501708828,9.27331042313978));
#60343=CARTESIAN_POINT('Ctrl Pts',(19.5626118128739,-8.75225671136026,5.79258031341651));
#60344=CARTESIAN_POINT('Ctrl Pts',(19.6488250265079,-9.98650595639443,2.25037552552701));
#60345=CARTESIAN_POINT('Ctrl Pts',(19.6953501991921,-10.0690958852635,0.28856125831586));
#60346=CARTESIAN_POINT('Ctrl Pts',(19.7021873309266,-10.0688072251689,0.000237565543710905));
#60347=CARTESIAN_POINT('Ctrl Pts',(18.4978126690739,-10.0684578404949,-0.000258528687930581));
#60348=CARTESIAN_POINT('Ctrl Pts',(18.5072626420736,-10.0688617098177,-0.39880635749866));
#60349=CARTESIAN_POINT('Ctrl Pts',(18.5563142937334,-9.94835311716881,-2.46729222591912));
#60350=CARTESIAN_POINT('Ctrl Pts',(18.6449676240533,-8.56242091716224,-6.06638934632804));
#60351=CARTESIAN_POINT('Ctrl Pts',(18.7637726600336,-4.62800017217989,-9.41794808173218));
#60352=CARTESIAN_POINT('Ctrl Pts',(18.8825776960137,0.42910780888478,-10.4848461196268));
#60353=CARTESIAN_POINT('Ctrl Pts',(19.001382731994,5.38212031846822,-9.00826912017127));
#60354=CARTESIAN_POINT('Ctrl Pts',(19.1201877679742,9.02950673474984,-5.34641373174648));
#60355=CARTESIAN_POINT('Ctrl Pts',(19.2389928039545,10.486462817826,-0.387594161788445));
#60356=CARTESIAN_POINT('Ctrl Pts',(19.3577978399347,9.39955167548687,4.66525025735512));
#60357=CARTESIAN_POINT('Ctrl Pts',(19.4766028759149,6.03244254300923,8.58637109780332));
#60358=CARTESIAN_POINT('Ctrl Pts',(19.5954079118952,1.20194836440568,10.4245600287591));
#60359=CARTESIAN_POINT('Ctrl Pts',(19.7142129478754,-3.92012144880135,9.73389847340455));
#60360=CARTESIAN_POINT('Ctrl Pts',(19.8330179838556,-8.09122536945768,6.68193113437607));
#60361=CARTESIAN_POINT('Ctrl Pts',(19.9275512242551,-9.84836097238885,2.96369447334041));
#60362=CARTESIAN_POINT('Ctrl Pts',(19.9824827859945,-10.0681886029895,0.646809804626538));
#60363=CARTESIAN_POINT('Ctrl Pts',(19.9978126690739,-10.0678175549596,0.000161722309567555));
#60364=CARTESIAN_POINT('Origin',(-2.04781266907391,0.,0.));
#60365=CARTESIAN_POINT('',(16.7021873309261,-10.0693485471037,-4.28479981268501E-5));
#60366=CARTESIAN_POINT('',(16.9978126690739,-10.068983884147,0.000203272603223198));
#60367=CARTESIAN_POINT('',(-2.04781266907391,-10.0685,8.88799240754737E-13));
#60368=CARTESIAN_POINT('Ctrl Pts',(16.7021873309266,-10.0693485471029,-4.28479981270415E-5));
#60369=CARTESIAN_POINT('Ctrl Pts',(16.7031491754488,-10.0693582384133,-0.0405977757395343));
#60370=CARTESIAN_POINT('Ctrl Pts',(16.7437990609208,-10.0592200321944,-1.75454265156612));
#60371=CARTESIAN_POINT('Ctrl Pts',(16.8241369873425,-9.15569694661239,-5.13119846144389));
#60372=CARTESIAN_POINT('Ctrl Pts',(16.9432011101916,-5.58610025115397,-8.88546387157073));
#60373=CARTESIAN_POINT('Ctrl Pts',(17.0622652330409,-0.655601156031094,
-10.4750260788765));
#60374=CARTESIAN_POINT('Ctrl Pts',(17.18132935589,4.43461744757741,-9.51263119870489));
#60375=CARTESIAN_POINT('Ctrl Pts',(17.3003934787392,8.4444613255881,-6.23274074140566));
#60376=CARTESIAN_POINT('Ctrl Pts',(17.4194576015884,10.3970403559991,-1.43441140007221));
#60377=CARTESIAN_POINT('Ctrl Pts',(17.5385217244376,9.81666141327586,3.71337352363487));
#60378=CARTESIAN_POINT('Ctrl Pts',(17.6575858472868,6.84471814600233,7.9564953170801));
#60379=CARTESIAN_POINT('Ctrl Pts',(17.776649970136,2.20524423460953,10.2612319969219));
#60380=CARTESIAN_POINT('Ctrl Pts',(17.8957140929852,-2.97147785275479,10.0660967410173));
#60381=CARTESIAN_POINT('Ctrl Pts',(18.0147782158344,-7.42427964536093,7.41862898225881));
#60382=CARTESIAN_POINT('Ctrl Pts',(18.1169359618149,-9.69291358885776,3.59636936095307));
#60383=CARTESIAN_POINT('Ctrl Pts',(18.1794056668456,-10.0673385713915,0.96089675820891));
#60384=CARTESIAN_POINT('Ctrl Pts',(18.2021873309266,-10.067713873447,-0.000111911682509278));
#60385=CARTESIAN_POINT('Ctrl Pts',(16.9978126690739,-10.068983884147,0.000203272603222782));
#60386=CARTESIAN_POINT('Ctrl Pts',(17.0320424981527,-10.0676740526606,-1.44320493355459));
#60387=CARTESIAN_POINT('Ctrl Pts',(17.1058740058916,-9.39095340106168,-4.55773078782869));
#60388=CARTESIAN_POINT('Ctrl Pts',(17.2193071922906,-6.29198527163358,-8.39803864038776));
#60389=CARTESIAN_POINT('Ctrl Pts',(17.3381122282708,-1.51991303483393,-10.3829666295545));
#60390=CARTESIAN_POINT('Ctrl Pts',(17.4569172642511,3.62086855820574,-9.84913410143739));
#60391=CARTESIAN_POINT('Ctrl Pts',(17.5757223002313,7.88327876779868,-6.92604125984493));
#60392=CARTESIAN_POINT('Ctrl Pts',(17.6945273362115,10.2333173002494,-2.32278899091503));
#60393=CARTESIAN_POINT('Ctrl Pts',(17.8133323721917,10.1008981213041,2.8439389597766));
#60394=CARTESIAN_POINT('Ctrl Pts',(17.932137408172,7.51814424662471,7.32076763398781));
#60395=CARTESIAN_POINT('Ctrl Pts',(18.0509424441522,3.11159515355942,10.0216818580638));
#60396=CARTESIAN_POINT('Ctrl Pts',(18.1697474801324,-2.0497828143526,10.2914781289125));
#60397=CARTESIAN_POINT('Ctrl Pts',(18.2885525161126,-6.71391252885095,8.06470769580882));
#60398=CARTESIAN_POINT('Ctrl Pts',(18.3979075790931,-9.5078985277881,4.21428934597389));
#60399=CARTESIAN_POINT('Ctrl Pts',(18.4676609634136,-10.0671692284589,1.27137439832779));
#60400=CARTESIAN_POINT('Ctrl Pts',(18.4978126690739,-10.0684578404949,-0.000258528687930581));
#60401=CARTESIAN_POINT('Origin',(-2.04781266907391,0.,0.));
#60402=CARTESIAN_POINT('',(15.2021873309261,-10.0678410649975,0.000175016129901548));
#60403=CARTESIAN_POINT('',(15.4978126690739,-10.0676474335291,-1.53024526838852E-5));
#60404=CARTESIAN_POINT('',(-2.04781266907391,-10.0685,8.88799240754737E-13));
#60405=CARTESIAN_POINT('Ctrl Pts',(15.2021873309266,-10.0678410649967,0.000175016129901062));
#60406=CARTESIAN_POINT('Ctrl Pts',(15.2268926840521,-10.0671942423325,-1.04194376071667));
#60407=CARTESIAN_POINT('Ctrl Pts',(15.2912860781273,-9.64759913025132,-3.75868851590533));
#60408=CARTESIAN_POINT('Ctrl Pts',(15.3953675131521,-7.24279157083963,-7.5959169617832));
#60409=CARTESIAN_POINT('Ctrl Pts',(15.5144316360014,-2.72729766624086,-10.134980595376));
#60410=CARTESIAN_POINT('Ctrl Pts',(15.6334957588506,2.45262862798792,-10.2049300361201));
#60411=CARTESIAN_POINT('Ctrl Pts',(15.7525598816997,7.03503822268641,-7.78872399268793));
#60412=CARTESIAN_POINT('Ctrl Pts',(15.8716240045489,9.90355082869269,-3.47500578595657));
#60413=CARTESIAN_POINT('Ctrl Pts',(15.9906881273981,10.3593308516804,1.68530369202511));
#60414=CARTESIAN_POINT('Ctrl Pts',(16.1097522502473,8.29133980341716,6.43503445936399));
#60415=CARTESIAN_POINT('Ctrl Pts',(16.2288163730965,4.20338782935896,9.61704294390578));
#60416=CARTESIAN_POINT('Ctrl Pts',(16.3478804959457,-0.908606021232575,
10.4561187506221));
#60417=CARTESIAN_POINT('Ctrl Pts',(16.4669446187949,-5.79924256367529,8.74784372954778));
#60418=CARTESIAN_POINT('Ctrl Pts',(16.5850468971219,-9.24895530858255,4.93940945473011));
#60419=CARTESIAN_POINT('Ctrl Pts',(16.6634611344991,-10.0689583514083,1.63279703573205));
#60420=CARTESIAN_POINT('Ctrl Pts',(16.7021873309266,-10.0693485471029,-4.28479981270415E-5));
#60421=CARTESIAN_POINT('Ctrl Pts',(15.4978126690739,-10.0676474335291,-1.53024526847872E-5));
#60422=CARTESIAN_POINT('Ctrl Pts',(15.5172206755717,-10.0676909481092,-0.818727170628262));
#60423=CARTESIAN_POINT('Ctrl Pts',(15.5762303607296,-9.76753611475359,-3.30797412144366));
#60424=CARTESIAN_POINT('Ctrl Pts',(15.6748417245476,-7.73832233327883,-7.08763000799124));
#60425=CARTESIAN_POINT('Ctrl Pts',(15.7936467605279,-3.41635808961021,-9.92192668121746));
#60426=CARTESIAN_POINT('Ctrl Pts',(15.9124517965081,1.73436619692707,-10.349304593008));
#60427=CARTESIAN_POINT('Ctrl Pts',(16.0312568324883,6.46435783014953,-8.26608792039404));
#60428=CARTESIAN_POINT('Ctrl Pts',(16.1500618684685,9.62618789133837,-4.17763549685113));
#60429=CARTESIAN_POINT('Ctrl Pts',(16.2688669044488,10.4528412291769,0.924252076827058));
#60430=CARTESIAN_POINT('Ctrl Pts',(16.387671940429,8.74378346239289,5.80192919869627));
#60431=CARTESIAN_POINT('Ctrl Pts',(16.5064769764092,4.91360777791608,9.27214054405468));
#60432=CARTESIAN_POINT('Ctrl Pts',(16.6252820123894,-0.10853949907314,10.493062033603));
#60433=CARTESIAN_POINT('Ctrl Pts',(16.7440870483697,-5.10435663222344,9.16851542153781));
#60434=CARTESIAN_POINT('Ctrl Pts',(16.8628920843499,-8.86192920482737,5.61981693941426));
#60435=CARTESIAN_POINT('Ctrl Pts',(16.9474672912513,-10.0064894810931,2.12306056737073));
#60436=CARTESIAN_POINT('Ctrl Pts',(16.9924408194926,-10.0691894422205,0.226724174883204));
#60437=CARTESIAN_POINT('Ctrl Pts',(16.9978126690739,-10.068983884147,0.000203272603222782));
#60438=CARTESIAN_POINT('Origin',(-2.04781266907391,0.,0.));
#60439=CARTESIAN_POINT('',(13.7021873309261,-10.0685519820608,-0.000259412661711476));
#60440=CARTESIAN_POINT('',(13.9978126690739,-10.0690725182231,-0.000180988700121398));
#60441=CARTESIAN_POINT('',(-2.04781266907391,-10.0685,8.88799240754737E-13));
#60442=CARTESIAN_POINT('Ctrl Pts',(13.7021873309266,-10.0685519820599,-0.000259412661711006));
#60443=CARTESIAN_POINT('Ctrl Pts',(13.7109481517056,-10.0689330049364,-0.369732586853416));
#60444=CARTESIAN_POINT('Ctrl Pts',(13.7593970134343,-9.95863578298735,-2.41275720947365));
#60445=CARTESIAN_POINT('Ctrl Pts',(13.8475339161127,-8.60968456928456,-6.00244249004976));
#60446=CARTESIAN_POINT('Ctrl Pts',(13.9665980389618,-4.68986963828456,-9.38941462524836));
#60447=CARTESIAN_POINT('Ctrl Pts',(14.0856621618111,0.372505318117175,-10.4889095723486));
#60448=CARTESIAN_POINT('Ctrl Pts',(14.2047262846602,5.34412941819326,-9.03306509389438));
#60449=CARTESIAN_POINT('Ctrl Pts',(14.3237904075095,9.0138007744326,-5.37655836272329));
#60450=CARTESIAN_POINT('Ctrl Pts',(14.4428545303586,10.4875031089042,-0.410198451553393));
#60451=CARTESIAN_POINT('Ctrl Pts',(14.5619186532078,9.40620866463942,4.65609522950223));
#60452=CARTESIAN_POINT('Ctrl Pts',(14.680982776057,6.03334561832389,8.58805710733127));
#60453=CARTESIAN_POINT('Ctrl Pts',(14.8000468989062,1.19062092241009,10.4277709050425));
#60454=CARTESIAN_POINT('Ctrl Pts',(14.9191110217554,-3.94216639278166,9.72704006162999));
#60455=CARTESIAN_POINT('Ctrl Pts',(15.0381751446046,-8.1145513767218,6.65657871458557));
#60456=CARTESIAN_POINT('Ctrl Pts',(15.1325339143283,-9.85448854023772,2.93802654270935));
#60457=CARTESIAN_POINT('Ctrl Pts',(15.1872046431023,-10.0682333339112,0.632173281041699));
#60458=CARTESIAN_POINT('Ctrl Pts',(15.2021873309266,-10.0678410649967,0.000175016129901062));
#60459=CARTESIAN_POINT('Ctrl Pts',(13.9978126690739,-10.0690725182231,-0.000180988700121433));
#60460=CARTESIAN_POINT('Ctrl Pts',(14.0023988529907,-10.0692339538579,-0.193566905138866));
#60461=CARTESIAN_POINT('Ctrl Pts',(14.0465867155677,-10.0166511244356,-2.05675165468336));
#60462=CARTESIAN_POINT('Ctrl Pts',(14.1303762568047,-8.91698065775955,-5.53205094092975));
#60463=CARTESIAN_POINT('Ctrl Pts',(14.2491812927849,-5.19462682919267,-9.11767425220551));
#60464=CARTESIAN_POINT('Ctrl Pts',(14.3679863287651,-0.212130169948613,
-10.4914790403879));
#60465=CARTESIAN_POINT('Ctrl Pts',(14.4867913647454,4.82182626140632,-9.32019973867041));
#60466=CARTESIAN_POINT('Ctrl Pts',(14.6055964007256,8.68607599507601,-5.88797210180758));
#60467=CARTESIAN_POINT('Ctrl Pts',(14.7244014367058,10.4432068245734,-1.02740589986761));
#60468=CARTESIAN_POINT('Ctrl Pts',(14.843206472686,9.66696371942952,4.08239440906108));
#60469=CARTESIAN_POINT('Ctrl Pts',(14.9620115086663,6.54565225307114,8.20186370563207));
#60470=CARTESIAN_POINT('Ctrl Pts',(15.0808165446465,1.83645834009328,10.3316771353446));
#60471=CARTESIAN_POINT('Ctrl Pts',(15.1996215806267,-3.31823433289184,9.95517215199806));
#60472=CARTESIAN_POINT('Ctrl Pts',(15.318426616607,-7.6679703954037,7.16368352728626));
#60473=CARTESIAN_POINT('Ctrl Pts',(15.4178236460893,-9.75086494544946,3.37429334153181));
#60474=CARTESIAN_POINT('Ctrl Pts',(15.4776189969116,-10.0676021574126,0.851839269170285));
#60475=CARTESIAN_POINT('Ctrl Pts',(15.4978126690739,-10.0676474335291,-1.53024526847872E-5));
#60476=CARTESIAN_POINT('Origin',(-2.04781266907391,0.,0.));
#60477=CARTESIAN_POINT('',(12.2021873309261,-10.0687619984752,0.000243267090029437));
#60478=CARTESIAN_POINT('',(12.4978126690739,-10.068355685636,0.000256951768887181));
#60479=CARTESIAN_POINT('',(-2.04781266907391,-10.0685,8.88799240754737E-13));
#60480=CARTESIAN_POINT('Ctrl Pts',(12.2021873309266,-10.0687619984744,0.000243267090029586));
#60481=CARTESIAN_POINT('Ctrl Pts',(12.2346916603088,-10.0673727699987,-1.37049085012941));
#60482=CARTESIAN_POINT('Ctrl Pts',(12.3068840306407,-9.44098893284163,-4.41613269318898));
#60483=CARTESIAN_POINT('Ctrl Pts',(12.4187644419224,-6.4647907115389,-8.26815972783132));
#60484=CARTESIAN_POINT('Ctrl Pts',(12.5378285647716,-1.72252266142237,-10.3532072281887));
#60485=CARTESIAN_POINT('Ctrl Pts',(12.6568926876207,3.43939149564005,-9.91597551270928));
#60486=CARTESIAN_POINT('Ctrl Pts',(12.7759568104699,7.76339084105272,-7.06298427564369));
#60487=CARTESIAN_POINT('Ctrl Pts',(12.8950209333191,10.1960497611052,-2.48928774913569));
#60488=CARTESIAN_POINT('Ctrl Pts',(13.0140850561683,10.1447166360597,2.69085648130572));
#60489=CARTESIAN_POINT('Ctrl Pts',(13.1331491790175,7.62189739490336,7.21544623225042));
#60490=CARTESIAN_POINT('Ctrl Pts',(13.2522133018667,3.242208783639,9.98218745727736));
#60491=CARTESIAN_POINT('Ctrl Pts',(13.3712774247159,-1.92735639902351,10.3170384093535));
#60492=CARTESIAN_POINT('Ctrl Pts',(13.4903415475651,-6.62737326881817,8.13842170108466));
#60493=CARTESIAN_POINT('Ctrl Pts',(13.6006448496353,-9.48578114781274,4.28329148486634));
#60494=CARTESIAN_POINT('Ctrl Pts',(13.6712601107558,-10.0672069050758,1.30404511470363));
#60495=CARTESIAN_POINT('Ctrl Pts',(13.7021873309266,-10.0685519820599,-0.000259412661711006));
#60496=CARTESIAN_POINT('Ctrl Pts',(12.4978126690739,-10.068355685636,0.000256951768887251));
#60497=CARTESIAN_POINT('Ctrl Pts',(12.5271787090698,-10.0671313314383,-1.23827706190051));
#60498=CARTESIAN_POINT('Ctrl Pts',(12.5961464277258,-9.52924259170233,-4.14807463219822));
#60499=CARTESIAN_POINT('Ctrl Pts',(12.7047158250419,-6.79320660134877,-7.99802949077405));
#60500=CARTESIAN_POINT('Ctrl Pts',(12.8235208610222,-2.15128867552026,-10.270739442634));
#60501=CARTESIAN_POINT('Ctrl Pts',(12.9423258970024,3.01250138671254,-10.0519136018449));
#60502=CARTESIAN_POINT('Ctrl Pts',(13.0611309329826,7.44550131720053,-7.39463601534687));
#60503=CARTESIAN_POINT('Ctrl Pts',(13.1799359689628,10.0723281742079,-2.94352455654064));
#60504=CARTESIAN_POINT('Ctrl Pts',(13.2987410049431,10.2557509996443,2.2216442328137));
#60505=CARTESIAN_POINT('Ctrl Pts',(13.4175460409233,7.95127401622754,6.84787362491195));
#60506=CARTESIAN_POINT('Ctrl Pts',(13.5363510769035,3.71793067228796,9.81290594981732));
#60507=CARTESIAN_POINT('Ctrl Pts',(13.6551561128838,-1.41732994803981,10.3974663972667));
#60508=CARTESIAN_POINT('Ctrl Pts',(13.773961148864,-6.20876641478464,8.4597488893313));
#60509=CARTESIAN_POINT('Ctrl Pts',(13.8881800009274,-9.36722388326039,4.62383802070818));
#60510=CARTESIAN_POINT('Ctrl Pts',(13.9627971743306,-10.0678399578368,1.47631966265573));
#60511=CARTESIAN_POINT('Ctrl Pts',(13.9978126690739,-10.0690725182231,-0.000180988700121433));
#60512=CARTESIAN_POINT('Origin',(-2.04781266907391,0.,0.));
#60513=CARTESIAN_POINT('',(10.7021873309261,-10.0677324747908,-0.000124116338529288));
#60514=CARTESIAN_POINT('',(10.9978126690739,-10.0678806802972,-0.000184627883193511));
#60515=CARTESIAN_POINT('',(-2.04781266907391,-10.0685,8.88799240754737E-13));
#60516=CARTESIAN_POINT('Ctrl Pts',(10.7021873309266,-10.0677324747899,-0.000124116338529254));
#60517=CARTESIAN_POINT('Ctrl Pts',(10.7187471279623,-10.0680357258477,-0.698669416730243));
#60518=CARTESIAN_POINT('Ctrl Pts',(10.7749949659477,-9.82463694103478,-3.07117511324269));
#60519=CARTESIAN_POINT('Ctrl Pts',(10.8709308448829,-7.98104280653367,-6.81607951458966));
#60520=CARTESIAN_POINT('Ctrl Pts',(10.9899949677321,-3.74862912490046,-9.80325272105535));
#60521=CARTESIAN_POINT('Ctrl Pts',(11.1090590905813,1.39703676169904,-10.4021282685512));
#60522=CARTESIAN_POINT('Ctrl Pts',(11.2281232134305,6.20235238676807,-8.46680631048589));
#60523=CARTESIAN_POINT('Ctrl Pts',(11.3471873362796,9.49663242937081,-4.4687757529724));
#60524=CARTESIAN_POINT('Ctrl Pts',(11.4662514591288,10.4773145627358,0.617951278351491));
#60525=CARTESIAN_POINT('Ctrl Pts',(11.585315581978,8.90548208136188,5.55413117665345));
#60526=CARTESIAN_POINT('Ctrl Pts',(11.7043797048272,5.1640695012078,9.13719707654523));
#60527=CARTESIAN_POINT('Ctrl Pts',(11.8234438276764,0.164570911090679,10.4942317796089));
#60528=CARTESIAN_POINT('Ctrl Pts',(11.9425079505256,-4.87502093509933,9.29463044511586));
#60529=CARTESIAN_POINT('Ctrl Pts',(12.0615720733748,-8.72694564487861,5.83064352711308));
#60530=CARTESIAN_POINT('Ctrl Pts',(12.1481318668418,-9.98163401640052,2.27962975137199));
#60531=CARTESIAN_POINT('Ctrl Pts',(12.1950036193591,-10.0690690288565,0.303186251026718));
#60532=CARTESIAN_POINT('Ctrl Pts',(12.2021873309266,-10.0687619984744,0.000243267090029586));
#60533=CARTESIAN_POINT('Ctrl Pts',(10.9978126690739,-10.0678806802972,-0.000184627883194205));
#60534=CARTESIAN_POINT('Ctrl Pts',(11.0123568864888,-10.0682859280004,-0.613680591180964));
#60535=CARTESIAN_POINT('Ctrl Pts',(11.0665027825639,-9.86284322026599,-2.89736401120441));
#60536=CARTESIAN_POINT('Ctrl Pts',(11.160250357299,-8.15680043132904,-6.60172238036183));
#60537=CARTESIAN_POINT('Ctrl Pts',(11.2790553932792,-4.01603127915127,-9.69472147247038));
#60538=CARTESIAN_POINT('Ctrl Pts',(11.3978604292594,1.09897013081975,-10.4359185659656));
#60539=CARTESIAN_POINT('Ctrl Pts',(11.5166654652397,5.94737696585456,-8.64550975304073));
#60540=CARTESIAN_POINT('Ctrl Pts',(11.6354705012199,9.35303445790701,-4.75782283120169));
#60541=CARTESIAN_POINT('Ctrl Pts',(11.7542755372001,10.4897783773862,0.284044463455958));
#60542=CARTESIAN_POINT('Ctrl Pts',(11.8730805731804,9.08185076370161,5.25700659784181));
#60543=CARTESIAN_POINT('Ctrl Pts',(11.9918856091606,5.47079489740727,8.95469345396048));
#60544=CARTESIAN_POINT('Ctrl Pts',(12.1106906451408,0.532601741995187,10.4800986182537));
#60545=CARTESIAN_POINT('Ctrl Pts',(12.229495681121,-4.53479304595954,9.46318042173016));
#60546=CARTESIAN_POINT('Ctrl Pts',(12.3483007171013,-8.50211132536573,6.15062880321902));
#60547=CARTESIAN_POINT('Ctrl Pts',(12.4377397130855,-9.93610591059234,2.53361694437834));
#60548=CARTESIAN_POINT('Ctrl Pts',(12.4875770304097,-10.068782438687,0.431952428547841));
#60549=CARTESIAN_POINT('Ctrl Pts',(12.4978126690739,-10.068355685636,0.000256951768887251));
#60550=CARTESIAN_POINT('Origin',(-2.04781266907391,0.,0.));
#60551=CARTESIAN_POINT('',(9.20218733092611,-10.0693573956675,-2.74992815830247E-5));
#60552=CARTESIAN_POINT('',(9.49781266907389,-10.0693547016817,1.23210960275731E-5));
#60553=CARTESIAN_POINT('',(-2.04781266907391,-10.0685,8.88799240754737E-13));
#60554=CARTESIAN_POINT('Ctrl Pts',(9.20218733092662,-10.0693573956667,-2.74992815838676E-5));
#60555=CARTESIAN_POINT('Ctrl Pts',(9.20280259561581,-10.069361467561,-0.025969271077885));
#60556=CARTESIAN_POINT('Ctrl Pts',(9.24310590125473,-10.0629317368011,-1.72529954123353));
#60557=CARTESIAN_POINT('Ctrl Pts',(9.32309724784339,-9.17795769784646,-5.09127456787318));
#60558=CARTESIAN_POINT('Ctrl Pts',(9.44216137069257,-5.62474557186012,-8.86105081131867));
#60559=CARTESIAN_POINT('Ctrl Pts',(9.56122549354177,-0.701216157947351,
-10.4720714344758));
#60560=CARTESIAN_POINT('Ctrl Pts',(9.68028961639095,4.39314562723144,-9.53185478943469));
#60561=CARTESIAN_POINT('Ctrl Pts',(9.79935373924015,8.41723617534466,-6.26945925877189));
#60562=CARTESIAN_POINT('Ctrl Pts',(9.91841786208933,10.3906945481397,-1.47967936938784));
#60563=CARTESIAN_POINT('Ctrl Pts',(10.0374819849385,9.83274093243286,3.67058442003326));
#60564=CARTESIAN_POINT('Ctrl Pts',(10.1565461077877,6.87930565177331,7.92660948819928));
#60565=CARTESIAN_POINT('Ctrl Pts',(10.2756102306369,2.24991341570653,10.2515303175065));
#60566=CARTESIAN_POINT('Ctrl Pts',(10.3946743534861,-2.92760943542397,10.0789427631348));
#60567=CARTESIAN_POINT('Ctrl Pts',(10.5137384763353,-7.39189934643209,7.450893119697));
#60568=CARTESIAN_POINT('Ctrl Pts',(10.6162428021488,-9.68491157861813,3.62561645258545));
#60569=CARTESIAN_POINT('Ctrl Pts',(10.6790590870126,-10.0673089391382,0.975499320207935));
#60570=CARTESIAN_POINT('Ctrl Pts',(10.7021873309266,-10.0677324747899,-0.000124116338529254));
#60571=CARTESIAN_POINT('Ctrl Pts',(9.49781266907388,-10.0693547016817,1.23210960274191E-5));
#60572=CARTESIAN_POINT('Ctrl Pts',(9.53713674256793,-10.069234798959,-1.65803352234717));
#60573=CARTESIAN_POINT('Ctrl Pts',(9.61606249472204,-9.23007000544182,-4.98594698332601));
#60574=CARTESIAN_POINT('Ctrl Pts',(9.73458992553625,-5.7418540840304,-8.78335034833538));
#60575=CARTESIAN_POINT('Ctrl Pts',(9.85339496151647,-0.85257594587396,-10.4589313947658));
#60576=CARTESIAN_POINT('Ctrl Pts',(9.97219999749669,4.24352503079001,-9.5973239487348));
#60577=CARTESIAN_POINT('Ctrl Pts',(10.0910050334769,8.31020699042318,-6.40754176265919));
#60578=CARTESIAN_POINT('Ctrl Pts',(10.2098100694571,10.3609505381623,-1.66338077710884));
#60579=CARTESIAN_POINT('Ctrl Pts',(10.3286151054374,9.89827436029318,3.48429280518479));
#60580=CARTESIAN_POINT('Ctrl Pts',(10.4474201414176,7.03441713875368,7.78672634564157));
#60581=CARTESIAN_POINT('Ctrl Pts',(10.5662251773978,2.46411003797023,10.2002104578618));
#60582=CARTESIAN_POINT('Ctrl Pts',(10.6850302133781,-2.70395522724915,10.1392681093327));
#60583=CARTESIAN_POINT('Ctrl Pts',(10.8038352493583,-7.21607928511531,7.61868304989973));
#60584=CARTESIAN_POINT('Ctrl Pts',(10.9080960679236,-9.63960661620993,3.78474211175173));
#60585=CARTESIAN_POINT('Ctrl Pts',(10.9727552078288,-10.06718250051,1.05677504796456));
#60586=CARTESIAN_POINT('Ctrl Pts',(10.9978126690739,-10.0678806802972,-0.000184627883194205));
#60587=CARTESIAN_POINT('Origin',(-2.04781266907391,0.,0.));
#60588=CARTESIAN_POINT('',(7.70218733092612,-10.0678139565754,0.000164567336945893));
#60589=CARTESIAN_POINT('',(7.99781266907388,-10.0678351491011,0.000168688374646564));
#60590=CARTESIAN_POINT('',(-2.04781266907391,-10.0685,8.88799240754737E-13));
#60591=CARTESIAN_POINT('Ctrl Pts',(7.70218733092662,-10.0678139565745,0.000164567336945823));
#60592=CARTESIAN_POINT('Ctrl Pts',(7.72654610421904,-10.0672163852583,-1.02734273559108));
#60593=CARTESIAN_POINT('Ctrl Pts',(7.7905929184612,-9.65592558851642,-3.72944759571061));
#60594=CARTESIAN_POINT('Ctrl Pts',(7.89432777365307,-7.27580489710256,-7.56430084860656));
#60595=CARTESIAN_POINT('Ctrl Pts',(8.01339189650228,-2.77141204137876,-10.1230064469915));
#60596=CARTESIAN_POINT('Ctrl Pts',(8.13245601935145,2.40816047958505,-10.2155150302614));
#60597=CARTESIAN_POINT('Ctrl Pts',(8.25152014220066,7.00104976392646,-7.81928938152035));
#60598=CARTESIAN_POINT('Ctrl Pts',(8.37058426504984,9.88832242924462,-3.51810513831368));
#60599=CARTESIAN_POINT('Ctrl Pts',(8.48964838789904,10.3665724996254,1.640170368877));
#60600=CARTESIAN_POINT('Ctrl Pts',(8.60871251074823,8.31928726688984,6.39886268018749));
#60601=CARTESIAN_POINT('Ctrl Pts',(8.72777663359742,4.2452324639752,9.59864498539987));
#60602=CARTESIAN_POINT('Ctrl Pts',(8.84684075644661,-0.863058530129139,
10.4599767782965));
#60603=CARTESIAN_POINT('Ctrl Pts',(8.96590487929581,-5.76108863167953,8.77301783919674));
#60604=CARTESIAN_POINT('Ctrl Pts',(9.08435373745581,-9.23752730731809,4.96851206513218));
#60605=CARTESIAN_POINT('Ctrl Pts',(9.16311455466607,-10.0690988074194,1.647421254088));
#60606=CARTESIAN_POINT('Ctrl Pts',(9.20218733092662,-10.0693573956667,-2.74992815838676E-5));
#60607=CARTESIAN_POINT('Ctrl Pts',(7.99781266907388,-10.0678351491011,0.000168688374646772));
#60608=CARTESIAN_POINT('Ctrl Pts',(8.02231491998694,-10.0672151254831,-1.03338480850318));
#60609=CARTESIAN_POINT('Ctrl Pts',(8.08641884956008,-9.65301482534439,-3.73790128031381));
#60610=CARTESIAN_POINT('Ctrl Pts',(8.19012445779329,-7.26905861171694,-7.56815159489579));
#60611=CARTESIAN_POINT('Ctrl Pts',(8.30892949377352,-2.77463030036995,-10.1201560442598));
#60612=CARTESIAN_POINT('Ctrl Pts',(8.42773452975374,2.39288398919242,-10.2171540987775));
#60613=CARTESIAN_POINT('Ctrl Pts',(8.54653956573398,6.97991854406481,-7.83561540544965));
#60614=CARTESIAN_POINT('Ctrl Pts',(8.66534460171419,9.87372380620264,-3.55326749101827));
#60615=CARTESIAN_POINT('Ctrl Pts',(8.78414963769443,10.3723036410682,1.59105274626059));
#60616=CARTESIAN_POINT('Ctrl Pts',(8.90295467367466,8.35470964850016,6.34940614177092));
#60617=CARTESIAN_POINT('Ctrl Pts',(9.02175970965488,4.31038153005013,9.56748361531403));
#60618=CARTESIAN_POINT('Ctrl Pts',(9.14056474563511,-0.779584044405554,
10.4646251906893));
#60619=CARTESIAN_POINT('Ctrl Pts',(9.25936978161534,-5.68043358093007,8.82319703942633));
#60620=CARTESIAN_POINT('Ctrl Pts',(9.37817481759556,-9.20329045551407,5.0413863624348));
#60621=CARTESIAN_POINT('Ctrl Pts',(9.45765578008175,-10.0664847388306,1.69317227532734));
#60622=CARTESIAN_POINT('Ctrl Pts',(9.49753506390785,-10.0693555481254,0.0117171637218366));
#60623=CARTESIAN_POINT('Ctrl Pts',(9.49781266907388,-10.0693547016817,1.23210960274191E-5));
#60624=CARTESIAN_POINT('Origin',(-2.04781266907391,0.,0.));
#60625=CARTESIAN_POINT('',(6.20218733092611,-10.0685983650411,-0.000257252931398383));
#60626=CARTESIAN_POINT('',(6.49781266907388,-10.0684276282593,-0.000258472074762262));
#60627=CARTESIAN_POINT('',(-2.04781266907391,-10.0685,8.88799240754737E-13));
#60628=CARTESIAN_POINT('Ctrl Pts',(6.20218733092662,-10.0685983650402,-0.000257252931398708));
#60629=CARTESIAN_POINT('Ctrl Pts',(6.21060157187254,-10.0689647571135,-0.355109286964507));
#60630=CARTESIAN_POINT('Ctrl Pts',(6.2587038537682,-9.96380652404249,-2.3835007597516));
#60631=CARTESIAN_POINT('Ctrl Pts',(6.34649417661359,-8.63574497305666,-5.96488834675535));
#60632=CARTESIAN_POINT('Ctrl Pts',(6.46555829946278,-4.73071828381995,-9.36890008208345));
#60633=CARTESIAN_POINT('Ctrl Pts',(6.58462242231197,0.326820099645189,-10.4904324434886));
#60634=CARTESIAN_POINT('Ctrl Pts',(6.70368654516116,5.30473759593165,-9.05625437293148));
#60635=CARTESIAN_POINT('Ctrl Pts',(6.82275066801036,8.99029910157828,-5.41576460835333));
#60636=CARTESIAN_POINT('Ctrl Pts',(6.94181479085954,10.4856171330745,-0.45587012131181));
#60637=CARTESIAN_POINT('Ctrl Pts',(7.06087891370874,9.42639785288965,4.61508480398452));
#60638=CARTESIAN_POINT('Ctrl Pts',(7.17994303655793,6.07069142041281,8.56169900820262));
#60639=CARTESIAN_POINT('Ctrl Pts',(7.29900715940712,1.23602504267618,10.4224865710064));
#60640=CARTESIAN_POINT('Ctrl Pts',(7.41807128225631,-3.89976544150229,9.74411687790103));
#60641=CARTESIAN_POINT('Ctrl Pts',(7.5371354051055,-8.0854834406099,6.69185637626472));
#60642=CARTESIAN_POINT('Ctrl Pts',(7.63184075466227,-9.84804949270156,2.96728702792277));
#60643=CARTESIAN_POINT('Ctrl Pts',(7.68685806326931,-10.068190015358,0.646787214435549));
#60644=CARTESIAN_POINT('Ctrl Pts',(7.70218733092662,-10.0678139565745,0.000164567336945823));
#60645=CARTESIAN_POINT('Ctrl Pts',(6.49781266907388,-10.0684276282593,-0.000258472074763094));
#60646=CARTESIAN_POINT('Ctrl Pts',(6.50749309740595,-10.0688389233335,-0.408529162113861));
#60647=CARTESIAN_POINT('Ctrl Pts',(6.5567752043981,-9.94479598934652,-2.48674672099571));
#60648=CARTESIAN_POINT('Ctrl Pts',(6.64565899005034,-8.54481685095021,-6.09116053372568));
#60649=CARTESIAN_POINT('Ctrl Pts',(6.76446402603055,-4.60070654709105,-9.43131119895073));
#60650=CARTESIAN_POINT('Ctrl Pts',(6.88326906201079,0.459469946313315,-10.4835594638622));
#60651=CARTESIAN_POINT('Ctrl Pts',(7.00207409799101,5.40818554410445,-8.99264481587256));
#60652=CARTESIAN_POINT('Ctrl Pts',(7.12087913397124,9.04495199435029,-5.32024201364924));
#60653=CARTESIAN_POINT('Ctrl Pts',(7.23968416995146,10.4875413103608,-0.357223917697587));
#60654=CARTESIAN_POINT('Ctrl Pts',(7.3584892059317,9.38600177395559,4.69245163674624));
#60655=CARTESIAN_POINT('Ctrl Pts',(7.47729424191192,6.00755126144244,8.6038049434562));
#60656=CARTESIAN_POINT('Ctrl Pts',(7.59609927789215,1.17175397485717,10.4279971368574));
#60657=CARTESIAN_POINT('Ctrl Pts',(7.71490431387238,-3.94829421545725,9.72250505024742));
#60658=CARTESIAN_POINT('Ctrl Pts',(7.83370934985261,-8.11054219940231,6.65847106291035));
#60659=CARTESIAN_POINT('Ctrl Pts',(7.92801213491977,-9.85264516588156,2.94423812985646));
#60660=CARTESIAN_POINT('Ctrl Pts',(7.98271324132686,-10.0682172365206,0.637092471587673));
#60661=CARTESIAN_POINT('Ctrl Pts',(7.99781266907388,-10.0678351491011,0.000168688374646772));
#60662=CARTESIAN_POINT('Origin',(-2.04781266907391,0.,0.));
#60663=CARTESIAN_POINT('',(4.70218733092611,-10.0687162765567,0.00024819917633277));
#60664=CARTESIAN_POINT('',(4.99781266907388,-10.0690106407173,0.000197091441647979));
#60665=CARTESIAN_POINT('',(-2.04781266907391,-10.0685,8.88799240754737E-13));
#60666=CARTESIAN_POINT('Ctrl Pts',(4.70218733092661,-10.0687162765559,0.000248199176332876));
#60667=CARTESIAN_POINT('Ctrl Pts',(4.73434508047578,-10.0673293742563,-1.35588812249017));
#60668=CARTESIAN_POINT('Ctrl Pts',(4.80619087097467,-9.4509651757737,-4.38694580302619));
#60669=CARTESIAN_POINT('Ctrl Pts',(4.91772470242328,-6.50073919290531,-8.23992561706452));
#60670=CARTESIAN_POINT('Ctrl Pts',(5.03678882527248,-1.76759699461112,-10.3456070432611));
#60671=CARTESIAN_POINT('Ctrl Pts',(5.15585294812166,3.39617245408182,-9.93086083333501));
#60672=CARTESIAN_POINT('Ctrl Pts',(5.27491707097087,7.73255624289876,-7.09672869562723));
#60673=CARTESIAN_POINT('Ctrl Pts',(5.39398119382005,10.1851116230995,-2.53367035226248));
#60674=CARTESIAN_POINT('Ctrl Pts',(5.51304531666925,10.1563397399983,2.64664831714824));
#60675=CARTESIAN_POINT('Ctrl Pts',(5.63210943951844,7.65325008554719,7.18218263183298));
#60676=CARTESIAN_POINT('Ctrl Pts',(5.75117356236763,3.28565282500688,9.96797219811811));
#60677=CARTESIAN_POINT('Ctrl Pts',(5.87023768521683,-1.8824049738298,10.3253346552754));
#60678=CARTESIAN_POINT('Ctrl Pts',(5.989301808066,-6.59186566003927,8.16720829591889));
#60679=CARTESIAN_POINT('Ctrl Pts',(6.09995168996929,-9.476070400193,4.31248985718041));
#60680=CARTESIAN_POINT('Ctrl Pts',(6.17091353092281,-10.0672365699004,1.31864621258765));
#60681=CARTESIAN_POINT('Ctrl Pts',(6.20218733092662,-10.0685983650402,-0.000257252931398708));
#60682=CARTESIAN_POINT('Ctrl Pts',(4.99781266907388,-10.0690106407173,0.000197091441647562));
#60683=CARTESIAN_POINT('Ctrl Pts',(5.03227295348504,-10.0677201749372,-1.45291781706314));
#60684=CARTESIAN_POINT('Ctrl Pts',(5.10633491655628,-9.38403346435216,-4.5771238626216));
#60685=CARTESIAN_POINT('Ctrl Pts',(5.21999855828759,-6.26763830931662,-8.41622490713541));
#60686=CARTESIAN_POINT('Ctrl Pts',(5.33880359426783,-1.48983776572259,-10.387324732371));
#60687=CARTESIAN_POINT('Ctrl Pts',(5.45760863024804,3.64937630016661,-9.83860682635921));
#60688=CARTESIAN_POINT('Ctrl Pts',(5.57641366622829,7.90330340852995,-6.90318237457325));
#60689=CARTESIAN_POINT('Ctrl Pts',(5.6952187022085,10.2400011457753,-2.29314373697339));
#60690=CARTESIAN_POINT('Ctrl Pts',(5.81402373818874,10.092619765449,2.87317906402775));
#60691=CARTESIAN_POINT('Ctrl Pts',(5.93282877416896,7.49691190116663,7.34250935375952));
#60692=CARTESIAN_POINT('Ctrl Pts',(6.05163381014919,3.08255948452053,10.0306509603461));
#60693=CARTESIAN_POINT('Ctrl Pts',(6.17043884612943,-2.07957816526778,10.285498836636));
#60694=CARTESIAN_POINT('Ctrl Pts',(6.28924388210963,-6.73723963188388,8.0452305005185));
#60695=CARTESIAN_POINT('Ctrl Pts',(6.39836848975781,-9.51419863391599,4.19486836671947));
#60696=CARTESIAN_POINT('Ctrl Pts',(6.46789141874588,-10.0671563557027,1.26166601093287));
#60697=CARTESIAN_POINT('Ctrl Pts',(6.49781266907388,-10.0684276282593,-0.000258472074763094));
#60698=CARTESIAN_POINT('Origin',(-2.04781266907391,0.,0.));
#60699=CARTESIAN_POINT('',(3.20218733092611,-10.0677530223773,-0.000135991633093525));
#60700=CARTESIAN_POINT('',(3.49781266907387,-10.0676463066001,-6.32822640955766E-6));
#60701=CARTESIAN_POINT('',(-2.04781266907391,-10.0685,8.88799240754737E-13));
#60702=CARTESIAN_POINT('Ctrl Pts',(3.20218733092662,-10.0677530223764,-0.000135991633093968));
#60703=CARTESIAN_POINT('Ctrl Pts',(3.21840054812928,-10.0680791684123,-0.684057449144463));
#60704=CARTESIAN_POINT('Ctrl Pts',(3.27430180628167,-9.83131823889777,-3.04191515837554));
#60705=CARTESIAN_POINT('Ctrl Pts',(3.36989110538379,-8.01065275437778,-6.78125553845112));
#60706=CARTESIAN_POINT('Ctrl Pts',(3.48895522823299,-3.79128906016513,-9.78683357839978));
#60707=CARTESIAN_POINT('Ctrl Pts',(3.60801935108218,1.35171977960818,-10.4081140398368));
#60708=CARTESIAN_POINT('Ctrl Pts',(3.72708347393137,6.16541861617209,-8.49373872428129));
#60709=CARTESIAN_POINT('Ctrl Pts',(3.84614759678056,9.47707978558044,-4.51009345431341));
#60710=CARTESIAN_POINT('Ctrl Pts',(3.96521171962975,10.4799065191379,0.572314231060847));
#60711=CARTESIAN_POINT('Ctrl Pts',(4.08427584247894,8.92958717780655,5.51529301695582));
#60712=CARTESIAN_POINT('Ctrl Pts',(4.20333996532814,5.20381518222463,9.11461967271146));
#60713=CARTESIAN_POINT('Ctrl Pts',(4.32240408817732,0.210274215357055,10.4934155060823));
#60714=CARTESIAN_POINT('Ctrl Pts',(4.44146821102652,-4.83449438284527,9.31577416488656));
#60715=CARTESIAN_POINT('Ctrl Pts',(4.56053233387571,-8.70146904413809,5.86859614412498));
#60716=CARTESIAN_POINT('Ctrl Pts',(4.64743870717574,-9.97669658877405,2.3088844955255));
#60717=CARTESIAN_POINT('Ctrl Pts',(4.69465703952604,-10.0690410436371,0.31781089632451));
#60718=CARTESIAN_POINT('Ctrl Pts',(4.70218733092661,-10.0687162765559,0.000248199176332876));
#60719=CARTESIAN_POINT('Ctrl Pts',(3.49781266907388,-10.0676463066001,-6.32822640948827E-6));
#60720=CARTESIAN_POINT('Ctrl Pts',(3.51745113090405,-10.0676645129864,-0.828440043131245));
#60721=CARTESIAN_POINT('Ctrl Pts',(3.57669127139431,-9.76268316383691,-3.32742756187295));
#60722=CARTESIAN_POINT('Ctrl Pts',(3.67553309054464,-7.71776422714997,-7.11001033739966));
#60723=CARTESIAN_POINT('Ctrl Pts',(3.79433812652486,-3.38761003189172,-9.93177879011561));
#60724=CARTESIAN_POINT('Ctrl Pts',(3.9131431625051,1.76433033496111,-10.3442384994258));
#60725=CARTESIAN_POINT('Ctrl Pts',(4.03194819848532,6.48826917337762,-8.24733258682529));
#60726=CARTESIAN_POINT('Ctrl Pts',(4.15075323446555,9.63824588685654,-4.14974070134389));
#60727=CARTESIAN_POINT('Ctrl Pts',(4.26955827044577,10.4501207782042,0.954519452312438));
#60728=CARTESIAN_POINT('Ctrl Pts',(4.38836330642601,8.72694450777083,5.82722671793283));
#60729=CARTESIAN_POINT('Ctrl Pts',(4.50716834240623,4.88673521132993,9.28633138748812));
#60730=CARTESIAN_POINT('Ctrl Pts',(4.62597337838646,-0.138926773910176,
10.4927037037835));
#60731=CARTESIAN_POINT('Ctrl Pts',(4.74477841436669,-5.13088709320036,9.15369484419977));
#60732=CARTESIAN_POINT('Ctrl Pts',(4.86358345034691,-8.87816693820219,5.59412937652621));
#60733=CARTESIAN_POINT('Ctrl Pts',(4.94792820191598,-10.009504711213,2.10361019298977));
#60734=CARTESIAN_POINT('Ctrl Pts',(4.99267127482497,-10.0692031752089,0.21699845455443));
#60735=CARTESIAN_POINT('Ctrl Pts',(4.99781266907388,-10.0690106407173,0.000197091441647562));
#60736=CARTESIAN_POINT('Origin',(-2.04781266907391,0.,0.));
#60737=CARTESIAN_POINT('',(1.70218733092611,-10.069362524867,-1.19920097210299E-5));
#60738=CARTESIAN_POINT('',(1.99781266907388,-10.0690473037901,-0.000187867633422711));
#60739=CARTESIAN_POINT('',(-2.04781266907391,-10.0685,8.88799240754737E-13));
#60740=CARTESIAN_POINT('Ctrl Pts',(1.70218733092661,-10.0693625248661,-1.1992009720295E-5));
#60741=CARTESIAN_POINT('Ctrl Pts',(1.70245601578278,-10.0693633221876,-0.0113406947917886));
#60742=CARTESIAN_POINT('Ctrl Pts',(1.74241274158867,-10.0665796830594,-1.69605702657895));
#60743=CARTESIAN_POINT('Ctrl Pts',(1.8220575083443,-9.20004427129698,-5.05125418271118));
#60744=CARTESIAN_POINT('Ctrl Pts',(1.94112163119349,-5.6632842472853,-8.83646963134304));
#60745=CARTESIAN_POINT('Ctrl Pts',(2.06018575404269,-0.74681783530992,-10.4689181755661));
#60746=CARTESIAN_POINT('Ctrl Pts',(2.17924987689187,4.35159046461578,-9.55089756705936));
#60747=CARTESIAN_POINT('Ctrl Pts',(2.29831399974107,8.38985137183536,-6.30605886170975));
#60748=CARTESIAN_POINT('Ctrl Pts',(2.41737812259025,10.3841516444387,-1.52491926888339));
#60749=CARTESIAN_POINT('Ctrl Pts',(2.53644224543945,9.84863394411602,3.62772569058057));
#60750=CARTESIAN_POINT('Ctrl Pts',(2.65550636828864,6.91376266876593,7.89657330678198));
#60751=CARTESIAN_POINT('Ctrl Pts',(2.77457049113784,2.29453992050261,10.2416341848227));
#60752=CARTESIAN_POINT('Ctrl Pts',(2.89363461398702,-2.88368548691312,10.0915976062867));
#60753=CARTESIAN_POINT('Ctrl Pts',(3.01269873683622,-7.35937883651767,7.48301592715619));
#60754=CARTESIAN_POINT('Ctrl Pts',(3.11554964248275,-9.67683852224496,3.65486230485631));
#60755=CARTESIAN_POINT('Ctrl Pts',(3.17871250717955,-10.0672808014341,0.990101508502404));
#60756=CARTESIAN_POINT('Ctrl Pts',(3.20218733092662,-10.0677530223764,-0.000135991633093968));
#60757=CARTESIAN_POINT('Ctrl Pts',(1.99781266907388,-10.0690473037901,-0.000187867633422503));
#60758=CARTESIAN_POINT('Ctrl Pts',(2.00262930832307,-10.0692215762849,-0.203292878761537));
#60759=CARTESIAN_POINT('Ctrl Pts',(2.04704762623233,-10.0137050096471,-2.07620136021942));
#60760=CARTESIAN_POINT('Ctrl Pts',(2.13106762280168,-8.90092254260253,-5.55785119946268));
#60761=CARTESIAN_POINT('Ctrl Pts',(2.2498726587819,-5.16820041446581,-9.13267955350996));
#60762=CARTESIAN_POINT('Ctrl Pts',(2.36867769476214,-0.181746135518434,
-10.4920493795623));
#60763=CARTESIAN_POINT('Ctrl Pts',(2.48748273074236,4.84879718275033,-9.30619672407481));
#60764=CARTESIAN_POINT('Ctrl Pts',(2.60628776672259,8.70309103847143,-5.86279268462035));
#60765=CARTESIAN_POINT('Ctrl Pts',(2.72509280270281,10.4461383825637,-0.997158240267306));
#60766=CARTESIAN_POINT('Ctrl Pts',(2.84389783868305,9.65510063715378,4.11037265272831));
#60767=CARTESIAN_POINT('Ctrl Pts',(2.96270287466327,6.52187234635328,8.22078541060934));
#60768=CARTESIAN_POINT('Ctrl Pts',(3.0815079106435,1.80653027708299,10.3369521629193));
#60769=CARTESIAN_POINT('Ctrl Pts',(3.20031294662373,-3.3470504283007,9.94552085593946));
#60770=CARTESIAN_POINT('Ctrl Pts',(3.31911798260395,-7.68868414698893,7.14144717485069));
#60771=CARTESIAN_POINT('Ctrl Pts',(3.418284556754,-9.75579215615403,3.3548406284196));
#60772=CARTESIAN_POINT('Ctrl Pts',(3.47784945224398,-10.0676277991405,0.842126931641699));
#60773=CARTESIAN_POINT('Ctrl Pts',(3.49781266907388,-10.0676463066001,-6.32822640948827E-6));
#60774=CARTESIAN_POINT('Ctrl Pts',(149.800942407062,42.7797111789148,1.66533453693773E-15));
#60775=CARTESIAN_POINT('Ctrl Pts',(149.800942407062,42.7797111789148,6.39954382888827));
#60776=CARTESIAN_POINT('Ctrl Pts',(149.800942407062,39.863341598027,19.1970122769317));
#60777=CARTESIAN_POINT('Ctrl Pts',(149.800942407062,28.946492695985,32.8750119363481));
#60778=CARTESIAN_POINT('Ctrl Pts',(149.800942407062,15.8639072776604,40.4205994697869));
#60779=CARTESIAN_POINT('Ctrl Pts',(149.800942407062,3.24590135017625,43.301577152732));
#60780=CARTESIAN_POINT('Ctrl Pts',(149.800942407062,-9.66246509364301,42.3352179983522));
#60781=CARTESIAN_POINT('Ctrl Pts',(149.800942407062,-21.7112177724829,37.6059878389314));
#60782=CARTESIAN_POINT('Ctrl Pts',(149.800942407062,-31.8309343700387,29.5353382462332));
#60783=CARTESIAN_POINT('Ctrl Pts',(149.800942407062,-39.122456989573,18.840983833502));
#60784=CARTESIAN_POINT('Ctrl Pts',(149.800942407062,-42.9388386664135,6.47217930280024));
#60785=CARTESIAN_POINT('Ctrl Pts',(149.800942407062,-42.9375051905117,-6.47131760733891));
#60786=CARTESIAN_POINT('Ctrl Pts',(149.800942407062,-39.124073437403,-18.840591107856));
#60787=CARTESIAN_POINT('Ctrl Pts',(149.800942407062,-31.8314962733083,-29.5357296654429));
#60788=CARTESIAN_POINT('Ctrl Pts',(149.800942407062,-21.7119250540969,-37.6042252482423));
#60789=CARTESIAN_POINT('Ctrl Pts',(149.800942407062,-11.6699958492274,-41.5482999069467));
#60790=CARTESIAN_POINT('Ctrl Pts',(149.800942407062,-3.20970073774902,-42.8162553642041));
#60791=CARTESIAN_POINT('Ctrl Pts',(149.800942407062,9.63353641205357,-42.8436296395881));
#60792=CARTESIAN_POINT('Ctrl Pts',(149.800942407062,26.2255697150551,-36.3220340248293));
#60793=CARTESIAN_POINT('Ctrl Pts',(149.800942407062,39.8583355435163,-19.1842701722528));
#60794=CARTESIAN_POINT('Ctrl Pts',(149.800942407062,42.7797111789148,-6.39954382888828));
#60795=CARTESIAN_POINT('Ctrl Pts',(149.800942407062,42.7797111789148,-1.11022302462516E-15));
#60796=CARTESIAN_POINT('Ctrl Pts',(149.929058852228,42.6083285177578,1.6044350367448E-15));
#60797=CARTESIAN_POINT('Ctrl Pts',(149.929058852228,42.6083285177578,6.37393351687803));
#60798=CARTESIAN_POINT('Ctrl Pts',(149.929058852228,39.7036566731736,19.1201007008175));
#60799=CARTESIAN_POINT('Ctrl Pts',(149.929058852228,28.8305409178108,32.7433162931913));
#60800=CARTESIAN_POINT('Ctrl Pts',(149.929058852228,15.8003735948979,40.2586747848402));
#60801=CARTESIAN_POINT('Ctrl Pts',(149.929058852228,3.2328979919691,43.128112374127));
#60802=CARTESIAN_POINT('Ctrl Pts',(149.929058852228,-9.62376090884556,42.1656288257134));
#60803=CARTESIAN_POINT('Ctrl Pts',(149.929058852228,-21.6242408141415,37.4553429755425));
#60804=CARTESIAN_POINT('Ctrl Pts',(149.929058852228,-31.70343097621,29.417016729647));
#60805=CARTESIAN_POINT('Ctrl Pts',(149.929058852228,-38.9657377435684,18.7655047447997));
#60806=CARTESIAN_POINT('Ctrl Pts',(149.929058852228,-42.7668318717438,6.44626702799623));
#60807=CARTESIAN_POINT('Ctrl Pts',(149.929058852228,-42.7654990928386,-6.44539485123875));
#60808=CARTESIAN_POINT('Ctrl Pts',(149.929058852228,-38.9673466917161,-18.7651207412867));
#60809=CARTESIAN_POINT('Ctrl Pts',(149.929058852228,-31.7039876586539,-29.4174081300967));
#60810=CARTESIAN_POINT('Ctrl Pts',(149.929058852228,-21.624937316283,-37.4535929374206));
#60811=CARTESIAN_POINT('Ctrl Pts',(149.929058852228,-11.6232588436889,-41.3818583960817));
#60812=CARTESIAN_POINT('Ctrl Pts',(149.929058852228,-3.19684006364051,-42.6447363292776));
#60813=CARTESIAN_POINT('Ctrl Pts',(149.929058852228,9.59495902491427,-42.6720001774473));
#60814=CARTESIAN_POINT('Ctrl Pts',(149.929058852228,26.1205158346157,-36.1765312663764));
#60815=CARTESIAN_POINT('Ctrl Pts',(149.929058852228,39.698671634606,-19.107410283042));
#60816=CARTESIAN_POINT('Ctrl Pts',(149.929058852228,42.6083285177578,-6.37393351687802));
#60817=CARTESIAN_POINT('Ctrl Pts',(149.929058852228,42.6083285177578,-1.11924517280189E-15));
#60818=CARTESIAN_POINT('Ctrl Pts',(150.,42.3949460423634,1.34680329382573E-15));
#60819=CARTESIAN_POINT('Ctrl Pts',(150.,42.3949460423634,6.34200576304127));
#60820=CARTESIAN_POINT('Ctrl Pts',(150.,39.5048170839467,19.0243485874962));
#60821=CARTESIAN_POINT('Ctrl Pts',(150.,28.686154291952,32.5793359361951));
#60822=CARTESIAN_POINT('Ctrl Pts',(150.,15.7212401985096,40.0570575598128));
#60823=CARTESIAN_POINT('Ctrl Pts',(150.,3.21670757275077,42.9121245965004));
#60824=CARTESIAN_POINT('Ctrl Pts',(150.,-9.57556375463445,41.9544600711998));
#60825=CARTESIAN_POINT('Ctrl Pts',(150.,-21.5159461649562,37.2677637901972));
#60826=CARTESIAN_POINT('Ctrl Pts',(150.,-31.5446558958809,29.2696958196848));
#60827=CARTESIAN_POINT('Ctrl Pts',(150.,-38.7705942826772,18.6715268427006));
#60828=CARTESIAN_POINT('Ctrl Pts',(150.,-42.552652141369,6.41397987874088));
#60829=CARTESIAN_POINT('Ctrl Pts',(150.,-42.5513272438122,-6.41311568970265));
#60830=CARTESIAN_POINT('Ctrl Pts',(150.,-38.7721954392263,-18.6711429050351));
#60831=CARTESIAN_POINT('Ctrl Pts',(150.,-31.5452105619922,-29.2700848574892));
#60832=CARTESIAN_POINT('Ctrl Pts',(150.,-21.5166412433614,-37.2660210896304));
#60833=CARTESIAN_POINT('Ctrl Pts',(150.,-11.5650456899347,-41.1746160267573));
#60834=CARTESIAN_POINT('Ctrl Pts',(150.,-3.18083083083891,-42.431168918257));
#60835=CARTESIAN_POINT('Ctrl Pts',(150.,9.546903277546,-42.4582964268803));
#60836=CARTESIAN_POINT('Ctrl Pts',(150.,25.9897016808724,-35.995356792079));
#60837=CARTESIAN_POINT('Ctrl Pts',(150.,39.499856760821,-19.011721557077));
#60838=CARTESIAN_POINT('Ctrl Pts',(150.,42.3949460423634,-6.34200576304127));
#60839=CARTESIAN_POINT('Ctrl Pts',(150.,42.3949460423634,-1.12824228447505E-15));
#60840=CARTESIAN_POINT('Ctrl Pts',(150.,42.180969781841,9.42431733411802E-16));
#60841=CARTESIAN_POINT('Ctrl Pts',(150.,42.180969781841,6.30997632814664));
#60842=CARTESIAN_POINT('Ctrl Pts',(150.,39.3054174750564,18.9283324370361));
#60843=CARTESIAN_POINT('Ctrl Pts',(150.,28.5413599122526,32.4148959132814));
#60844=CARTESIAN_POINT('Ctrl Pts',(150.,15.6418773072674,39.854876010461));
#60845=CARTESIAN_POINT('Ctrl Pts',(150.,3.20047197593293,42.6955317614601));
#60846=CARTESIAN_POINT('Ctrl Pts',(150.,-9.52723000930247,41.742697692085));
#60847=CARTESIAN_POINT('Ctrl Pts',(150.,-21.4073493146782,37.079657457624));
#60848=CARTESIAN_POINT('Ctrl Pts',(150.,-31.3854311726194,29.1219640275379));
#60849=CARTESIAN_POINT('Ctrl Pts',(150.,-38.5749022279962,18.5772869390667));
#60850=CARTESIAN_POINT('Ctrl Pts',(150.,-42.3378701338226,6.38159520180752));
#60851=CARTESIAN_POINT('Ctrl Pts',(150.,-42.3365553211424,-6.38074556656657));
#60852=CARTESIAN_POINT('Ctrl Pts',(150.,-38.5764960521524,-18.5768997099774));
#60853=CARTESIAN_POINT('Ctrl Pts',(150.,-31.3859852115361,-29.1223499684757));
#60854=CARTESIAN_POINT('Ctrl Pts',(150.,-21.4080466972356,-37.0779195360124));
#60855=CARTESIAN_POINT('Ctrl Pts',(150.,-11.5066635258887,-40.9667932429984));
#60856=CARTESIAN_POINT('Ctrl Pts',(150.,-3.16477802436578,-42.2170024976521));
#60857=CARTESIAN_POINT('Ctrl Pts',(150.,9.49870621121396,-42.2439936448794));
#60858=CARTESIAN_POINT('Ctrl Pts',(150.,25.8585187505318,-35.8136737578412));
#60859=CARTESIAN_POINT('Ctrl Pts',(150.,39.300481484882,-18.9157686698295));
#60860=CARTESIAN_POINT('Ctrl Pts',(150.,42.180969781841,-6.30997632814663));
#60861=CARTESIAN_POINT('Ctrl Pts',(150.,42.180969781841,-1.13546850555259E-15));
#60862=CARTESIAN_POINT('',(150.,42.180969781841,-1.11022302462516E-15));
#60863=CARTESIAN_POINT('',(149.800942407062,42.7797111789149,-5.55111512312578E-16));
#60864=CARTESIAN_POINT('Origin',(149.,42.180969781841,-1.11022302462516E-15));
#60865=CARTESIAN_POINT('Ctrl Pts',(149.800942407062,42.7797111789148,1.66533453693773E-15));
#60866=CARTESIAN_POINT('Ctrl Pts',(149.800942407062,42.7797111789148,6.39954382888827));
#60867=CARTESIAN_POINT('Ctrl Pts',(149.800942407062,39.863341598027,19.1970122769317));
#60868=CARTESIAN_POINT('Ctrl Pts',(149.800942407062,28.946492695985,32.8750119363481));
#60869=CARTESIAN_POINT('Ctrl Pts',(149.800942407062,15.8639072776604,40.4205994697869));
#60870=CARTESIAN_POINT('Ctrl Pts',(149.800942407062,3.24590135017625,43.301577152732));
#60871=CARTESIAN_POINT('Ctrl Pts',(149.800942407062,-9.66246509364301,42.3352179983522));
#60872=CARTESIAN_POINT('Ctrl Pts',(149.800942407062,-21.7112177724829,37.6059878389314));
#60873=CARTESIAN_POINT('Ctrl Pts',(149.800942407062,-31.8309343700387,29.5353382462332));
#60874=CARTESIAN_POINT('Ctrl Pts',(149.800942407062,-39.122456989573,18.840983833502));
#60875=CARTESIAN_POINT('Ctrl Pts',(149.800942407062,-42.9388386664135,6.47217930280024));
#60876=CARTESIAN_POINT('Ctrl Pts',(149.800942407062,-42.9375051905117,-6.47131760733891));
#60877=CARTESIAN_POINT('Ctrl Pts',(149.800942407062,-39.124073437403,-18.840591107856));
#60878=CARTESIAN_POINT('Ctrl Pts',(149.800942407062,-31.8314962733083,-29.5357296654429));
#60879=CARTESIAN_POINT('Ctrl Pts',(149.800942407062,-21.7119250540969,-37.6042252482423));
#60880=CARTESIAN_POINT('Ctrl Pts',(149.800942407062,-11.6699958492274,-41.5482999069467));
#60881=CARTESIAN_POINT('Ctrl Pts',(149.800942407062,-3.20970073774902,-42.8162553642041));
#60882=CARTESIAN_POINT('Ctrl Pts',(149.800942407062,9.63353641205357,-42.8436296395881));
#60883=CARTESIAN_POINT('Ctrl Pts',(149.800942407062,26.2255697150551,-36.3220340248293));
#60884=CARTESIAN_POINT('Ctrl Pts',(149.800942407062,39.8583355435163,-19.1842701722528));
#60885=CARTESIAN_POINT('Ctrl Pts',(149.800942407062,42.7797111789148,-6.39954382888828));
#60886=CARTESIAN_POINT('Ctrl Pts',(149.800942407062,42.7797111789148,-1.11022302462516E-15));
#60887=CARTESIAN_POINT('Ctrl Pts',(150.,42.180969781841,-1.13546850555259E-15));
#60888=CARTESIAN_POINT('Ctrl Pts',(150.,42.180969781841,-6.30997632814663));
#60889=CARTESIAN_POINT('Ctrl Pts',(150.,39.300481484882,-18.9157686698295));
#60890=CARTESIAN_POINT('Ctrl Pts',(150.,25.8585187505318,-35.8136737578412));
#60891=CARTESIAN_POINT('Ctrl Pts',(150.,9.49870621121396,-42.2439936448794));
#60892=CARTESIAN_POINT('Ctrl Pts',(150.,-3.16477802436578,-42.2170024976521));
#60893=CARTESIAN_POINT('Ctrl Pts',(150.,-11.5066635258887,-40.9667932429984));
#60894=CARTESIAN_POINT('Ctrl Pts',(150.,-21.4080466972356,-37.0779195360124));
#60895=CARTESIAN_POINT('Ctrl Pts',(150.,-31.3859852115361,-29.1223499684757));
#60896=CARTESIAN_POINT('Ctrl Pts',(150.,-38.5764960521524,-18.5768997099774));
#60897=CARTESIAN_POINT('Ctrl Pts',(150.,-42.3365553211424,-6.38074556656657));
#60898=CARTESIAN_POINT('Ctrl Pts',(150.,-42.3378701338226,6.38159520180752));
#60899=CARTESIAN_POINT('Ctrl Pts',(150.,-38.5749022279962,18.5772869390667));
#60900=CARTESIAN_POINT('Ctrl Pts',(150.,-31.3854311726194,29.1219640275379));
#60901=CARTESIAN_POINT('Ctrl Pts',(150.,-21.4073493146782,37.079657457624));
#60902=CARTESIAN_POINT('Ctrl Pts',(150.,-9.52723000930247,41.742697692085));
#60903=CARTESIAN_POINT('Ctrl Pts',(150.,3.20047197593293,42.6955317614601));
#60904=CARTESIAN_POINT('Ctrl Pts',(150.,15.6418773072674,39.854876010461));
#60905=CARTESIAN_POINT('Ctrl Pts',(150.,28.5413599122526,32.4148959132814));
#60906=CARTESIAN_POINT('Ctrl Pts',(150.,39.3054174750564,18.9283324370361));
#60907=CARTESIAN_POINT('Ctrl Pts',(150.,42.180969781841,6.30997632814664));
#60908=CARTESIAN_POINT('Ctrl Pts',(150.,42.180969781841,9.42431733411802E-16));
#60909=CARTESIAN_POINT('Ctrl Pts',(150.,42.5,0.));
#60910=CARTESIAN_POINT('Ctrl Pts',(150.,42.5,42.5));
#60911=CARTESIAN_POINT('Ctrl Pts',(150.,0.,42.5));
#60912=CARTESIAN_POINT('Ctrl Pts',(150.,-42.5,42.5));
#60913=CARTESIAN_POINT('Ctrl Pts',(150.,-42.5,0.));
#60914=CARTESIAN_POINT('Ctrl Pts',(150.,-42.5,-42.5));
#60915=CARTESIAN_POINT('Ctrl Pts',(150.,0.,-42.5));
#60916=CARTESIAN_POINT('Ctrl Pts',(150.,42.5,-42.5));
#60917=CARTESIAN_POINT('Ctrl Pts',(150.,42.5,0.));
#60918=CARTESIAN_POINT('Ctrl Pts',(149.933965156713,42.5974709813122,0.));
#60919=CARTESIAN_POINT('Ctrl Pts',(149.933965156713,42.5974709813122,42.5974709813122));
#60920=CARTESIAN_POINT('Ctrl Pts',(149.933965156713,0.,42.5974709813122));
#60921=CARTESIAN_POINT('Ctrl Pts',(149.933965156713,-42.5974709813122,42.5974709813122));
#60922=CARTESIAN_POINT('Ctrl Pts',(149.933965156713,-42.5974709813122,0.));
#60923=CARTESIAN_POINT('Ctrl Pts',(149.933965156713,-42.5974709813122,-42.5974709813122));
#60924=CARTESIAN_POINT('Ctrl Pts',(149.933965156713,0.,-42.5974709813122));
#60925=CARTESIAN_POINT('Ctrl Pts',(149.933965156713,42.5974709813122,-42.5974709813122));
#60926=CARTESIAN_POINT('Ctrl Pts',(149.933965156713,42.5974709813122,0.));
#60927=CARTESIAN_POINT('Ctrl Pts',(149.798898307353,42.7886652078195,0.));
#60928=CARTESIAN_POINT('Ctrl Pts',(149.798898307353,42.7886652078195,42.7886652078195));
#60929=CARTESIAN_POINT('Ctrl Pts',(149.798898307353,0.,42.7886652078195));
#60930=CARTESIAN_POINT('Ctrl Pts',(149.798898307353,-42.7886652078195,42.7886652078195));
#60931=CARTESIAN_POINT('Ctrl Pts',(149.798898307353,-42.7886652078195,0.));
#60932=CARTESIAN_POINT('Ctrl Pts',(149.798898307353,-42.7886652078195,-42.7886652078195));
#60933=CARTESIAN_POINT('Ctrl Pts',(149.798898307353,0.,-42.7886652078195));
#60934=CARTESIAN_POINT('Ctrl Pts',(149.798898307353,42.7886652078195,-42.7886652078195));
#60935=CARTESIAN_POINT('Ctrl Pts',(149.798898307353,42.7886652078195,0.));
#60936=CARTESIAN_POINT('Ctrl Pts',(149.587306656495,43.0642134786981,0.));
#60937=CARTESIAN_POINT('Ctrl Pts',(149.587306656495,43.0642134786981,43.0642134786981));
#60938=CARTESIAN_POINT('Ctrl Pts',(149.587306656495,0.,43.0642134786981));
#60939=CARTESIAN_POINT('Ctrl Pts',(149.587306656495,-43.0642134786981,43.0642134786981));
#60940=CARTESIAN_POINT('Ctrl Pts',(149.587306656495,-43.0642134786981,0.));
#60941=CARTESIAN_POINT('Ctrl Pts',(149.587306656495,-43.0642134786981,-43.0642134786981));
#60942=CARTESIAN_POINT('Ctrl Pts',(149.587306656495,0.,-43.0642134786981));
#60943=CARTESIAN_POINT('Ctrl Pts',(149.587306656495,43.0642134786981,-43.0642134786981));
#60944=CARTESIAN_POINT('Ctrl Pts',(149.587306656495,43.0642134786981,0.));
#60945=CARTESIAN_POINT('Ctrl Pts',(149.286904889827,43.4087538935563,0.));
#60946=CARTESIAN_POINT('Ctrl Pts',(149.286904889827,43.4087538935563,43.4087538935563));
#60947=CARTESIAN_POINT('Ctrl Pts',(149.286904889827,0.,43.4087538935563));
#60948=CARTESIAN_POINT('Ctrl Pts',(149.286904889827,-43.4087538935563,43.4087538935563));
#60949=CARTESIAN_POINT('Ctrl Pts',(149.286904889827,-43.4087538935563,0.));
#60950=CARTESIAN_POINT('Ctrl Pts',(149.286904889827,-43.4087538935563,-43.4087538935563));
#60951=CARTESIAN_POINT('Ctrl Pts',(149.286904889827,0.,-43.4087538935563));
#60952=CARTESIAN_POINT('Ctrl Pts',(149.286904889827,43.4087538935563,-43.4087538935563));
#60953=CARTESIAN_POINT('Ctrl Pts',(149.286904889827,43.4087538935563,0.));
#60954=CARTESIAN_POINT('Ctrl Pts',(148.878896254171,43.7987824668423,0.));
#60955=CARTESIAN_POINT('Ctrl Pts',(148.878896254171,43.7987824668423,43.7987824668423));
#60956=CARTESIAN_POINT('Ctrl Pts',(148.878896254171,0.,43.7987824668423));
#60957=CARTESIAN_POINT('Ctrl Pts',(148.878896254171,-43.7987824668423,43.7987824668423));
#60958=CARTESIAN_POINT('Ctrl Pts',(148.878896254171,-43.7987824668423,0.));
#60959=CARTESIAN_POINT('Ctrl Pts',(148.878896254171,-43.7987824668423,-43.7987824668423));
#60960=CARTESIAN_POINT('Ctrl Pts',(148.878896254171,0.,-43.7987824668423));
#60961=CARTESIAN_POINT('Ctrl Pts',(148.878896254171,43.7987824668423,-43.7987824668423));
#60962=CARTESIAN_POINT('Ctrl Pts',(148.878896254171,43.7987824668423,0.));
#60963=CARTESIAN_POINT('Ctrl Pts',(148.435583321827,44.144665560773,0.));
#60964=CARTESIAN_POINT('Ctrl Pts',(148.435583321827,44.144665560773,44.144665560773));
#60965=CARTESIAN_POINT('Ctrl Pts',(148.435583321827,0.,44.144665560773));
#60966=CARTESIAN_POINT('Ctrl Pts',(148.435583321827,-44.144665560773,44.144665560773));
#60967=CARTESIAN_POINT('Ctrl Pts',(148.435583321827,-44.144665560773,0.));
#60968=CARTESIAN_POINT('Ctrl Pts',(148.435583321827,-44.144665560773,-44.144665560773));
#60969=CARTESIAN_POINT('Ctrl Pts',(148.435583321827,0.,-44.144665560773));
#60970=CARTESIAN_POINT('Ctrl Pts',(148.435583321827,44.144665560773,-44.144665560773));
#60971=CARTESIAN_POINT('Ctrl Pts',(148.435583321827,44.144665560773,0.));
#60972=CARTESIAN_POINT('Ctrl Pts',(147.954251119396,44.4430082967122,0.));
#60973=CARTESIAN_POINT('Ctrl Pts',(147.954251119396,44.4430082967121,44.4430082967121));
#60974=CARTESIAN_POINT('Ctrl Pts',(147.954251119396,0.,44.4430082967122));
#60975=CARTESIAN_POINT('Ctrl Pts',(147.954251119396,-44.4430082967121,44.4430082967121));
#60976=CARTESIAN_POINT('Ctrl Pts',(147.954251119396,-44.4430082967122,0.));
#60977=CARTESIAN_POINT('Ctrl Pts',(147.954251119396,-44.4430082967121,-44.4430082967121));
#60978=CARTESIAN_POINT('Ctrl Pts',(147.954251119396,0.,-44.4430082967122));
#60979=CARTESIAN_POINT('Ctrl Pts',(147.954251119396,44.4430082967121,-44.4430082967121));
#60980=CARTESIAN_POINT('Ctrl Pts',(147.954251119396,44.4430082967122,0.));
#60981=CARTESIAN_POINT('Ctrl Pts',(147.433726231016,44.6923434026522,0.));
#60982=CARTESIAN_POINT('Ctrl Pts',(147.433726231016,44.6923434026522,44.6923434026522));
#60983=CARTESIAN_POINT('Ctrl Pts',(147.433726231016,0.,44.6923434026522));
#60984=CARTESIAN_POINT('Ctrl Pts',(147.433726231016,-44.6923434026522,44.6923434026522));
#60985=CARTESIAN_POINT('Ctrl Pts',(147.433726231016,-44.6923434026522,0.));
#60986=CARTESIAN_POINT('Ctrl Pts',(147.433726231016,-44.6923434026522,-44.6923434026522));
#60987=CARTESIAN_POINT('Ctrl Pts',(147.433726231016,0.,-44.6923434026522));
#60988=CARTESIAN_POINT('Ctrl Pts',(147.433726231016,44.6923434026522,-44.6923434026522));
#60989=CARTESIAN_POINT('Ctrl Pts',(147.433726231016,44.6923434026522,0.));
#60990=CARTESIAN_POINT('Ctrl Pts',(146.875905699336,44.8950429937247,0.));
#60991=CARTESIAN_POINT('Ctrl Pts',(146.875905699336,44.8950429937247,44.8950429937247));
#60992=CARTESIAN_POINT('Ctrl Pts',(146.875905699336,0.,44.8950429937247));
#60993=CARTESIAN_POINT('Ctrl Pts',(146.875905699336,-44.8950429937247,44.8950429937247));
#60994=CARTESIAN_POINT('Ctrl Pts',(146.875905699336,-44.8950429937247,0.));
#60995=CARTESIAN_POINT('Ctrl Pts',(146.875905699336,-44.8950429937247,-44.8950429937247));
#60996=CARTESIAN_POINT('Ctrl Pts',(146.875905699336,0.,-44.8950429937247));
#60997=CARTESIAN_POINT('Ctrl Pts',(146.875905699336,44.8950429937247,-44.8950429937247));
#60998=CARTESIAN_POINT('Ctrl Pts',(146.875905699336,44.8950429937247,0.));
#60999=CARTESIAN_POINT('Ctrl Pts',(146.283750613341,45.0548096983452,0.));
#61000=CARTESIAN_POINT('Ctrl Pts',(146.283750613341,45.0548096983452,45.0548096983452));
#61001=CARTESIAN_POINT('Ctrl Pts',(146.283750613341,0.,45.0548096983452));
#61002=CARTESIAN_POINT('Ctrl Pts',(146.283750613341,-45.0548096983452,45.0548096983452));
#61003=CARTESIAN_POINT('Ctrl Pts',(146.283750613341,-45.0548096983452,0.));
#61004=CARTESIAN_POINT('Ctrl Pts',(146.283750613341,-45.0548096983452,-45.0548096983452));
#61005=CARTESIAN_POINT('Ctrl Pts',(146.283750613341,0.,-45.0548096983452));
#61006=CARTESIAN_POINT('Ctrl Pts',(146.283750613341,45.0548096983452,-45.0548096983452));
#61007=CARTESIAN_POINT('Ctrl Pts',(146.283750613341,45.0548096983452,0.));
#61008=CARTESIAN_POINT('Ctrl Pts',(145.784885333877,45.1511857894411,0.));
#61009=CARTESIAN_POINT('Ctrl Pts',(145.784885333877,45.151185789441,45.151185789441));
#61010=CARTESIAN_POINT('Ctrl Pts',(145.784885333877,0.,45.1511857894411));
#61011=CARTESIAN_POINT('Ctrl Pts',(145.784885333877,-45.151185789441,45.151185789441));
#61012=CARTESIAN_POINT('Ctrl Pts',(145.784885333877,-45.1511857894411,0.));
#61013=CARTESIAN_POINT('Ctrl Pts',(145.784885333877,-45.151185789441,-45.151185789441));
#61014=CARTESIAN_POINT('Ctrl Pts',(145.784885333877,0.,-45.1511857894411));
#61015=CARTESIAN_POINT('Ctrl Pts',(145.784885333877,45.151185789441,-45.151185789441));
#61016=CARTESIAN_POINT('Ctrl Pts',(145.784885333877,45.1511857894411,0.));
#61017=CARTESIAN_POINT('Ctrl Pts',(145.397504244566,45.2069220328789,0.));
#61018=CARTESIAN_POINT('Ctrl Pts',(145.397504244566,45.2069220328789,45.2069220328789));
#61019=CARTESIAN_POINT('Ctrl Pts',(145.397504244566,0.,45.2069220328789));
#61020=CARTESIAN_POINT('Ctrl Pts',(145.397504244566,-45.2069220328789,45.2069220328789));
#61021=CARTESIAN_POINT('Ctrl Pts',(145.397504244566,-45.2069220328789,0.));
#61022=CARTESIAN_POINT('Ctrl Pts',(145.397504244566,-45.2069220328789,-45.2069220328789));
#61023=CARTESIAN_POINT('Ctrl Pts',(145.397504244566,0.,-45.2069220328789));
#61024=CARTESIAN_POINT('Ctrl Pts',(145.397504244566,45.2069220328789,-45.2069220328789));
#61025=CARTESIAN_POINT('Ctrl Pts',(145.397504244566,45.2069220328789,0.));
#61026=CARTESIAN_POINT('Ctrl Pts',(145.13346556309,45.2368462755315,0.));
#61027=CARTESIAN_POINT('Ctrl Pts',(145.13346556309,45.2368462755315,45.2368462755315));
#61028=CARTESIAN_POINT('Ctrl Pts',(145.13346556309,0.,45.2368462755315));
#61029=CARTESIAN_POINT('Ctrl Pts',(145.13346556309,-45.2368462755315,45.2368462755315));
#61030=CARTESIAN_POINT('Ctrl Pts',(145.13346556309,-45.2368462755315,0.));
#61031=CARTESIAN_POINT('Ctrl Pts',(145.13346556309,-45.2368462755315,-45.2368462755315));
#61032=CARTESIAN_POINT('Ctrl Pts',(145.13346556309,0.,-45.2368462755315));
#61033=CARTESIAN_POINT('Ctrl Pts',(145.13346556309,45.2368462755315,-45.2368462755315));
#61034=CARTESIAN_POINT('Ctrl Pts',(145.13346556309,45.2368462755315,0.));
#61035=CARTESIAN_POINT('Ctrl Pts',(145.,45.25,0.));
#61036=CARTESIAN_POINT('Ctrl Pts',(145.,45.25,45.25));
#61037=CARTESIAN_POINT('Ctrl Pts',(145.,0.,45.25));
#61038=CARTESIAN_POINT('Ctrl Pts',(145.,-45.25,45.25));
#61039=CARTESIAN_POINT('Ctrl Pts',(145.,-45.25,0.));
#61040=CARTESIAN_POINT('Ctrl Pts',(145.,-45.25,-45.25));
#61041=CARTESIAN_POINT('Ctrl Pts',(145.,0.,-45.25));
#61042=CARTESIAN_POINT('Ctrl Pts',(145.,45.25,-45.25));
#61043=CARTESIAN_POINT('Ctrl Pts',(145.,45.25,0.));
#61044=CARTESIAN_POINT('',(145.052346201785,45.2447205552935,1.02695629777827E-14));
#61045=CARTESIAN_POINT('Ctrl Pts',(145.052346201785,45.2447205552935,0.));
#61046=CARTESIAN_POINT('Ctrl Pts',(145.174905813468,45.2320766440608,0.));
#61047=CARTESIAN_POINT('Ctrl Pts',(145.427915588065,45.2025084676856,0.));
#61048=CARTESIAN_POINT('Ctrl Pts',(145.804474881143,45.147387267467,0.));
#61049=CARTESIAN_POINT('Ctrl Pts',(146.29305636807,45.0522989544503,0.));
#61050=CARTESIAN_POINT('Ctrl Pts',(146.875905699336,44.8950429937247,0.));
#61051=CARTESIAN_POINT('Ctrl Pts',(147.433726231016,44.6923434026522,0.));
#61052=CARTESIAN_POINT('Ctrl Pts',(147.954251119396,44.4430082967122,0.));
#61053=CARTESIAN_POINT('Ctrl Pts',(148.435583321827,44.144665560773,0.));
#61054=CARTESIAN_POINT('Ctrl Pts',(148.878896254171,43.7987824668423,0.));
#61055=CARTESIAN_POINT('Ctrl Pts',(149.23898720348,43.4545599506045,0.));
#61056=CARTESIAN_POINT('Ctrl Pts',(149.498546133041,43.1646721820276,0.));
#61057=CARTESIAN_POINT('Ctrl Pts',(149.673066024454,42.948492018341,0.));
#61058=CARTESIAN_POINT('Ctrl Pts',(149.772227121177,42.8181239065276,0.));
#61059=CARTESIAN_POINT('Ctrl Pts',(149.800942407062,42.7797111789148,0.));
#61060=CARTESIAN_POINT('Ctrl Pts',(145.052346201785,45.2447205552935,2.22005293331856E-14));
#61061=CARTESIAN_POINT('Ctrl Pts',(145.052346201785,45.2447205552935,-6.76829188978049));
#61062=CARTESIAN_POINT('Ctrl Pts',(145.052346201785,43.7025428909119,-13.5356220341073));
#61063=CARTESIAN_POINT('Ctrl Pts',(145.052346201785,40.766566870602,-19.6317498036206));
#61064=CARTESIAN_POINT('Ctrl Pts',(145.052346201785,37.8305908502921,-25.7278775731339));
#61065=CARTESIAN_POINT('Ctrl Pts',(145.052346201785,33.5008164740539,-31.1528029678338));
#61066=CARTESIAN_POINT('Ctrl Pts',(145.052346201785,28.2108765407992,-35.3745247878701));
#61067=CARTESIAN_POINT('Ctrl Pts',(145.052346201785,24.6842499186295,-38.1890060012277));
#61068=CARTESIAN_POINT('Ctrl Pts',(145.052346201785,20.7308830488968,-40.4687300702904));
#61069=CARTESIAN_POINT('Ctrl Pts',(145.052346201785,16.5302272146236,-42.1168092796416));
#61070=CARTESIAN_POINT('Ctrl Pts',(145.052346201785,12.3295713803504,-43.7648884889929));
#61071=CARTESIAN_POINT('Ctrl Pts',(145.052346201785,7.88162658153661,-44.7813228386328));
#61072=CARTESIAN_POINT('Ctrl Pts',(145.052346201785,3.38209886913992,-45.1190318016268));
#61073=CARTESIAN_POINT('Ctrl Pts',(145.052346201785,1.13233501294157,-45.2878862831238));
#61074=CARTESIAN_POINT('Ctrl Pts',(145.052346201785,-1.13032457165251,-45.2870594179593));
#61075=CARTESIAN_POINT('Ctrl Pts',(145.052346201785,-3.38031805124389,-45.1183542446882));
#61076=CARTESIAN_POINT('Ctrl Pts',(145.052346201785,-5.63031153083528,-44.9496490714171));
#61077=CARTESIAN_POINT('Ctrl Pts',(145.052346201785,-7.86763890542398,-44.6130655900395));
#61078=CARTESIAN_POINT('Ctrl Pts',(145.052346201785,-10.0671664521223,-44.1108615201447));
#61079=CARTESIAN_POINT('Ctrl Pts',(145.052346201785,-14.4662215455191,-43.1064533803549));
#61080=CARTESIAN_POINT('Ctrl Pts',(145.052346201785,-18.7140773273544,-41.4395628864962));
#61081=CARTESIAN_POINT('Ctrl Pts',(145.052346201785,-22.6218925892863,-39.1836030048322));
#61082=CARTESIAN_POINT('Ctrl Pts',(145.052346201785,-26.5297078512182,-36.9276431231683));
#61083=CARTESIAN_POINT('Ctrl Pts',(145.052346201785,-30.0974825932466,-34.0826138536992));
#61084=CARTESIAN_POINT('Ctrl Pts',(145.052346201785,-33.1668138343388,-30.7750429976082));
#61085=CARTESIAN_POINT('Ctrl Pts',(145.052346201785,-36.236145075431,-27.4674721415172));
#61086=CARTESIAN_POINT('Ctrl Pts',(145.052346201785,-38.8070328155871,-23.6973596988043));
#61087=CARTESIAN_POINT('Ctrl Pts',(145.052346201785,-40.7647434819831,-19.6319380731881));
#61088=CARTESIAN_POINT('Ctrl Pts',(145.052346201785,-42.7224541483791,-15.5665164475719));
#61089=CARTESIAN_POINT('Ctrl Pts',(145.052346201785,-44.0669877410151,-11.2057856390525));
#61090=CARTESIAN_POINT('Ctrl Pts',(145.052346201785,-44.7395187366316,-6.74386240496236));
#61091=CARTESIAN_POINT('Ctrl Pts',(145.052346201785,-45.4120497322481,-2.28193917087223));
#61092=CARTESIAN_POINT('Ctrl Pts',(145.052346201785,-45.4125781308451,2.28117648878862));
#61093=CARTESIAN_POINT('Ctrl Pts',(145.052346201785,-44.7401784091482,6.7429968860534));
#61094=CARTESIAN_POINT('Ctrl Pts',(145.052346201785,-44.0677786874512,11.2048172833182));
#61095=CARTESIAN_POINT('Ctrl Pts',(145.052346201785,-42.7224508454602,15.565342418187));
#61096=CARTESIAN_POINT('Ctrl Pts',(145.052346201785,-40.7645356928476,19.6307299209617));
#61097=CARTESIAN_POINT('Ctrl Pts',(145.052346201785,-38.806620540235,23.6961174237364));
#61098=CARTESIAN_POINT('Ctrl Pts',(145.052346201785,-36.2361180770008,27.4663672944172));
#61099=CARTESIAN_POINT('Ctrl Pts',(145.052346201785,-33.1671049059906,30.7741206679022));
#61100=CARTESIAN_POINT('Ctrl Pts',(145.052346201785,-30.0980917349805,34.0818740413872));
#61101=CARTESIAN_POINT('Ctrl Pts',(145.052346201785,-26.5305678561944,36.9271309176765));
#61102=CARTESIAN_POINT('Ctrl Pts',(145.052346201785,-22.6229601830524,39.1834368258006));
#61103=CARTESIAN_POINT('Ctrl Pts',(145.052346201785,-18.7153525099103,41.4397427339247));
#61104=CARTESIAN_POINT('Ctrl Pts',(145.052346201785,-14.4676610424124,43.1070976738836));
#61105=CARTESIAN_POINT('Ctrl Pts',(145.052346201785,-10.0684701752482,44.111150221036));
#61106=CARTESIAN_POINT('Ctrl Pts',(145.052346201785,-5.66927930808405,45.1152027681884));
#61107=CARTESIAN_POINT('Ctrl Pts',(145.052346201785,-1.11858904125367,45.4559529225344));
#61108=CARTESIAN_POINT('Ctrl Pts',(145.052346201785,3.38092641212812,45.1185504117569));
#61109=CARTESIAN_POINT('Ctrl Pts',(145.052346201785,7.88044186550994,44.7811479009795));
#61110=CARTESIAN_POINT('Ctrl Pts',(145.052346201785,12.3287825054432,43.7655927250787));
#61111=CARTESIAN_POINT('Ctrl Pts',(145.052346201785,16.5296206098188,42.1177659511616));
#61112=CARTESIAN_POINT('Ctrl Pts',(145.052346201785,20.7304587141944,40.4699391772446));
#61113=CARTESIAN_POINT('Ctrl Pts',(145.052346201785,24.6837942830125,38.1898408053112));
#61114=CARTESIAN_POINT('Ctrl Pts',(145.052346201785,28.2104075661917,35.3752621818815));
#61115=CARTESIAN_POINT('Ctrl Pts',(145.052346201785,33.5003274909606,31.153394246737));
#61116=CARTESIAN_POINT('Ctrl Pts',(145.052346201785,37.8301222730421,25.7289457457255));
#61117=CARTESIAN_POINT('Ctrl Pts',(145.052346201785,40.7662205391253,19.6326701564864));
#61118=CARTESIAN_POINT('Ctrl Pts',(145.052346201785,43.7023188052085,13.5363945672473));
#61119=CARTESIAN_POINT('Ctrl Pts',(145.052346201785,45.2447205552935,6.76829188978051));
#61120=CARTESIAN_POINT('Ctrl Pts',(145.052346201785,45.2447205552935,9.95224728270563E-18));
#61121=CARTESIAN_POINT('Origin',(150.,40.,0.));
#61122=CARTESIAN_POINT('',(150.,-40.,-4.89858719658941E-15));
#61123=CARTESIAN_POINT('Origin',(150.,0.,0.));
#61124=CARTESIAN_POINT('Ctrl Pts',(144.949725458869,45.25,0.));
#61125=CARTESIAN_POINT('Ctrl Pts',(144.949725458869,45.25,6.7690816575667));
#61126=CARTESIAN_POINT('Ctrl Pts',(144.949725458869,42.1648365451369,20.3068665039156));
#61127=CARTESIAN_POINT('Ctrl Pts',(144.949725458869,30.6173698508514,34.773750398626));
#61128=CARTESIAN_POINT('Ctrl Pts',(144.949725458869,16.7790808079035,42.7550258982421));
#61129=CARTESIAN_POINT('Ctrl Pts',(144.949725458869,3.43250170520011,45.8020469304542));
#61130=CARTESIAN_POINT('Ctrl Pts',(144.949725458869,-10.2211621066311,44.7796771846639));
#61131=CARTESIAN_POINT('Ctrl Pts',(144.949725458869,-22.9657234529246,39.7770286917242));
#61132=CARTESIAN_POINT('Ctrl Pts',(144.949725458869,-33.669543934109,31.2402620542942));
#61133=CARTESIAN_POINT('Ctrl Pts',(144.949725458869,-41.3819511520428,19.928192631312));
#61134=CARTESIAN_POINT('Ctrl Pts',(144.949725458869,-45.4184056225061,6.84509078443417));
#61135=CARTESIAN_POINT('Ctrl Pts',(144.949725458869,-45.4168202417441,-6.84585355551244));
#61136=CARTESIAN_POINT('Ctrl Pts',(144.949725458869,-41.3827487973803,-19.9295724953403));
#61137=CARTESIAN_POINT('Ctrl Pts',(144.949725458869,-33.6691856138111,-31.2412295863112));
#61138=CARTESIAN_POINT('Ctrl Pts',(144.949725458869,-22.964612455083,-39.7773133236046));
#61139=CARTESIAN_POINT('Ctrl Pts',(144.949725458869,-12.3437338327282,-43.9450258169844));
#61140=CARTESIAN_POINT('Ctrl Pts',(144.949725458869,-3.39338007143899,-45.2915168413879));
#61141=CARTESIAN_POINT('Ctrl Pts',(144.949725458869,5.65831435357198,-45.2948246879816));
#61142=CARTESIAN_POINT('Ctrl Pts',(144.949725458869,16.7794738875531,-42.7534423036548));
#61143=CARTESIAN_POINT('Ctrl Pts',(144.949725458869,30.6178724964854,-34.7734770169522));
#61144=CARTESIAN_POINT('Ctrl Pts',(144.949725458869,42.165284768839,-20.3053212573473));
#61145=CARTESIAN_POINT('Ctrl Pts',(144.949725458869,45.25,-6.76908165756668));
#61146=CARTESIAN_POINT('Ctrl Pts',(144.949725458869,45.25,2.16493489801906E-14));
#61147=CARTESIAN_POINT('Ctrl Pts',(144.983992698424,45.25,-5.91199053597181E-19));
#61148=CARTESIAN_POINT('Ctrl Pts',(144.983992698424,45.25,6.76908170730493));
#61149=CARTESIAN_POINT('Ctrl Pts',(144.983992698424,42.1648365693141,20.3068664930911));
#61150=CARTESIAN_POINT('Ctrl Pts',(144.983992698424,30.617369871655,34.7737504108949));
#61151=CARTESIAN_POINT('Ctrl Pts',(144.983992698424,16.7790808420695,42.7550259094975));
#61152=CARTESIAN_POINT('Ctrl Pts',(144.983992698424,3.43250170511537,45.8020469445006));
#61153=CARTESIAN_POINT('Ctrl Pts',(144.983992698424,-10.2211621158898,44.7796772061424));
#61154=CARTESIAN_POINT('Ctrl Pts',(144.983992698424,-22.9657234551507,39.7770287101634));
#61155=CARTESIAN_POINT('Ctrl Pts',(144.983992698424,-33.6695439624845,31.2402620570481));
#61156=CARTESIAN_POINT('Ctrl Pts',(144.983992698424,-41.3819511714999,19.9281926323005));
#61157=CARTESIAN_POINT('Ctrl Pts',(144.983992698424,-45.4184056447783,6.84509081325278));
#61158=CARTESIAN_POINT('Ctrl Pts',(144.983992698424,-45.4168202558775,-6.84585355997736));
#61159=CARTESIAN_POINT('Ctrl Pts',(144.983992698424,-41.3827488152505,-19.9295725093942));
#61160=CARTESIAN_POINT('Ctrl Pts',(144.983992698424,-33.6691856378096,-31.2412295916867));
#61161=CARTESIAN_POINT('Ctrl Pts',(144.983992698424,-22.9646124434915,-39.7773133514703));
#61162=CARTESIAN_POINT('Ctrl Pts',(144.983992698424,-12.3437338632281,-43.9450258307769));
#61163=CARTESIAN_POINT('Ctrl Pts',(144.983992698424,-3.39338007314566,-45.2915168578961));
#61164=CARTESIAN_POINT('Ctrl Pts',(144.983992698424,5.65831436041522,-45.2948247082715));
#61165=CARTESIAN_POINT('Ctrl Pts',(144.983992698424,16.779473895429,-42.7534423129232));
#61166=CARTESIAN_POINT('Ctrl Pts',(144.983992698424,30.6178725490117,-34.773477016942));
#61167=CARTESIAN_POINT('Ctrl Pts',(144.983992698424,42.165284776593,-20.3053212511383));
#61168=CARTESIAN_POINT('Ctrl Pts',(144.983992698424,45.25,-6.76908170730491));
#61169=CARTESIAN_POINT('Ctrl Pts',(144.983992698424,45.25,2.164903013931E-14));
#61170=CARTESIAN_POINT('Ctrl Pts',(145.018259874226,45.2482370848744,2.73206091863161E-18));
#61171=CARTESIAN_POINT('Ctrl Pts',(145.018259874226,45.2482370848744,6.76881798756309));
#61172=CARTESIAN_POINT('Ctrl Pts',(145.018259874226,42.1631938504406,20.306075348744));
#61173=CARTESIAN_POINT('Ctrl Pts',(145.018259874226,30.6161770357389,34.7723956446846));
#61174=CARTESIAN_POINT('Ctrl Pts',(145.018259874226,16.7784271382763,42.753360197182));
#61175=CARTESIAN_POINT('Ctrl Pts',(145.018259874226,3.4323679767359,45.8002625219183));
#61176=CARTESIAN_POINT('Ctrl Pts',(145.018259874226,-10.2207639050251,44.7779326145172));
#61177=CARTESIAN_POINT('Ctrl Pts',(145.018259874226,-22.9648287231876,39.775479018976));
#61178=CARTESIAN_POINT('Ctrl Pts',(145.018259874226,-33.6682322155377,31.2390449536092));
#61179=CARTESIAN_POINT('Ctrl Pts',(145.018259874226,-41.3803389534149,19.9274162408695));
#61180=CARTESIAN_POINT('Ctrl Pts',(145.018259874226,-45.4166361686436,6.8448241322546));
#61181=CARTESIAN_POINT('Ctrl Pts',(145.018259874226,-45.4150508415151,-6.84558684928235));
#61182=CARTESIAN_POINT('Ctrl Pts',(145.018259874226,-41.3811365660909,-19.9287960641935));
#61183=CARTESIAN_POINT('Ctrl Pts',(145.018259874225,-33.6678739048263,-31.2400124505512));
#61184=CARTESIAN_POINT('Ctrl Pts',(145.018259874226,-22.9637177548238,-39.7757636491859));
#61185=CARTESIAN_POINT('Ctrl Pts',(145.018259874226,-12.343252958118,-43.9433137567165));
#61186=CARTESIAN_POINT('Ctrl Pts',(145.018259874226,-3.39324786892202,-45.2897523252833));
#61187=CARTESIAN_POINT('Ctrl Pts',(145.018259874226,5.65809391559272,-45.2930600467837));
#61188=CARTESIAN_POINT('Ctrl Pts',(145.018259874226,16.7788201763436,-42.7517766623053));
#61189=CARTESIAN_POINT('Ctrl Pts',(145.018259874226,30.6166796934864,-34.7721222613928));
#61190=CARTESIAN_POINT('Ctrl Pts',(145.018259874226,42.1636420402706,-20.3045301669893));
#61191=CARTESIAN_POINT('Ctrl Pts',(145.018259874225,45.2482370848744,-6.76881798756306));
#61192=CARTESIAN_POINT('Ctrl Pts',(145.018259874225,45.2482370848744,2.16477326845411E-14));
#61193=CARTESIAN_POINT('Ctrl Pts',(145.052346201785,45.2447205552935,9.95224728270563E-18));
#61194=CARTESIAN_POINT('Ctrl Pts',(145.052346201785,45.2447205552935,6.76829188978051));
#61195=CARTESIAN_POINT('Ctrl Pts',(145.052346201785,42.1599170551236,20.304497244714));
#61196=CARTESIAN_POINT('Ctrl Pts',(145.052346201785,30.6137976362395,34.7696932474113));
#61197=CARTESIAN_POINT('Ctrl Pts',(145.052346201785,16.7771231453764,42.7500375491779));
#61198=CARTESIAN_POINT('Ctrl Pts',(145.052346201785,3.43210122557674,45.7967030768803));
#61199=CARTESIAN_POINT('Ctrl Pts',(145.052346201785,-10.2199695749144,44.7744526138424));
#61200=CARTESIAN_POINT('Ctrl Pts',(145.052346201785,-22.9630439774083,39.7723877939658));
#61201=CARTESIAN_POINT('Ctrl Pts',(145.052346201785,-33.6656156137666,31.2366171650979));
#61202=CARTESIAN_POINT('Ctrl Pts',(145.052346201785,-41.3771230034692,19.9258675530557));
#61203=CARTESIAN_POINT('Ctrl Pts',(145.052346201785,-45.4131065294422,6.84429214844948));
#61204=CARTESIAN_POINT('Ctrl Pts',(145.052346201785,-45.4115213336511,-6.84505483053309));
#61205=CARTESIAN_POINT('Ctrl Pts',(145.052346201785,-41.3779205557432,-19.9272472560913));
#61206=CARTESIAN_POINT('Ctrl Pts',(145.052346201785,-33.665257335275,-31.2375845842302));
#61207=CARTESIAN_POINT('Ctrl Pts',(145.052346201785,-22.9619331091898,-39.7726723926374));
#61208=CARTESIAN_POINT('Ctrl Pts',(145.052346201785,-12.3422936546013,-43.9398986272843));
#61209=CARTESIAN_POINT('Ctrl Pts',(145.052346201785,-3.3929841562466,-45.2862325527948));
#61210=CARTESIAN_POINT('Ctrl Pts',(145.052346201785,5.65765418212972,-45.2895400134528));
#61211=CARTESIAN_POINT('Ctrl Pts',(145.052346201785,16.7775161791643,-42.748454139353));
#61212=CARTESIAN_POINT('Ctrl Pts',(145.052346201785,30.6143002232285,-34.7694198976337));
#61213=CARTESIAN_POINT('Ctrl Pts',(145.052346201785,42.1603652265302,-20.302952178434));
#61214=CARTESIAN_POINT('Ctrl Pts',(145.052346201785,45.2447205552935,-6.76829188978049));
#61215=CARTESIAN_POINT('Ctrl Pts',(145.052346201785,45.2447205552935,2.16454634609096E-14));
#61216=CARTESIAN_POINT('',(144.949725458869,45.25,0.));
#61217=CARTESIAN_POINT('Origin',(144.949725458869,44.25,2.22044604925031E-15));
#61218=CARTESIAN_POINT('',(144.949725458869,-45.2494769985824,-2.1306127088172E-5));
#61219=CARTESIAN_POINT('Ctrl Pts',(144.949725458869,45.25,0.));
#61220=CARTESIAN_POINT('Ctrl Pts',(144.949725458869,45.25,6.7690816575667));
#61221=CARTESIAN_POINT('Ctrl Pts',(144.949725458869,42.1648365451369,20.3068665039156));
#61222=CARTESIAN_POINT('Ctrl Pts',(144.949725458869,30.6173698508514,34.773750398626));
#61223=CARTESIAN_POINT('Ctrl Pts',(144.949725458869,16.7790808079035,42.7550258982421));
#61224=CARTESIAN_POINT('Ctrl Pts',(144.949725458869,3.43250170520011,45.8020469304542));
#61225=CARTESIAN_POINT('Ctrl Pts',(144.949725458869,-10.2211621066311,44.7796771846639));
#61226=CARTESIAN_POINT('Ctrl Pts',(144.949725458869,-22.9657234529246,39.7770286917242));
#61227=CARTESIAN_POINT('Ctrl Pts',(144.949725458869,-33.669543934109,31.2402620542942));
#61228=CARTESIAN_POINT('Ctrl Pts',(144.949725458869,-41.3819511520428,19.928192631312));
#61229=CARTESIAN_POINT('Ctrl Pts',(144.949725458869,-44.7456261491756,9.02572788426523));
#61230=CARTESIAN_POINT('Ctrl Pts',(144.949725458869,-45.2496069923152,2.2563645227576));
#61231=CARTESIAN_POINT('Ctrl Pts',(144.949725458869,-45.2494769985824,-2.13061270880333E-5));
#61232=CARTESIAN_POINT('Ctrl Pts',(144.949725458869,-45.2494769985824,-2.13061270880333E-5));
#61233=CARTESIAN_POINT('Ctrl Pts',(144.949725458869,-45.249346990526,-2.25665575868847));
#61234=CARTESIAN_POINT('Ctrl Pts',(144.949725458869,-44.7445120407232,-9.02635324779967));
#61235=CARTESIAN_POINT('Ctrl Pts',(144.949725458869,-41.3827487973803,-19.9295724953403));
#61236=CARTESIAN_POINT('Ctrl Pts',(144.949725458869,-33.6691856138111,-31.2412295863112));
#61237=CARTESIAN_POINT('Ctrl Pts',(144.949725458869,-22.964612455083,-39.7773133236046));
#61238=CARTESIAN_POINT('Ctrl Pts',(144.949725458869,-12.3437338327282,-43.9450258169844));
#61239=CARTESIAN_POINT('Ctrl Pts',(144.949725458869,-3.39338007143899,-45.2915168413879));
#61240=CARTESIAN_POINT('Ctrl Pts',(144.949725458869,5.65831435357198,-45.2948246879816));
#61241=CARTESIAN_POINT('Ctrl Pts',(144.949725458869,16.7794738875531,-42.7534423036548));
#61242=CARTESIAN_POINT('Ctrl Pts',(144.949725458869,30.6178724964854,-34.7734770169522));
#61243=CARTESIAN_POINT('Ctrl Pts',(144.949725458869,42.165284768839,-20.3053212573473));
#61244=CARTESIAN_POINT('Ctrl Pts',(144.949725458869,45.25,-6.76908165756668));
#61245=CARTESIAN_POINT('Ctrl Pts',(144.949725458869,45.25,2.16493489801906E-14));
#61246=CARTESIAN_POINT('Origin',(141.5,0.,0.));
#61247=CARTESIAN_POINT('',(138.148957714707,-45.2494845256127,9.03060215408595E-5));
#61248=CARTESIAN_POINT('',(141.5,-45.25,-5.54152676614177E-15));
#61249=CARTESIAN_POINT('',(138.148957714707,45.25,2.22044604925031E-15));
#61250=CARTESIAN_POINT('Ctrl Pts',(138.148957714707,45.25,2.2264190519331E-15));
#61251=CARTESIAN_POINT('Ctrl Pts',(138.148957714707,45.25,-6.7690816575667));
#61252=CARTESIAN_POINT('Ctrl Pts',(138.148957714707,42.1649342707521,-20.3066141672358));
#61253=CARTESIAN_POINT('Ctrl Pts',(138.148957714707,30.6171004388781,-34.7739601994177));
#61254=CARTESIAN_POINT('Ctrl Pts',(138.148957714707,16.7788181304315,-42.753764956745));
#61255=CARTESIAN_POINT('Ctrl Pts',(138.148957714707,5.65734431171932,-45.2949327941415));
#61256=CARTESIAN_POINT('Ctrl Pts',(138.148957714707,-3.39412279496853,-45.2914545846661));
#61257=CARTESIAN_POINT('Ctrl Pts',(138.148957714707,-12.3447494858218,-43.9447739161242));
#61258=CARTESIAN_POINT('Ctrl Pts',(138.148957714707,-22.9652924680895,-39.7769035859333));
#61259=CARTESIAN_POINT('Ctrl Pts',(138.148957714707,-33.6697810414458,-31.2406023043119));
#61260=CARTESIAN_POINT('Ctrl Pts',(138.148957714707,-41.3831681040918,-19.9287494573035));
#61261=CARTESIAN_POINT('Ctrl Pts',(138.148957714707,-44.744620958737,-9.02566331161857));
#61262=CARTESIAN_POINT('Ctrl Pts',(138.148957714707,-45.2493608977663,-2.25627569231703));
#61263=CARTESIAN_POINT('Ctrl Pts',(138.148957714707,-45.2494845256127,9.03060215429186E-5));
#61264=CARTESIAN_POINT('Ctrl Pts',(138.148957714707,-45.2494845256127,9.03060215429186E-5));
#61265=CARTESIAN_POINT('Ctrl Pts',(138.148957714707,-45.2496081670812,2.25670492585174));
#61266=CARTESIAN_POINT('Ctrl Pts',(138.148957714707,-44.745535934965,9.02625915503247));
#61267=CARTESIAN_POINT('Ctrl Pts',(138.148957714707,-41.3815739483978,19.9289830561684));
#61268=CARTESIAN_POINT('Ctrl Pts',(138.148957714707,-33.6690063462301,31.2408447514654));
#61269=CARTESIAN_POINT('Ctrl Pts',(138.148957714707,-22.9649051952057,39.7775234675741));
#61270=CARTESIAN_POINT('Ctrl Pts',(138.148957714707,-10.2204034199948,44.7798057750713));
#61271=CARTESIAN_POINT('Ctrl Pts',(138.148957714707,3.43335289998614,45.802026673096));
#61272=CARTESIAN_POINT('Ctrl Pts',(138.148957714707,16.7799522682876,42.7546133012331));
#61273=CARTESIAN_POINT('Ctrl Pts',(138.148957714707,30.6179907862887,34.773357927853));
#61274=CARTESIAN_POINT('Ctrl Pts',(138.148957714707,42.1653310999819,20.3055292486728));
#61275=CARTESIAN_POINT('Ctrl Pts',(138.148957714707,45.25,6.76908165756671));
#61276=CARTESIAN_POINT('Ctrl Pts',(138.148957714707,45.25,-4.35425039039354E-17));
#61277=CARTESIAN_POINT('Ctrl Pts',(137.855055085043,45.2058353646297,0.));
#61278=CARTESIAN_POINT('Ctrl Pts',(137.855055085043,45.2058353646297,6.762474938822));
#61279=CARTESIAN_POINT('Ctrl Pts',(137.855055085043,42.1241771447709,20.2857107670094));
#61280=CARTESIAN_POINT('Ctrl Pts',(137.855055085043,30.5881071973639,34.7394186422512));
#61281=CARTESIAN_POINT('Ctrl Pts',(137.855055085043,16.7635747992608,42.7128841983194));
#61282=CARTESIAN_POINT('Ctrl Pts',(137.855055085043,3.4300018993469,45.7573232519416));
#61283=CARTESIAN_POINT('Ctrl Pts',(137.855055085043,-10.2104281627488,44.7361000558667));
#61284=CARTESIAN_POINT('Ctrl Pts',(137.855055085043,-22.9424911252773,39.7387000461403));
#61285=CARTESIAN_POINT('Ctrl Pts',(137.855055085043,-33.6361449232785,31.2103532483248));
#61286=CARTESIAN_POINT('Ctrl Pts',(137.855055085043,-41.3411849511718,19.9095320888761));
#61287=CARTESIAN_POINT('Ctrl Pts',(137.855055085043,-45.3739549727839,6.83917687143108));
#61288=CARTESIAN_POINT('Ctrl Pts',(137.855055085043,-45.3726283874437,-6.83822120345465));
#61289=CARTESIAN_POINT('Ctrl Pts',(137.855055085043,-41.3427775509474,-19.909298718007));
#61290=CARTESIAN_POINT('Ctrl Pts',(137.855055085043,-33.6369188623808,-31.2101110378032));
#61291=CARTESIAN_POINT('Ctrl Pts',(137.855055085043,-22.9428780201773,-39.7380807695128));
#61292=CARTESIAN_POINT('Ctrl Pts',(137.855055085043,-12.332700836987,-43.9018831997389));
#61293=CARTESIAN_POINT('Ctrl Pts',(137.855055085043,-3.39081008346264,-45.247249489039));
#61294=CARTESIAN_POINT('Ctrl Pts',(137.855055085043,5.65182266423444,-45.2507243037332));
#61295=CARTESIAN_POINT('Ctrl Pts',(137.855055085043,16.7624417683392,-42.7120366818274));
#61296=CARTESIAN_POINT('Ctrl Pts',(137.855055085043,30.5872177189448,-34.7400203259904));
#61297=CARTESIAN_POINT('Ctrl Pts',(137.855055085043,42.123780702852,-20.2867946266766));
#61298=CARTESIAN_POINT('Ctrl Pts',(137.855055085043,45.2058353646297,-6.76247493882199));
#61299=CARTESIAN_POINT('Ctrl Pts',(137.855055085043,45.2058353646297,2.22044604925031E-15));
#61300=CARTESIAN_POINT('Ctrl Pts',(137.950099288556,45.2350597921624,1.01520278271097E-17));
#61301=CARTESIAN_POINT('Ctrl Pts',(137.950099288556,45.2350597921624,6.76685018093561));
#61302=CARTESIAN_POINT('Ctrl Pts',(137.950099288556,42.1514110071022,20.2988241759859));
#61303=CARTESIAN_POINT('Ctrl Pts',(137.950099288556,30.6078830357159,34.7618776385385));
#61304=CARTESIAN_POINT('Ctrl Pts',(137.950099288556,16.7744143707633,42.7404977506388));
#61305=CARTESIAN_POINT('Ctrl Pts',(137.950099288556,3.43221929087274,45.7869051502943));
#61306=CARTESIAN_POINT('Ctrl Pts',(137.950099288556,-10.2170295852962,44.7650222726377));
#61307=CARTESIAN_POINT('Ctrl Pts',(137.950099288556,-22.9573229974232,39.7643913625708));
#61308=CARTESIAN_POINT('Ctrl Pts',(137.950099288556,-33.6578917785504,31.2305301259859));
#61309=CARTESIAN_POINT('Ctrl Pts',(137.950099288556,-41.3679122929742,19.9224031471328));
#61310=CARTESIAN_POINT('Ctrl Pts',(137.950099288556,-45.4032895967549,6.843600216278));
#61311=CARTESIAN_POINT('Ctrl Pts',(137.950099288556,-45.4019615910912,-6.84264225249156));
#61312=CARTESIAN_POINT('Ctrl Pts',(137.950099288556,-41.3695058181057,-19.9221705393488));
#61313=CARTESIAN_POINT('Ctrl Pts',(137.950099288556,-33.6586659205302,-31.2302879324169));
#61314=CARTESIAN_POINT('Ctrl Pts',(137.950099288556,-22.9577091861056,-39.7637723365677));
#61315=CARTESIAN_POINT('Ctrl Pts',(137.950099288556,-12.3406757259972,-43.9302655824307));
#61316=CARTESIAN_POINT('Ctrl Pts',(137.950099288556,-3.39300226903125,-45.2765018058852));
#61317=CARTESIAN_POINT('Ctrl Pts',(137.950099288556,5.65547689196804,-45.2799791350405));
#61318=CARTESIAN_POINT('Ctrl Pts',(137.950099288556,16.773278779478,-42.7396495526642));
#61319=CARTESIAN_POINT('Ctrl Pts',(137.950099288556,30.6069951898968,-34.7624788629571));
#61320=CARTESIAN_POINT('Ctrl Pts',(137.950099288556,42.1510131614596,-20.2999090614021));
#61321=CARTESIAN_POINT('Ctrl Pts',(137.950099288556,45.2350597921624,-6.7668501809356));
#61322=CARTESIAN_POINT('Ctrl Pts',(137.950099288556,45.2350597921624,2.22246688854806E-15));
#61323=CARTESIAN_POINT('Ctrl Pts',(138.049521967683,45.25,-4.57772263137747E-18));
#61324=CARTESIAN_POINT('Ctrl Pts',(138.049521967683,45.25,6.7690851555878));
#61325=CARTESIAN_POINT('Ctrl Pts',(138.049521967683,42.1653327604727,20.3055284538557));
#61326=CARTESIAN_POINT('Ctrl Pts',(138.049521967683,30.6179921980673,34.7733587758922));
#61327=CARTESIAN_POINT('Ctrl Pts',(138.049521967683,16.779954629945,42.754614061163));
#61328=CARTESIAN_POINT('Ctrl Pts',(138.049521967683,3.43335288203689,45.8020276276972));
#61329=CARTESIAN_POINT('Ctrl Pts',(138.049521967683,-10.2204040638982,44.7798072466659));
#61330=CARTESIAN_POINT('Ctrl Pts',(138.049521967683,-22.9649053288983,39.7775247298782));
#61331=CARTESIAN_POINT('Ctrl Pts',(138.049521967683,-33.6690082995622,31.2408449275282));
#61332=CARTESIAN_POINT('Ctrl Pts',(138.049521967683,-41.3815752705949,19.9289831065789));
#61333=CARTESIAN_POINT('Ctrl Pts',(138.049521967683,-45.4182853776635,6.8458605298419));
#61334=CARTESIAN_POINT('Ctrl Pts',(138.049521967683,-45.4169569295764,-6.84490223829727));
#61335=CARTESIAN_POINT('Ctrl Pts',(138.049521967683,-41.3831693213291,-19.9287504281582));
#61336=CARTESIAN_POINT('Ctrl Pts',(138.049521967683,-33.669782695211,-31.2406026551428));
#61337=CARTESIAN_POINT('Ctrl Pts',(138.049521967683,-22.965291638655,-39.7769055038315));
#61338=CARTESIAN_POINT('Ctrl Pts',(138.049521967683,-12.344751611106,-43.9447748499145));
#61339=CARTESIAN_POINT('Ctrl Pts',(138.049521967683,-3.39412290850554,-45.2914557087235));
#61340=CARTESIAN_POINT('Ctrl Pts',(138.049521967683,5.65734478257735,-45.2949341881843));
#61341=CARTESIAN_POINT('Ctrl Pts',(138.049521967683,16.7788186512198,-42.7537655821415));
#61342=CARTESIAN_POINT('Ctrl Pts',(138.049521967683,30.6171040739598,-34.7739601931386));
#61343=CARTESIAN_POINT('Ctrl Pts',(138.049521967683,42.1649347756601,-20.3066136997884));
#61344=CARTESIAN_POINT('Ctrl Pts',(138.049521967683,45.25,-6.7690851555878));
#61345=CARTESIAN_POINT('Ctrl Pts',(138.049521967683,45.25,2.22448746226608E-15));
#61346=CARTESIAN_POINT('Ctrl Pts',(138.148957714707,45.25,-4.35425039039354E-17));
#61347=CARTESIAN_POINT('Ctrl Pts',(138.148957714707,45.25,6.76908165756671));
#61348=CARTESIAN_POINT('Ctrl Pts',(138.148957714707,42.1653310999819,20.3055292486728));
#61349=CARTESIAN_POINT('Ctrl Pts',(138.148957714707,30.6179907862887,34.773357927853));
#61350=CARTESIAN_POINT('Ctrl Pts',(138.148957714707,16.7799522682876,42.7546133012331));
#61351=CARTESIAN_POINT('Ctrl Pts',(138.148957714707,3.43335289998614,45.802026673096));
#61352=CARTESIAN_POINT('Ctrl Pts',(138.148957714707,-10.2204034199948,44.7798057750713));
#61353=CARTESIAN_POINT('Ctrl Pts',(138.148957714707,-22.9649051952057,39.7775234675741));
#61354=CARTESIAN_POINT('Ctrl Pts',(138.148957714707,-33.6690063462301,31.2408447514654));
#61355=CARTESIAN_POINT('Ctrl Pts',(138.148957714707,-41.3815739483978,19.9289830561684));
#61356=CARTESIAN_POINT('Ctrl Pts',(138.148957714707,-45.4182838555602,6.84585852547692));
#61357=CARTESIAN_POINT('Ctrl Pts',(138.148957714707,-45.4169559741891,-6.84490192384386));
#61358=CARTESIAN_POINT('Ctrl Pts',(138.148957714707,-41.3831681040918,-19.9287494573035));
#61359=CARTESIAN_POINT('Ctrl Pts',(138.148957714707,-33.6697810414458,-31.2406023043119));
#61360=CARTESIAN_POINT('Ctrl Pts',(138.148957714707,-22.9652924680895,-39.7769035859333));
#61361=CARTESIAN_POINT('Ctrl Pts',(138.148957714707,-12.3447494858218,-43.9447739161242));
#61362=CARTESIAN_POINT('Ctrl Pts',(138.148957714707,-3.39412279496853,-45.2914545846661));
#61363=CARTESIAN_POINT('Ctrl Pts',(138.148957714707,5.65734431171932,-45.2949327941415));
#61364=CARTESIAN_POINT('Ctrl Pts',(138.148957714707,16.7788181304315,-42.753764956745));
#61365=CARTESIAN_POINT('Ctrl Pts',(138.148957714707,30.6171004388781,-34.7739601994177));
#61366=CARTESIAN_POINT('Ctrl Pts',(138.148957714707,42.1649342707521,-20.3066141672358));
#61367=CARTESIAN_POINT('Ctrl Pts',(138.148957714707,45.25,-6.7690816575667));
#61368=CARTESIAN_POINT('Ctrl Pts',(138.148957714707,45.25,2.2264190519331E-15));
#61369=CARTESIAN_POINT('',(137.855055085043,45.2058353646297,1.11022302462516E-15));
#61370=CARTESIAN_POINT('Origin',(138.148957714707,44.25,-1.66533453693773E-15));
#61371=CARTESIAN_POINT('Ctrl Pts',(137.855055085043,45.2058353646297,0.));
#61372=CARTESIAN_POINT('Ctrl Pts',(137.855055085043,45.2058353646297,6.762474938822));
#61373=CARTESIAN_POINT('Ctrl Pts',(137.855055085043,42.1241771447709,20.2857107670094));
#61374=CARTESIAN_POINT('Ctrl Pts',(137.855055085043,30.5881071973639,34.7394186422512));
#61375=CARTESIAN_POINT('Ctrl Pts',(137.855055085043,16.7635747992608,42.7128841983194));
#61376=CARTESIAN_POINT('Ctrl Pts',(137.855055085043,3.4300018993469,45.7573232519416));
#61377=CARTESIAN_POINT('Ctrl Pts',(137.855055085043,-10.2104281627488,44.7361000558667));
#61378=CARTESIAN_POINT('Ctrl Pts',(137.855055085043,-22.9424911252773,39.7387000461403));
#61379=CARTESIAN_POINT('Ctrl Pts',(137.855055085043,-33.6361449232785,31.2103532483248));
#61380=CARTESIAN_POINT('Ctrl Pts',(137.855055085043,-41.3411849511718,19.9095320888761));
#61381=CARTESIAN_POINT('Ctrl Pts',(137.855055085043,-45.3739549727839,6.83917687143108));
#61382=CARTESIAN_POINT('Ctrl Pts',(137.855055085043,-45.3726283874437,-6.83822120345465));
#61383=CARTESIAN_POINT('Ctrl Pts',(137.855055085043,-41.3427775509474,-19.909298718007));
#61384=CARTESIAN_POINT('Ctrl Pts',(137.855055085043,-33.6369188623808,-31.2101110378032));
#61385=CARTESIAN_POINT('Ctrl Pts',(137.855055085043,-22.9428780201773,-39.7380807695128));
#61386=CARTESIAN_POINT('Ctrl Pts',(137.855055085043,-12.332700836987,-43.9018831997389));
#61387=CARTESIAN_POINT('Ctrl Pts',(137.855055085043,-3.39081008346264,-45.247249489039));
#61388=CARTESIAN_POINT('Ctrl Pts',(137.855055085043,5.65182266423444,-45.2507243037332));
#61389=CARTESIAN_POINT('Ctrl Pts',(137.855055085043,16.7624417683392,-42.7120366818274));
#61390=CARTESIAN_POINT('Ctrl Pts',(137.855055085043,30.5872177189448,-34.7400203259904));
#61391=CARTESIAN_POINT('Ctrl Pts',(137.855055085043,42.123780702852,-20.2867946266766));
#61392=CARTESIAN_POINT('Ctrl Pts',(137.855055085043,45.2058353646297,-6.76247493882199));
#61393=CARTESIAN_POINT('Ctrl Pts',(137.855055085043,45.2058353646297,2.22044604925031E-15));
#61394=CARTESIAN_POINT('Ctrl Pts',(138.,45.25,0.));
#61395=CARTESIAN_POINT('Ctrl Pts',(138.,45.25,45.25));
#61396=CARTESIAN_POINT('Ctrl Pts',(138.,0.,45.25));
#61397=CARTESIAN_POINT('Ctrl Pts',(138.,-45.25,45.25));
#61398=CARTESIAN_POINT('Ctrl Pts',(138.,-45.25,0.));
#61399=CARTESIAN_POINT('Ctrl Pts',(138.,-45.25,-45.25));
#61400=CARTESIAN_POINT('Ctrl Pts',(138.,0.,-45.25));
#61401=CARTESIAN_POINT('Ctrl Pts',(138.,45.25,-45.25));
#61402=CARTESIAN_POINT('Ctrl Pts',(138.,45.25,0.));
#61403=CARTESIAN_POINT('Ctrl Pts',(137.733721569282,45.1696034559015,0.));
#61404=CARTESIAN_POINT('Ctrl Pts',(137.733721569282,45.1696034559015,45.1696034559015));
#61405=CARTESIAN_POINT('Ctrl Pts',(137.733721569282,0.,45.1696034559015));
#61406=CARTESIAN_POINT('Ctrl Pts',(137.733721569282,-45.1696034559015,45.1696034559015));
#61407=CARTESIAN_POINT('Ctrl Pts',(137.733721569282,-45.1696034559015,0.));
#61408=CARTESIAN_POINT('Ctrl Pts',(137.733721569282,-45.1696034559015,-45.1696034559015));
#61409=CARTESIAN_POINT('Ctrl Pts',(137.733721569282,0.,-45.1696034559015));
#61410=CARTESIAN_POINT('Ctrl Pts',(137.733721569282,45.1696034559015,-45.1696034559015));
#61411=CARTESIAN_POINT('Ctrl Pts',(137.733721569282,45.1696034559015,0.));
#61412=CARTESIAN_POINT('Ctrl Pts',(137.205586355274,45.0033879840311,0.));
#61413=CARTESIAN_POINT('Ctrl Pts',(137.205586355274,45.0033879840311,45.0033879840311));
#61414=CARTESIAN_POINT('Ctrl Pts',(137.205586355274,0.,45.0033879840311));
#61415=CARTESIAN_POINT('Ctrl Pts',(137.205586355274,-45.0033879840311,45.0033879840311));
#61416=CARTESIAN_POINT('Ctrl Pts',(137.205586355274,-45.0033879840311,0.));
#61417=CARTESIAN_POINT('Ctrl Pts',(137.205586355274,-45.0033879840311,-45.0033879840311));
#61418=CARTESIAN_POINT('Ctrl Pts',(137.205586355274,0.,-45.0033879840311));
#61419=CARTESIAN_POINT('Ctrl Pts',(137.205586355274,45.0033879840311,-45.0033879840311));
#61420=CARTESIAN_POINT('Ctrl Pts',(137.205586355274,45.0033879840311,0.));
#61421=CARTESIAN_POINT('Ctrl Pts',(136.426648468102,44.7377976755922,0.));
#61422=CARTESIAN_POINT('Ctrl Pts',(136.426648468102,44.7377976755922,44.7377976755922));
#61423=CARTESIAN_POINT('Ctrl Pts',(136.426648468102,0.,44.7377976755922));
#61424=CARTESIAN_POINT('Ctrl Pts',(136.426648468102,-44.7377976755922,44.7377976755922));
#61425=CARTESIAN_POINT('Ctrl Pts',(136.426648468102,-44.7377976755922,0.));
#61426=CARTESIAN_POINT('Ctrl Pts',(136.426648468102,-44.7377976755922,-44.7377976755922));
#61427=CARTESIAN_POINT('Ctrl Pts',(136.426648468102,0.,-44.7377976755922));
#61428=CARTESIAN_POINT('Ctrl Pts',(136.426648468102,44.7377976755922,-44.7377976755922));
#61429=CARTESIAN_POINT('Ctrl Pts',(136.426648468102,44.7377976755922,0.));
#61430=CARTESIAN_POINT('Ctrl Pts',(135.414787422122,44.350906139381,0.));
#61431=CARTESIAN_POINT('Ctrl Pts',(135.414787422122,44.350906139381,44.350906139381));
#61432=CARTESIAN_POINT('Ctrl Pts',(135.414787422122,0.,44.350906139381));
#61433=CARTESIAN_POINT('Ctrl Pts',(135.414787422122,-44.350906139381,44.350906139381));
#61434=CARTESIAN_POINT('Ctrl Pts',(135.414787422122,-44.350906139381,0.));
#61435=CARTESIAN_POINT('Ctrl Pts',(135.414787422122,-44.350906139381,-44.350906139381));
#61436=CARTESIAN_POINT('Ctrl Pts',(135.414787422122,0.,-44.350906139381));
#61437=CARTESIAN_POINT('Ctrl Pts',(135.414787422122,44.350906139381,-44.350906139381));
#61438=CARTESIAN_POINT('Ctrl Pts',(135.414787422122,44.350906139381,0.));
#61439=CARTESIAN_POINT('Ctrl Pts',(134.195388228683,43.8112254901541,0.));
#61440=CARTESIAN_POINT('Ctrl Pts',(134.195388228683,43.8112254901541,43.8112254901541));
#61441=CARTESIAN_POINT('Ctrl Pts',(134.195388228683,0.,43.8112254901541));
#61442=CARTESIAN_POINT('Ctrl Pts',(134.195388228683,-43.8112254901541,43.8112254901541));
#61443=CARTESIAN_POINT('Ctrl Pts',(134.195388228683,-43.8112254901541,0.));
#61444=CARTESIAN_POINT('Ctrl Pts',(134.195388228683,-43.8112254901541,-43.8112254901541));
#61445=CARTESIAN_POINT('Ctrl Pts',(134.195388228683,0.,-43.8112254901541));
#61446=CARTESIAN_POINT('Ctrl Pts',(134.195388228683,43.8112254901541,-43.8112254901541));
#61447=CARTESIAN_POINT('Ctrl Pts',(134.195388228683,43.8112254901541,0.));
#61448=CARTESIAN_POINT('Ctrl Pts',(133.022036870624,43.2136312541229,0.));
#61449=CARTESIAN_POINT('Ctrl Pts',(133.022036870624,43.2136312541229,43.2136312541229));
#61450=CARTESIAN_POINT('Ctrl Pts',(133.022036870624,0.,43.2136312541229));
#61451=CARTESIAN_POINT('Ctrl Pts',(133.022036870624,-43.2136312541229,43.2136312541229));
#61452=CARTESIAN_POINT('Ctrl Pts',(133.022036870624,-43.2136312541229,0.));
#61453=CARTESIAN_POINT('Ctrl Pts',(133.022036870624,-43.2136312541229,-43.2136312541229));
#61454=CARTESIAN_POINT('Ctrl Pts',(133.022036870624,0.,-43.2136312541229));
#61455=CARTESIAN_POINT('Ctrl Pts',(133.022036870624,43.2136312541229,-43.2136312541229));
#61456=CARTESIAN_POINT('Ctrl Pts',(133.022036870624,43.2136312541229,0.));
#61457=CARTESIAN_POINT('Ctrl Pts',(131.894325225331,42.5564406463359,0.));
#61458=CARTESIAN_POINT('Ctrl Pts',(131.894325225331,42.5564406463358,42.5564406463358));
#61459=CARTESIAN_POINT('Ctrl Pts',(131.894325225331,0.,42.5564406463359));
#61460=CARTESIAN_POINT('Ctrl Pts',(131.894325225331,-42.5564406463358,42.5564406463358));
#61461=CARTESIAN_POINT('Ctrl Pts',(131.894325225331,-42.5564406463359,0.));
#61462=CARTESIAN_POINT('Ctrl Pts',(131.894325225331,-42.5564406463358,-42.5564406463358));
#61463=CARTESIAN_POINT('Ctrl Pts',(131.894325225331,0.,-42.5564406463359));
#61464=CARTESIAN_POINT('Ctrl Pts',(131.894325225331,42.5564406463358,-42.5564406463358));
#61465=CARTESIAN_POINT('Ctrl Pts',(131.894325225331,42.5564406463359,0.));
#61466=CARTESIAN_POINT('Ctrl Pts',(130.809844110982,41.8388975654704,0.));
#61467=CARTESIAN_POINT('Ctrl Pts',(130.809844110982,41.8388975654704,41.8388975654704));
#61468=CARTESIAN_POINT('Ctrl Pts',(130.809844110982,0.,41.8388975654704));
#61469=CARTESIAN_POINT('Ctrl Pts',(130.809844110982,-41.8388975654704,41.8388975654704));
#61470=CARTESIAN_POINT('Ctrl Pts',(130.809844110982,-41.8388975654704,0.));
#61471=CARTESIAN_POINT('Ctrl Pts',(130.809844110982,-41.8388975654704,-41.8388975654704));
#61472=CARTESIAN_POINT('Ctrl Pts',(130.809844110982,0.,-41.8388975654704));
#61473=CARTESIAN_POINT('Ctrl Pts',(130.809844110982,41.8388975654704,-41.8388975654704));
#61474=CARTESIAN_POINT('Ctrl Pts',(130.809844110982,41.8388975654704,0.));
#61475=CARTESIAN_POINT('Ctrl Pts',(129.763264721445,41.0619597887374,0.));
#61476=CARTESIAN_POINT('Ctrl Pts',(129.763264721445,41.0619597887374,41.0619597887374));
#61477=CARTESIAN_POINT('Ctrl Pts',(129.763264721445,0.,41.0619597887374));
#61478=CARTESIAN_POINT('Ctrl Pts',(129.763264721445,-41.0619597887374,41.0619597887374));
#61479=CARTESIAN_POINT('Ctrl Pts',(129.763264721445,-41.0619597887374,0.));
#61480=CARTESIAN_POINT('Ctrl Pts',(129.763264721445,-41.0619597887374,-41.0619597887374));
#61481=CARTESIAN_POINT('Ctrl Pts',(129.763264721445,0.,-41.0619597887374));
#61482=CARTESIAN_POINT('Ctrl Pts',(129.763264721445,41.0619597887374,-41.0619597887374));
#61483=CARTESIAN_POINT('Ctrl Pts',(129.763264721445,41.0619597887374,0.));
#61484=CARTESIAN_POINT('Ctrl Pts',(128.747640262206,40.2275943271253,0.));
#61485=CARTESIAN_POINT('Ctrl Pts',(128.747640262206,40.2275943271253,40.2275943271253));
#61486=CARTESIAN_POINT('Ctrl Pts',(128.747640262206,0.,40.2275943271253));
#61487=CARTESIAN_POINT('Ctrl Pts',(128.747640262206,-40.2275943271253,40.2275943271253));
#61488=CARTESIAN_POINT('Ctrl Pts',(128.747640262206,-40.2275943271253,0.));
#61489=CARTESIAN_POINT('Ctrl Pts',(128.747640262206,-40.2275943271253,-40.2275943271253));
#61490=CARTESIAN_POINT('Ctrl Pts',(128.747640262206,0.,-40.2275943271253));
#61491=CARTESIAN_POINT('Ctrl Pts',(128.747640262206,40.2275943271253,-40.2275943271253));
#61492=CARTESIAN_POINT('Ctrl Pts',(128.747640262206,40.2275943271253,0.));
#61493=CARTESIAN_POINT('Ctrl Pts',(127.755431446906,39.3383655845225,0.));
#61494=CARTESIAN_POINT('Ctrl Pts',(127.755431446906,39.3383655845224,39.3383655845224));
#61495=CARTESIAN_POINT('Ctrl Pts',(127.755431446906,0.,39.3383655845225));
#61496=CARTESIAN_POINT('Ctrl Pts',(127.755431446906,-39.3383655845224,39.3383655845224));
#61497=CARTESIAN_POINT('Ctrl Pts',(127.755431446906,-39.3383655845225,0.));
#61498=CARTESIAN_POINT('Ctrl Pts',(127.755431446906,-39.3383655845224,-39.3383655845224));
#61499=CARTESIAN_POINT('Ctrl Pts',(127.755431446906,0.,-39.3383655845225));
#61500=CARTESIAN_POINT('Ctrl Pts',(127.755431446906,39.3383655845224,-39.3383655845224));
#61501=CARTESIAN_POINT('Ctrl Pts',(127.755431446906,39.3383655845225,0.));
#61502=CARTESIAN_POINT('Ctrl Pts',(126.779460089513,38.3971171615454,0.));
#61503=CARTESIAN_POINT('Ctrl Pts',(126.779460089513,38.3971171615453,38.3971171615453));
#61504=CARTESIAN_POINT('Ctrl Pts',(126.779460089513,0.,38.3971171615454));
#61505=CARTESIAN_POINT('Ctrl Pts',(126.779460089513,-38.3971171615453,38.3971171615453));
#61506=CARTESIAN_POINT('Ctrl Pts',(126.779460089513,-38.3971171615454,0.));
#61507=CARTESIAN_POINT('Ctrl Pts',(126.779460089513,-38.3971171615453,-38.3971171615453));
#61508=CARTESIAN_POINT('Ctrl Pts',(126.779460089513,0.,-38.3971171615454));
#61509=CARTESIAN_POINT('Ctrl Pts',(126.779460089513,38.3971171615453,-38.3971171615453));
#61510=CARTESIAN_POINT('Ctrl Pts',(126.779460089513,38.3971171615454,0.));
#61511=CARTESIAN_POINT('Ctrl Pts',(125.813896300499,37.4068538610988,0.));
#61512=CARTESIAN_POINT('Ctrl Pts',(125.813896300499,37.4068538610988,37.4068538610988));
#61513=CARTESIAN_POINT('Ctrl Pts',(125.813896300499,0.,37.4068538610988));
#61514=CARTESIAN_POINT('Ctrl Pts',(125.813896300499,-37.4068538610988,37.4068538610988));
#61515=CARTESIAN_POINT('Ctrl Pts',(125.813896300499,-37.4068538610988,0.));
#61516=CARTESIAN_POINT('Ctrl Pts',(125.813896300499,-37.4068538610988,-37.4068538610988));
#61517=CARTESIAN_POINT('Ctrl Pts',(125.813896300499,0.,-37.4068538610988));
#61518=CARTESIAN_POINT('Ctrl Pts',(125.813896300499,37.4068538610988,-37.4068538610988));
#61519=CARTESIAN_POINT('Ctrl Pts',(125.813896300499,37.4068538610988,0.));
#61520=CARTESIAN_POINT('Ctrl Pts',(124.854917533862,36.3706304382947,0.));
#61521=CARTESIAN_POINT('Ctrl Pts',(124.854917533862,36.3706304382947,36.3706304382947));
#61522=CARTESIAN_POINT('Ctrl Pts',(124.854917533862,0.,36.3706304382947));
#61523=CARTESIAN_POINT('Ctrl Pts',(124.854917533862,-36.3706304382947,36.3706304382947));
#61524=CARTESIAN_POINT('Ctrl Pts',(124.854917533862,-36.3706304382947,0.));
#61525=CARTESIAN_POINT('Ctrl Pts',(124.854917533862,-36.3706304382947,-36.3706304382947));
#61526=CARTESIAN_POINT('Ctrl Pts',(124.854917533862,0.,-36.3706304382947));
#61527=CARTESIAN_POINT('Ctrl Pts',(124.854917533862,36.3706304382947,-36.3706304382947));
#61528=CARTESIAN_POINT('Ctrl Pts',(124.854917533862,36.3706304382947,0.));
#61529=CARTESIAN_POINT('Ctrl Pts',(123.900175258903,35.2911361038403,0.));
#61530=CARTESIAN_POINT('Ctrl Pts',(123.900175258903,35.2911361038403,35.2911361038403));
#61531=CARTESIAN_POINT('Ctrl Pts',(123.900175258903,0.,35.2911361038403));
#61532=CARTESIAN_POINT('Ctrl Pts',(123.900175258903,-35.2911361038403,35.2911361038403));
#61533=CARTESIAN_POINT('Ctrl Pts',(123.900175258903,-35.2911361038403,0.));
#61534=CARTESIAN_POINT('Ctrl Pts',(123.900175258903,-35.2911361038403,-35.2911361038403));
#61535=CARTESIAN_POINT('Ctrl Pts',(123.900175258903,0.,-35.2911361038403));
#61536=CARTESIAN_POINT('Ctrl Pts',(123.900175258903,35.2911361038403,-35.2911361038403));
#61537=CARTESIAN_POINT('Ctrl Pts',(123.900175258903,35.2911361038403,0.));
#61538=CARTESIAN_POINT('Ctrl Pts',(123.138810144074,34.3945883061935,0.));
#61539=CARTESIAN_POINT('Ctrl Pts',(123.138810144074,34.3945883061935,34.3945883061935));
#61540=CARTESIAN_POINT('Ctrl Pts',(123.138810144074,0.,34.3945883061935));
#61541=CARTESIAN_POINT('Ctrl Pts',(123.138810144074,-34.3945883061935,34.3945883061935));
#61542=CARTESIAN_POINT('Ctrl Pts',(123.138810144074,-34.3945883061935,0.));
#61543=CARTESIAN_POINT('Ctrl Pts',(123.138810144074,-34.3945883061935,-34.3945883061935));
#61544=CARTESIAN_POINT('Ctrl Pts',(123.138810144074,0.,-34.3945883061935));
#61545=CARTESIAN_POINT('Ctrl Pts',(123.138810144074,34.3945883061935,-34.3945883061935));
#61546=CARTESIAN_POINT('Ctrl Pts',(123.138810144074,34.3945883061935,0.));
#61547=CARTESIAN_POINT('Ctrl Pts',(122.568954053309,33.7042250366683,0.));
#61548=CARTESIAN_POINT('Ctrl Pts',(122.568954053309,33.7042250366683,33.7042250366683));
#61549=CARTESIAN_POINT('Ctrl Pts',(122.568954053309,0.,33.7042250366683));
#61550=CARTESIAN_POINT('Ctrl Pts',(122.568954053309,-33.7042250366683,33.7042250366683));
#61551=CARTESIAN_POINT('Ctrl Pts',(122.568954053309,-33.7042250366683,0.));
#61552=CARTESIAN_POINT('Ctrl Pts',(122.568954053309,-33.7042250366683,-33.7042250366683));
#61553=CARTESIAN_POINT('Ctrl Pts',(122.568954053309,0.,-33.7042250366683));
#61554=CARTESIAN_POINT('Ctrl Pts',(122.568954053309,33.7042250366683,-33.7042250366683));
#61555=CARTESIAN_POINT('Ctrl Pts',(122.568954053309,33.7042250366683,0.));
#61556=CARTESIAN_POINT('Ctrl Pts',(122.189565449241,33.2360618564895,0.));
#61557=CARTESIAN_POINT('Ctrl Pts',(122.189565449241,33.2360618564895,33.2360618564895));
#61558=CARTESIAN_POINT('Ctrl Pts',(122.189565449241,0.,33.2360618564895));
#61559=CARTESIAN_POINT('Ctrl Pts',(122.189565449241,-33.2360618564895,33.2360618564895));
#61560=CARTESIAN_POINT('Ctrl Pts',(122.189565449241,-33.2360618564895,0.));
#61561=CARTESIAN_POINT('Ctrl Pts',(122.189565449241,-33.2360618564895,-33.2360618564895));
#61562=CARTESIAN_POINT('Ctrl Pts',(122.189565449241,0.,-33.2360618564895));
#61563=CARTESIAN_POINT('Ctrl Pts',(122.189565449241,33.2360618564895,-33.2360618564895));
#61564=CARTESIAN_POINT('Ctrl Pts',(122.189565449241,33.2360618564895,0.));
#61565=CARTESIAN_POINT('Ctrl Pts',(122.,33.,0.));
#61566=CARTESIAN_POINT('Ctrl Pts',(122.,33.,33.));
#61567=CARTESIAN_POINT('Ctrl Pts',(122.,0.,33.));
#61568=CARTESIAN_POINT('Ctrl Pts',(122.,-33.,33.));
#61569=CARTESIAN_POINT('Ctrl Pts',(122.,-33.,0.));
#61570=CARTESIAN_POINT('Ctrl Pts',(122.,-33.,-33.));
#61571=CARTESIAN_POINT('Ctrl Pts',(122.,0.,-33.));
#61572=CARTESIAN_POINT('Ctrl Pts',(122.,33.,-33.));
#61573=CARTESIAN_POINT('Ctrl Pts',(122.,33.,0.));
#61574=CARTESIAN_POINT('',(122.,33.,0.));
#61575=CARTESIAN_POINT('Ctrl Pts',(122.,33.,0.));
#61576=CARTESIAN_POINT('Ctrl Pts',(122.189565449241,33.2360618564895,0.));
#61577=CARTESIAN_POINT('Ctrl Pts',(122.568954053309,33.7042250366683,0.));
#61578=CARTESIAN_POINT('Ctrl Pts',(123.138810144074,34.3945883061935,0.));
#61579=CARTESIAN_POINT('Ctrl Pts',(123.900175258903,35.2911361038403,0.));
#61580=CARTESIAN_POINT('Ctrl Pts',(124.854917533862,36.3706304382947,0.));
#61581=CARTESIAN_POINT('Ctrl Pts',(125.813896300499,37.4068538610988,0.));
#61582=CARTESIAN_POINT('Ctrl Pts',(126.779460089513,38.3971171615454,0.));
#61583=CARTESIAN_POINT('Ctrl Pts',(127.755431446906,39.3383655845225,0.));
#61584=CARTESIAN_POINT('Ctrl Pts',(128.747640262206,40.2275943271253,0.));
#61585=CARTESIAN_POINT('Ctrl Pts',(129.763264721445,41.0619597887374,0.));
#61586=CARTESIAN_POINT('Ctrl Pts',(130.809844110982,41.8388975654704,0.));
#61587=CARTESIAN_POINT('Ctrl Pts',(131.894325225331,42.5564406463359,0.));
#61588=CARTESIAN_POINT('Ctrl Pts',(133.022036870624,43.2136312541229,0.));
#61589=CARTESIAN_POINT('Ctrl Pts',(134.195388228683,43.8112254901541,0.));
#61590=CARTESIAN_POINT('Ctrl Pts',(135.388188737997,44.3391341165731,0.));
#61591=CARTESIAN_POINT('Ctrl Pts',(136.371496319856,44.7166662230984,0.));
#61592=CARTESIAN_POINT('Ctrl Pts',(137.120711206628,44.9743239684511,0.));
#61593=CARTESIAN_POINT('Ctrl Pts',(137.618677570373,45.1331534198878,0.));
#61594=CARTESIAN_POINT('Ctrl Pts',(137.85505508508,45.205835364641,0.));
#61595=CARTESIAN_POINT('',(122.,-33.,-4.04133443718627E-15));
#61596=CARTESIAN_POINT('Origin',(122.,0.,0.));
#61597=CARTESIAN_POINT('Origin',(122.,0.,0.));
#61598=CARTESIAN_POINT('Origin',(104.414213562373,0.,0.));
#61599=CARTESIAN_POINT('',(104.414213562373,-4.04133443718627E-15,33.));
#61600=CARTESIAN_POINT('',(104.414213562373,-33.,-4.04133443718627E-15));
#61601=CARTESIAN_POINT('Origin',(104.414213562373,0.,0.));
#61602=CARTESIAN_POINT('Origin',(104.414213562373,0.,0.));
#61603=CARTESIAN_POINT('',(103.707106781187,-4.00546536289508E-15,32.7071067811865));
#61604=CARTESIAN_POINT('Origin',(104.414213562373,-3.91886975727153E-15,
32.));
#61605=CARTESIAN_POINT('',(103.707106781187,-32.7071067811865,-4.00546536289508E-15));
#61606=CARTESIAN_POINT('Origin',(103.707106781187,0.,-5.00683170361885E-15));
#61607=CARTESIAN_POINT('Origin',(103.707106781187,0.,-5.00683170361885E-15));
#61608=CARTESIAN_POINT('Origin',(100.5,0.,0.));
#61609=CARTESIAN_POINT('',(97.2928932188134,-26.2928932188134,-3.2199507520743E-15));
#61610=CARTESIAN_POINT('',(100.5,-29.5,-3.61270805748469E-15));
#61611=CARTESIAN_POINT('',(97.2928932188134,-3.2199507520743E-15,26.2928932188134));
#61612=CARTESIAN_POINT('Origin',(97.2928932188134,0.,-4.02493844009288E-15));
#61613=CARTESIAN_POINT('Origin',(97.2928932188134,0.,-4.02493844009288E-15));
#61614=CARTESIAN_POINT('Origin',(113.,0.,0.));
#61615=CARTESIAN_POINT('',(113.,-33.,-4.04133443718627E-15));
#61616=CARTESIAN_POINT('Origin',(98.,0.,0.));
#61617=CARTESIAN_POINT('',(97.,-3.13335514645075E-15,25.5857864376269));
#61618=CARTESIAN_POINT('Origin',(98.,-3.13335514645075E-15,25.5857864376269));
#61619=CARTESIAN_POINT('Origin',(97.,0.,0.));
#61620=CARTESIAN_POINT('Origin',(97.,26.,0.));
#61621=CARTESIAN_POINT('',(97.,-17.,-2.0818995585505E-15));
#61622=CARTESIAN_POINT('Origin',(97.,0.,0.));
#61623=CARTESIAN_POINT('Origin',(93.,0.,0.));
#61624=CARTESIAN_POINT('',(93.,-2.0818995585505E-15,17.));
#61625=CARTESIAN_POINT('',(93.,-17.,-2.0818995585505E-15));
#61626=CARTESIAN_POINT('Origin',(93.,0.,0.));
#61627=CARTESIAN_POINT('Origin',(93.,0.,0.));
#61628=CARTESIAN_POINT('',(92.,-1.95943487863577E-15,16.));
#61629=CARTESIAN_POINT('Origin',(93.,-1.95943487863577E-15,16.));
#61630=CARTESIAN_POINT('Origin',(92.,0.,0.));
#61631=CARTESIAN_POINT('Origin',(92.,17.,0.));
#61632=CARTESIAN_POINT('',(92.,-14.,-1.71450551880629E-15));
#61633=CARTESIAN_POINT('Origin',(92.,0.,0.));
#61634=CARTESIAN_POINT('Origin',(94.5,0.,0.));
#61635=CARTESIAN_POINT('',(94.5,-17.,-2.0818995585505E-15));
#61636=CARTESIAN_POINT('Origin',(89.,0.,0.));
#61637=CARTESIAN_POINT('',(89.,-1.71450551880629E-15,14.));
#61638=CARTESIAN_POINT('',(89.,-14.,-1.71450551880629E-15));
#61639=CARTESIAN_POINT('Origin',(89.,0.,0.));
#61640=CARTESIAN_POINT('Origin',(89.,0.,0.));
#61641=CARTESIAN_POINT('',(88.,-1.59204083889156E-15,13.));
#61642=CARTESIAN_POINT('Origin',(89.,-1.59204083889156E-15,13.));
#61643=CARTESIAN_POINT('Origin',(88.,0.,0.));
#61644=CARTESIAN_POINT('Origin',(88.,14.,0.));
#61645=CARTESIAN_POINT('',(88.,11.5,0.7));
#61646=CARTESIAN_POINT('',(88.,11.5,-0.7));
#61647=CARTESIAN_POINT('',(88.,11.5,0.7));
#61648=CARTESIAN_POINT('',(88.,11.3514471211877,1.97095110413219));
#61649=CARTESIAN_POINT('Origin',(88.,10.6623800874337,1.24625349616492));
#61650=CARTESIAN_POINT('',(88.,11.0285849021483,3.33321392294394));
#61651=CARTESIAN_POINT('',(88.,11.0285849021483,3.33321392294394));
#61652=CARTESIAN_POINT('',(88.,10.5909347898596,4.53564772407893));
#61653=CARTESIAN_POINT('Origin',(88.,10.0875684170659,3.67157463993582));
#61654=CARTESIAN_POINT('',(88.,9.96261593757892,5.7867334205317));
#61655=CARTESIAN_POINT('',(88.,9.96261593757892,5.7867334205317));
#61656=CARTESIAN_POINT('',(88.,9.25946242264883,6.85582640121192));
#61657=CARTESIAN_POINT('Origin',(88.,8.96893332226436,5.89896024451612));
#61658=CARTESIAN_POINT('',(88.,8.35955976908767,7.92828862157849));
#61659=CARTESIAN_POINT('',(88.,8.35955976908767,7.92828862157849));
#61660=CARTESIAN_POINT('',(88.,7.42881003951057,8.80640570249105));
#61661=CARTESIAN_POINT('Origin',(88.,7.36678071053768,7.80833137542559));
#61662=CARTESIAN_POINT('',(88.,6.30583756965351,9.64242773087495));
#61663=CARTESIAN_POINT('',(88.,6.30583756965351,9.64242773087495));
#61664=CARTESIAN_POINT('',(88.,5.1976685842665,10.2822293928957));
#61665=CARTESIAN_POINT('Origin',(88.,5.36748304388578,9.29675334077463));
#61666=CARTESIAN_POINT('',(88.,3.91216603463411,10.8367410653506));
#61667=CARTESIAN_POINT('',(88.,3.91216603463411,10.8367410653506));
#61668=CARTESIAN_POINT('',(88.,2.68631947027825,11.2037354352735));
#61669=CARTESIAN_POINT('Origin',(88.,3.07882297701681,10.2839849271476));
#61670=CARTESIAN_POINT('',(88.,1.30758861606115,11.4468428840072));
#61671=CARTESIAN_POINT('',(88.,1.30758861606115,11.4468428840072));
#61672=CARTESIAN_POINT('',(88.,0.0301501783194164,11.5212452003569));
#61673=CARTESIAN_POINT('Origin',(88.,0.624182766533239,10.7168042241878));
#61674=CARTESIAN_POINT('',(88.,-1.36748124326036,11.4398424398823));
#61675=CARTESIAN_POINT('',(88.,-1.36748124326036,11.4398424398823));
#61676=CARTESIAN_POINT('',(88.,-2.62764451755669,11.2176416545259));
#61677=CARTESIAN_POINT('Origin',(88.,-1.86410729845783,10.5718778315606));
#61678=CARTESIAN_POINT('',(88.,-3.96882983479838,10.8161171287304));
#61679=CARTESIAN_POINT('',(88.,-3.96882983479838,10.8161171287304));
#61680=CARTESIAN_POINT('',(88.,-5.14378221735089,10.309292143521));
#61681=CARTESIAN_POINT('Origin',(88.,-4.25190285648284,9.85701876860538));
#61682=CARTESIAN_POINT('',(88.,-6.3562177826491,9.60929214352105));
#61683=CARTESIAN_POINT('',(88.,-6.3562177826491,9.60929214352105));
#61684=CARTESIAN_POINT('',(88.,-7.3826172863893,8.84516602459817));
#61685=CARTESIAN_POINT('Origin',(88.,-6.41047723095084,8.61076527244046));
#61686=CARTESIAN_POINT('',(88.,-8.40094038459157,7.88442773158195));
#61687=CARTESIAN_POINT('',(88.,-8.40094038459157,7.88442773158195));
#61688=CARTESIAN_POINT('',(88.,-9.2234535465992,6.90419471580333));
#61689=CARTESIAN_POINT('Origin',(88.,-8.22346111860809,6.90030319162475));
#61690=CARTESIAN_POINT('',(88.,-9.99276611589833,5.73451177982522));
#61691=CARTESIAN_POINT('',(88.,-9.99276611589833,5.73451177982522));
#61692=CARTESIAN_POINT('',(88.,-10.56705103871,4.59101648279533));
#61693=CARTESIAN_POINT('Origin',(88.,-9.5931160887976,4.81784397967164));
#61694=CARTESIAN_POINT('',(88.,-11.0458792393659,3.27544681369506));
#61695=CARTESIAN_POINT('',(88.,-11.0458792393659,3.27544681369506));
#61696=CARTESIAN_POINT('',(88.,-11.3409760741447,2.03033536285951));
#61697=CARTESIAN_POINT('Origin',(88.,-10.4456036875545,2.47565355172201));
#61698=CARTESIAN_POINT('',(88.,-11.50350615392,0.639801662020789));
#61699=CARTESIAN_POINT('',(88.,-11.50350615392,0.639801662020789));
#61700=CARTESIAN_POINT('',(88.,-11.50350615392,-0.639801662020786));
#61701=CARTESIAN_POINT('Origin',(88.,-10.7349660877716,1.38777878078145E-15));
#61702=CARTESIAN_POINT('',(88.,-11.3409760741447,-2.03033536285951));
#61703=CARTESIAN_POINT('',(88.,-11.3409760741447,-2.03033536285951));
#61704=CARTESIAN_POINT('',(88.,-11.0458792393659,-3.27544681369505));
#61705=CARTESIAN_POINT('Origin',(88.,-10.4456036875545,-2.47565355172201));
#61706=CARTESIAN_POINT('',(88.,-10.56705103871,-4.59101648279533));
#61707=CARTESIAN_POINT('',(88.,-10.56705103871,-4.59101648279533));
#61708=CARTESIAN_POINT('',(88.,-9.99276611589833,-5.73451177982521));
#61709=CARTESIAN_POINT('Origin',(88.,-9.5931160887976,-4.81784397967164));
#61710=CARTESIAN_POINT('',(88.,-9.22345354659921,-6.90419471580332));
#61711=CARTESIAN_POINT('',(88.,-9.22345354659921,-6.90419471580332));
#61712=CARTESIAN_POINT('',(88.,-8.40094038459157,-7.88442773158195));
#61713=CARTESIAN_POINT('Origin',(88.,-8.22346111860809,-6.90030319162475));
#61714=CARTESIAN_POINT('',(88.,-7.3826172863893,-8.84516602459817));
#61715=CARTESIAN_POINT('',(88.,-7.3826172863893,-8.84516602459817));
#61716=CARTESIAN_POINT('',(88.,-6.35621778264911,-9.60929214352104));
#61717=CARTESIAN_POINT('Origin',(88.,-6.41047723095084,-8.61076527244045));
#61718=CARTESIAN_POINT('',(88.,-5.1437822173509,-10.309292143521));
#61719=CARTESIAN_POINT('',(88.,-5.1437822173509,-10.309292143521));
#61720=CARTESIAN_POINT('',(88.,-3.96882983479838,-10.8161171287304));
#61721=CARTESIAN_POINT('Origin',(88.,-4.25190285648285,-9.85701876860538));
#61722=CARTESIAN_POINT('',(88.,-2.6276445175567,-11.2176416545259));
#61723=CARTESIAN_POINT('',(88.,-2.6276445175567,-11.2176416545259));
#61724=CARTESIAN_POINT('',(88.,-1.36748124326036,-11.4398424398823));
#61725=CARTESIAN_POINT('Origin',(88.,-1.86410729845783,-10.5718778315606));
#61726=CARTESIAN_POINT('',(88.,0.0301501783194109,-11.5212452003569));
#61727=CARTESIAN_POINT('',(88.,0.0301501783194109,-11.5212452003569));
#61728=CARTESIAN_POINT('',(88.,1.30758861606115,-11.4468428840072));
#61729=CARTESIAN_POINT('Origin',(88.,0.624182766533234,-10.7168042241878));
#61730=CARTESIAN_POINT('',(88.,2.68631947027824,-11.2037354352735));
#61731=CARTESIAN_POINT('',(88.,2.68631947027824,-11.2037354352735));
#61732=CARTESIAN_POINT('',(88.,3.91216603463411,-10.8367410653506));
#61733=CARTESIAN_POINT('Origin',(88.,3.07882297701681,-10.2839849271476));
#61734=CARTESIAN_POINT('',(88.,5.19766858426649,-10.2822293928957));
#61735=CARTESIAN_POINT('',(88.,5.19766858426649,-10.2822293928957));
#61736=CARTESIAN_POINT('',(88.,6.30583756965351,-9.64242773087496));
#61737=CARTESIAN_POINT('Origin',(88.,5.36748304388578,-9.29675334077463));
#61738=CARTESIAN_POINT('',(88.,7.42881003951057,-8.80640570249106));
#61739=CARTESIAN_POINT('',(88.,7.42881003951057,-8.80640570249106));
#61740=CARTESIAN_POINT('',(88.,8.35955976908767,-7.92828862157849));
#61741=CARTESIAN_POINT('Origin',(88.,7.36678071053767,-7.8083313754256));
#61742=CARTESIAN_POINT('',(88.,9.25946242264882,-6.85582640121192));
#61743=CARTESIAN_POINT('',(88.,9.25946242264882,-6.85582640121192));
#61744=CARTESIAN_POINT('',(88.,9.96261593757892,-5.78673342053171));
#61745=CARTESIAN_POINT('Origin',(88.,8.96893332226436,-5.89896024451612));
#61746=CARTESIAN_POINT('',(88.,10.5909347898596,-4.53564772407893));
#61747=CARTESIAN_POINT('',(88.,10.5909347898596,-4.53564772407893));
#61748=CARTESIAN_POINT('',(88.,11.0285849021483,-3.33321392294394));
#61749=CARTESIAN_POINT('Origin',(88.,10.0875684170659,-3.67157463993583));
#61750=CARTESIAN_POINT('',(88.,11.3514471211877,-1.97095110413219));
#61751=CARTESIAN_POINT('',(88.,11.3514471211877,-1.97095110413219));
#61752=CARTESIAN_POINT('Origin',(88.,10.6623800874337,-1.24625349616493));
#61753=CARTESIAN_POINT('Origin',(90.,0.,0.));
#61754=CARTESIAN_POINT('',(90.,-14.,-1.71450551880629E-15));
#61755=CARTESIAN_POINT('Ctrl Pts',(127.110025063046,-14.1660632471973,-13.6372179765762));
#61756=CARTESIAN_POINT('Ctrl Pts',(126.561429493857,-11.2405277823208,-15.7553971673589));
#61757=CARTESIAN_POINT('Ctrl Pts',(126.561429493857,-8.02431030248638,-17.6122811951138));
#61758=CARTESIAN_POINT('Ctrl Pts',(127.110025063046,-4.72714558106274,-19.0867796319777));
#61759=CARTESIAN_POINT('Ctrl Pts',(127.362931194533,-14.0316094882686,-13.5170175430695));
#61760=CARTESIAN_POINT('Ctrl Pts',(126.820035970083,-11.1364717038075,-15.6131877334422));
#61761=CARTESIAN_POINT('Ctrl Pts',(126.820035970083,-7.95318135931332,-17.4510612707447));
#61762=CARTESIAN_POINT('Ctrl Pts',(127.362931194533,-4.69027583156434,-18.9102390443579));
#61763=CARTESIAN_POINT('Ctrl Pts',(127.647216190801,-13.68668967427,-13.1142576336319));
#61764=CARTESIAN_POINT('Ctrl Pts',(127.114082771185,-10.8436088537941,-15.1727363627014));
#61765=CARTESIAN_POINT('Ctrl Pts',(127.114082771185,-7.7181707081268,-16.977208917438));
#61766=CARTESIAN_POINT('Ctrl Pts',(127.647216190801,-4.51393542536476,-18.4101497684477));
#61767=CARTESIAN_POINT('Ctrl Pts',(127.47007422846,-13.3854383233912,-12.6523038901745));
#61768=CARTESIAN_POINT('Ctrl Pts',(126.93997655279,-10.5585493016115,-14.6990589472656));
#61769=CARTESIAN_POINT('Ctrl Pts',(126.93997655279,-7.45048380925175,-16.4935013959386));
#61770=CARTESIAN_POINT('Ctrl Pts',(127.47007422846,-4.26449742359677,-17.9182815739335));
#61771=CARTESIAN_POINT('Ctrl Pts',(127.328278974586,-13.295217287153,-12.4909704719789));
#61772=CARTESIAN_POINT('Ctrl Pts',(126.797908763857,-10.466876396916,-14.5387767698242));
#61773=CARTESIAN_POINT('Ctrl Pts',(126.797908763857,-7.35751182416132,-16.3339692429128));
#61774=CARTESIAN_POINT('Ctrl Pts',(127.328278974586,-4.16988910307908,-17.7594811554977));
#61775=CARTESIAN_POINT('',(127.328278974586,-4.16988910307908,-17.7594811554977));
#61776=CARTESIAN_POINT('',(127.464921070561,-4.72164036362646,-17.9837982557428));
#61777=CARTESIAN_POINT('Ctrl Pts',(127.328278974584,-4.16988910307848,-17.7594811554948));
#61778=CARTESIAN_POINT('Ctrl Pts',(127.328985683097,-4.17159829893104,-17.7599820161575));
#61779=CARTESIAN_POINT('Ctrl Pts',(127.32968995025,-4.17330794100423,-17.7604848064164));
#61780=CARTESIAN_POINT('Ctrl Pts',(127.404564207109,-4.35574867200842,-17.8143308393875));
#61781=CARTESIAN_POINT('Ctrl Pts',(127.452250527053,-4.54335712495651,-17.8897928354679));
#61782=CARTESIAN_POINT('Ctrl Pts',(127.464921070561,-4.72164036362227,-17.9837982557406));
#61783=CARTESIAN_POINT('',(127.328278974586,-13.295217287153,-12.4909704719789));
#61784=CARTESIAN_POINT('Ctrl Pts',(127.328278974586,-4.16988910307908,-17.7594811554977));
#61785=CARTESIAN_POINT('Ctrl Pts',(126.797908763857,-7.35751182416132,-16.3339692429128));
#61786=CARTESIAN_POINT('Ctrl Pts',(126.797908763857,-10.466876396916,-14.5387767698242));
#61787=CARTESIAN_POINT('Ctrl Pts',(127.328278974586,-13.295217287153,-12.4909704719789));
#61788=CARTESIAN_POINT('',(127.464921070561,-13.2136059641945,-13.0809596303012));
#61789=CARTESIAN_POINT('Ctrl Pts',(127.464921070561,-13.2136059641945,-13.0809596303012));
#61790=CARTESIAN_POINT('Ctrl Pts',(127.452250527052,-13.2213365014783,-12.8795591063997));
#61791=CARTESIAN_POINT('Ctrl Pts',(127.404564207055,-13.2497887222992,-12.6793544220839));
#61792=CARTESIAN_POINT('Ctrl Pts',(127.329689950251,-13.2943770553836,-12.4944330979339));
#61793=CARTESIAN_POINT('Ctrl Pts',(127.3289856831,-13.2947964472842,-12.4927011093395));
#61794=CARTESIAN_POINT('Ctrl Pts',(127.328278974586,-13.295217287153,-12.4909704719789));
#61795=CARTESIAN_POINT('',(126.797085404885,-11.8793261399438,-15.2022528231739));
#61796=CARTESIAN_POINT('Ctrl Pts',(126.797085404885,-11.8793261399438,-15.2022528231739));
#61797=CARTESIAN_POINT('Ctrl Pts',(127.006996076072,-12.4284032417257,-14.7210474214397));
#61798=CARTESIAN_POINT('Ctrl Pts',(127.231020546675,-12.8008456764682,-14.2508721651692));
#61799=CARTESIAN_POINT('Ctrl Pts',(127.422304943631,-13.1154157241859,-13.5911945182249));
#61800=CARTESIAN_POINT('Ctrl Pts',(127.458876008142,-13.1746427896695,-13.3958546673502));
#61801=CARTESIAN_POINT('Ctrl Pts',(127.468170789171,-13.2074104105918,-13.1741543020807));
#61802=CARTESIAN_POINT('Ctrl Pts',(127.467776491121,-13.21186381832,-13.1263470437446));
#61803=CARTESIAN_POINT('Ctrl Pts',(127.464921070561,-13.2136059641945,-13.0809596303012));
#61804=CARTESIAN_POINT('',(126.797085404885,-7.22587406965037,-17.8889246286188));
#61805=CARTESIAN_POINT('Ctrl Pts',(126.797739711379,-11.8790433321593,-15.201904292993));
#61806=CARTESIAN_POINT('Ctrl Pts',(126.665524611079,-10.3768517946564,-16.1726158137204));
#61807=CARTESIAN_POINT('Ctrl Pts',(126.665524611079,-8.81747024299963,-17.0729251723388));
#61808=CARTESIAN_POINT('Ctrl Pts',(126.797739711379,-7.22571363755199,-17.8885054448026));
#61809=CARTESIAN_POINT('Ctrl Pts',(127.464921070561,-4.72164036362645,-17.9837982557428));
#61810=CARTESIAN_POINT('Ctrl Pts',(127.468398488078,-4.77057001346949,-18.0095979457847));
#61811=CARTESIAN_POINT('Ctrl Pts',(127.468025475808,-4.8217199022571,-18.0321668235633));
#61812=CARTESIAN_POINT('Ctrl Pts',(127.456769053802,-5.0134023579572,-18.1047856321494));
#61813=CARTESIAN_POINT('Ctrl Pts',(127.427486401576,-5.18000926912678,-18.1447123913595));
#61814=CARTESIAN_POINT('Ctrl Pts',(127.322999543191,-5.60156722060295,-18.1899973333731));
#61815=CARTESIAN_POINT('Ctrl Pts',(127.242195869014,-5.86018690005347,-18.1870904290045));
#61816=CARTESIAN_POINT('Ctrl Pts',(127.036712870258,-6.48459473410091,-18.1063632325042));
#61817=CARTESIAN_POINT('Ctrl Pts',(126.91366853489,-6.84194426602908,-18.0193933569077));
#61818=CARTESIAN_POINT('Ctrl Pts',(126.797085404885,-7.22587406965036,-17.8889246286188));
#61819=CARTESIAN_POINT('Origin',(133.079689783217,-7.42462120245877,-12.8598211496117));
#61820=CARTESIAN_POINT('Origin',(133.079689783217,-7.42462120245877,-12.8598211496117));
#61821=CARTESIAN_POINT('Ctrl Pts',(127.110025063046,-4.72714558106216,19.086779631978));
#61822=CARTESIAN_POINT('Ctrl Pts',(126.56142949942,-8.02431026905037,17.6122812100665));
#61823=CARTESIAN_POINT('Ctrl Pts',(126.561429543075,-11.2405280447897,15.7553969773232));
#61824=CARTESIAN_POINT('Ctrl Pts',(127.110025063046,-14.1660632471965,13.6372179765768));
#61825=CARTESIAN_POINT('Ctrl Pts',(127.362931194533,-4.69027583156377,18.9102390443581));
#61826=CARTESIAN_POINT('Ctrl Pts',(126.820035975589,-7.95318132622473,17.451061285542));
#61827=CARTESIAN_POINT('Ctrl Pts',(126.82003601879,-11.1364719635492,15.613187545381));
#61828=CARTESIAN_POINT('Ctrl Pts',(127.362931194533,-14.0316094882678,13.51701754307));
#61829=CARTESIAN_POINT('Ctrl Pts',(127.647216190801,-4.5139354253642,18.4101497684479));
#61830=CARTESIAN_POINT('Ctrl Pts',(127.114082776592,-7.71817067563316,16.9772089319693));
#61831=CARTESIAN_POINT('Ctrl Pts',(127.114082819016,-10.8436091088655,15.1727361780217));
#61832=CARTESIAN_POINT('Ctrl Pts',(127.647216190801,-13.6866896742692,13.1142576336324));
#61833=CARTESIAN_POINT('Ctrl Pts',(127.47007422846,-4.26449742359621,17.9182815739338));
#61834=CARTESIAN_POINT('Ctrl Pts',(126.939976558165,-7.45048377694319,16.4935014103871));
#61835=CARTESIAN_POINT('Ctrl Pts',(126.939976600348,-10.5585495552302,14.6990587636378));
#61836=CARTESIAN_POINT('Ctrl Pts',(127.47007422846,-13.3854383233904,12.6523038901751));
#61837=CARTESIAN_POINT('Ctrl Pts',(127.328278974586,-4.16988910307852,17.759481155498));
#61838=CARTESIAN_POINT('Ctrl Pts',(126.797908769235,-7.35751179183616,16.3339692573687));
#61839=CARTESIAN_POINT('Ctrl Pts',(126.79790881144,-10.466876650665,14.538776586102));
#61840=CARTESIAN_POINT('Ctrl Pts',(127.328278974586,-13.2952172871522,12.4909704719795));
#61841=CARTESIAN_POINT('',(127.328278974586,-13.2952172871522,12.4909704719795));
#61842=CARTESIAN_POINT('',(127.328278974586,-4.16988910307852,17.759481155498));
#61843=CARTESIAN_POINT('Ctrl Pts',(127.328278974586,-13.2952172871522,12.4909704719795));
#61844=CARTESIAN_POINT('Ctrl Pts',(126.79790881144,-10.466876650665,14.538776586102));
#61845=CARTESIAN_POINT('Ctrl Pts',(126.797908769235,-7.35751179183616,16.3339692573687));
#61846=CARTESIAN_POINT('Ctrl Pts',(127.328278974586,-4.16988910307852,17.759481155498));
#61847=CARTESIAN_POINT('',(127.464921070561,-4.72164036362226,17.9837982557406));
#61848=CARTESIAN_POINT('Ctrl Pts',(127.464921070561,-4.72164036362226,17.9837982557406));
#61849=CARTESIAN_POINT('Ctrl Pts',(127.452250527055,-4.54335712498583,17.8897928354834));
#61850=CARTESIAN_POINT('Ctrl Pts',(127.404564207251,-4.3557486721359,17.8143308395414));
#61851=CARTESIAN_POINT('Ctrl Pts',(127.329689950245,-4.17330794100013,17.7604848064107));
#61852=CARTESIAN_POINT('Ctrl Pts',(127.328985683104,-4.17159829894034,17.7599820161634));
#61853=CARTESIAN_POINT('Ctrl Pts',(127.328278974586,-4.16988910307852,17.759481155498));
#61854=CARTESIAN_POINT('',(126.797085404885,-7.22587406965043,17.8889246286188));
#61855=CARTESIAN_POINT('Ctrl Pts',(126.797085404885,-7.22587406965036,17.8889246286188));
#61856=CARTESIAN_POINT('Ctrl Pts',(127.006996076078,-6.53459941639848,18.1238366465383));
#61857=CARTESIAN_POINT('Ctrl Pts',(127.231020546687,-5.94119448285199,18.211293628335));
#61858=CARTESIAN_POINT('Ctrl Pts',(127.422304943639,-5.21261185842928,18.1538804574448));
#61859=CARTESIAN_POINT('Ctrl Pts',(127.458876008146,-5.01382905246405,18.1075026753055));
#61860=CARTESIAN_POINT('Ctrl Pts',(127.46817078917,-4.80544709366776,18.0250300848132));
#61861=CARTESIAN_POINT('Ctrl Pts',(127.467776491121,-4.76181808960751,18.0049832198747));
#61862=CARTESIAN_POINT('Ctrl Pts',(127.464921070561,-4.72164036362226,17.9837982557406));
#61863=CARTESIAN_POINT('',(126.797085404885,-11.8793261399439,15.2022528231739));
#61864=CARTESIAN_POINT('Ctrl Pts',(126.79773972309,-7.22571363467581,17.8885054373022));
#61865=CARTESIAN_POINT('Ctrl Pts',(126.665524631933,-8.8174702476118,17.0729251533641));
#61866=CARTESIAN_POINT('Ctrl Pts',(126.665524637149,-10.3768518330538,16.1726157711598));
#61867=CARTESIAN_POINT('Ctrl Pts',(126.797739723243,-11.8790433270359,15.2019042866705));
#61868=CARTESIAN_POINT('',(127.464921070561,-13.2136059641945,13.0809596303012));
#61869=CARTESIAN_POINT('Ctrl Pts',(126.797085404885,-11.8793261399439,15.2022528231738));
#61870=CARTESIAN_POINT('Ctrl Pts',(126.913668534864,-12.1842802747836,14.9349942241724));
#61871=CARTESIAN_POINT('Ctrl Pts',(127.036712870204,-12.4382731623349,14.6690053893477));
#61872=CARTESIAN_POINT('Ctrl Pts',(127.242195868974,-12.8203888823498,14.168615940985));
#61873=CARTESIAN_POINT('Ctrl Pts',(127.322999543176,-12.9522161751463,13.9460981807893));
#61874=CARTESIAN_POINT('Ctrl Pts',(127.427486401576,-13.1237772407162,13.5583758145833));
#61875=CARTESIAN_POINT('Ctrl Pts',(127.456769053803,-13.1725031085346,13.3941266174573));
#61876=CARTESIAN_POINT('Ctrl Pts',(127.468025475808,-13.2054546033566,13.1918153370665));
#61877=CARTESIAN_POINT('Ctrl Pts',(127.468398488078,-13.2114843262592,13.1362337950855));
#61878=CARTESIAN_POINT('Ctrl Pts',(127.464921070561,-13.2136059641945,13.0809596303012));
#61879=CARTESIAN_POINT('Ctrl Pts',(127.464921070561,-13.2136059641945,13.0809596303012));
#61880=CARTESIAN_POINT('Ctrl Pts',(127.452250527053,-13.2213365014774,12.8795591064215));
#61881=CARTESIAN_POINT('Ctrl Pts',(127.40456420715,-13.2497887223457,12.6793544222081));
#61882=CARTESIAN_POINT('Ctrl Pts',(127.329689950249,-13.2943770553813,12.4944330979308));
#61883=CARTESIAN_POINT('Ctrl Pts',(127.328985683102,-13.2947964472824,12.4927011093444));
#61884=CARTESIAN_POINT('Ctrl Pts',(127.328278974586,-13.2952172871522,12.4909704719795));
#61885=CARTESIAN_POINT('Ctrl Pts',(127.223161057304,-13.0166384114774,12.850678779398));
#61886=CARTESIAN_POINT('Ctrl Pts',(129.536338172585,-14.9251180734187,15.0856868726168));
#61887=CARTESIAN_POINT('Ctrl Pts',(136.26235662497,-18.8252609361828,19.4192573625422));
#61888=CARTESIAN_POINT('Ctrl Pts',(145.009334196347,-20.6565416977987,21.0246267351951));
#61889=CARTESIAN_POINT('Ctrl Pts',(150.052765342883,-20.8995467586362,20.8872820358768));
#61890=CARTESIAN_POINT('Ctrl Pts',(127.284956078127,-13.0852837400993,12.72359605321));
#61891=CARTESIAN_POINT('Ctrl Pts',(129.605785369344,-14.989338089773,14.9334825814221));
#61892=CARTESIAN_POINT('Ctrl Pts',(136.344248889854,-18.8639156576751,19.1982227546206));
#61893=CARTESIAN_POINT('Ctrl Pts',(145.047721141658,-20.6291059319939,20.731619174958));
#61894=CARTESIAN_POINT('Ctrl Pts',(150.04110192192,-20.8302776360491,20.5710296934056));
#61895=CARTESIAN_POINT('Ctrl Pts',(127.321297410279,-13.1815939383355,12.5992378142346));
#61896=CARTESIAN_POINT('Ctrl Pts',(129.646063027636,-15.0920259101955,14.7851525894515));
#61897=CARTESIAN_POINT('Ctrl Pts',(136.391015543887,-18.9766896378183,18.9837203153837));
#61898=CARTESIAN_POINT('Ctrl Pts',(145.066397533214,-20.7324885411619,20.4301204760333));
#61899=CARTESIAN_POINT('Ctrl Pts',(150.020700025828,-20.9266035081301,20.2235460492494));
#61900=CARTESIAN_POINT('Ctrl Pts',(127.328278974586,-13.2952172871522,12.4909704719795));
#61901=CARTESIAN_POINT('Ctrl Pts',(129.651808158315,-15.2194053330612,14.6601796019475));
#61902=CARTESIAN_POINT('Ctrl Pts',(136.392499004845,-19.1389221942341,18.8169239233383));
#61903=CARTESIAN_POINT('Ctrl Pts',(145.055988199056,-20.9311521385778,20.218566086275));
#61904=CARTESIAN_POINT('Ctrl Pts',(150.,-21.1486739792529,19.988586466263));
#61905=CARTESIAN_POINT('',(127.849160658777,-13.5167868848207,13.4339138050526));
#61906=CARTESIAN_POINT('',(150.052765342883,-20.8995467586362,20.8872820358768));
#61907=CARTESIAN_POINT('Ctrl Pts',(127.84924144537,-13.5166592276754,13.4339349354541));
#61908=CARTESIAN_POINT('Ctrl Pts',(130.048406672691,-15.2174026484228,15.4098381536351));
#61909=CARTESIAN_POINT('Ctrl Pts',(136.59343849021,-18.8945767478887,19.4800222018206));
#61910=CARTESIAN_POINT('Ctrl Pts',(145.009334196347,-20.6565416977987,21.0246267351951));
#61911=CARTESIAN_POINT('Ctrl Pts',(150.052765342883,-20.8995467586362,20.8872820358768));
#61912=CARTESIAN_POINT('',(150.,-21.1486739792529,19.988586466263));
#61913=CARTESIAN_POINT('Origin',(149.99997684747,-21.8754325350461,20.6754794717924));
#61914=CARTESIAN_POINT('Ctrl Pts',(150.,-21.1486739792529,19.988586466263));
#61915=CARTESIAN_POINT('Ctrl Pts',(145.055988199056,-20.9311521385778,20.218566086275));
#61916=CARTESIAN_POINT('Ctrl Pts',(136.392499004845,-19.1389221942341,18.8169239233383));
#61917=CARTESIAN_POINT('Ctrl Pts',(129.651808158315,-15.2194053330612,14.6601796019475));
#61918=CARTESIAN_POINT('Ctrl Pts',(127.328278974586,-13.2952172871522,12.4909704719795));
#61919=CARTESIAN_POINT('Ctrl Pts',(127.84924144537,-13.5166592276754,13.4339349354541));
#61920=CARTESIAN_POINT('Ctrl Pts',(127.719533474886,-13.4163484485308,13.31739508064));
#61921=CARTESIAN_POINT('Ctrl Pts',(127.591421241578,-13.3153159262048,13.1997314770874));
#61922=CARTESIAN_POINT('Ctrl Pts',(127.464935561083,-13.2135838941545,13.0809632999976));
#61923=CARTESIAN_POINT('Ctrl Pts',(150.052765342888,-20.8995467586979,20.8872820361599));
#61924=CARTESIAN_POINT('Ctrl Pts',(152.168614364752,-21.0014822383913,20.8296099220071));
#61925=CARTESIAN_POINT('Ctrl Pts',(155.727083527126,-21.0459414018894,20.8146895081192));
#61926=CARTESIAN_POINT('Ctrl Pts',(160.687973683745,-20.9022688578489,20.8786948980203));
#61927=CARTESIAN_POINT('Ctrl Pts',(163.482362716732,-20.6580466346156,21.035876132756));
#61928=CARTESIAN_POINT('Ctrl Pts',(164.848300728213,-20.4572239433831,21.184196913403));
#61929=CARTESIAN_POINT('Ctrl Pts',(150.041092860165,-20.830277132788,20.5710296330652));
#61930=CARTESIAN_POINT('Ctrl Pts',(152.16392933006,-20.9162606478088,20.5038015525472));
#61931=CARTESIAN_POINT('Ctrl Pts',(155.727760367419,-20.9488880377099,20.4839037879759));
#61932=CARTESIAN_POINT('Ctrl Pts',(160.700196810596,-20.8351178347578,20.5627442654911));
#61933=CARTESIAN_POINT('Ctrl Pts',(163.509373737758,-20.6203677501259,20.7413000782778));
#61934=CARTESIAN_POINT('Ctrl Pts',(164.886050420642,-20.4340175279255,20.9042590799178));
#61935=CARTESIAN_POINT('Ctrl Pts',(150.020682003358,-20.9266030458978,20.2235458405872));
#61936=CARTESIAN_POINT('Ctrl Pts',(152.15474091165,-21.0094973016289,20.1374874488995));
#61937=CARTESIAN_POINT('Ctrl Pts',(155.729294662698,-21.039293174712,20.1053338731533));
#61938=CARTESIAN_POINT('Ctrl Pts',(160.722337303143,-20.9324362287602,20.2174477763172));
#61939=CARTESIAN_POINT('Ctrl Pts',(163.552607007736,-20.7223253727304,20.4336712388464));
#61940=CARTESIAN_POINT('Ctrl Pts',(164.942784454695,-20.5365303501091,20.6188742740247));
#61941=CARTESIAN_POINT('Ctrl Pts',(149.999976847469,-21.1486739791311,19.9885864663918));
#61942=CARTESIAN_POINT('Ctrl Pts',(152.145392515568,-21.2399176851882,19.8920472040836));
#61943=CARTESIAN_POINT('Ctrl Pts',(155.730853635437,-21.2754776366889,19.8537269301498));
#61944=CARTESIAN_POINT('Ctrl Pts',(160.744845538776,-21.1541157848699,19.983554404702));
#61945=CARTESIAN_POINT('Ctrl Pts',(163.596300012013,-20.9276206556128,20.2218429808621));
#61946=CARTESIAN_POINT('Ctrl Pts',(164.99999999999,-20.7313296143911,20.4211158465808));
#61947=CARTESIAN_POINT('',(164.84830072822,-20.4572239433773,21.1841969133289));
#61948=CARTESIAN_POINT('Ctrl Pts',(150.052765342888,-20.8995467586979,20.8872820361599));
#61949=CARTESIAN_POINT('Ctrl Pts',(152.168614364752,-21.0014822383913,20.8296099220071));
#61950=CARTESIAN_POINT('Ctrl Pts',(155.727083527126,-21.0459414018894,20.8146895081192));
#61951=CARTESIAN_POINT('Ctrl Pts',(160.687973683745,-20.9022688578489,20.8786948980203));
#61952=CARTESIAN_POINT('Ctrl Pts',(163.482362716732,-20.6580466346156,21.035876132756));
#61953=CARTESIAN_POINT('Ctrl Pts',(164.848300728213,-20.4572239433831,21.184196913403));
#61954=CARTESIAN_POINT('',(164.999999999995,-20.7313296143911,20.4211158465808));
#61955=CARTESIAN_POINT('Origin',(164.99999999999,-21.4437464396279,21.1228724048825));
#61956=CARTESIAN_POINT('Ctrl Pts',(164.99999999999,-20.7313296143911,20.4211158465808));
#61957=CARTESIAN_POINT('Ctrl Pts',(163.596300012013,-20.9276206556128,20.2218429808621));
#61958=CARTESIAN_POINT('Ctrl Pts',(160.744845538776,-21.1541157848699,19.983554404702));
#61959=CARTESIAN_POINT('Ctrl Pts',(155.730861335799,-21.2754774503045,19.8537271295355));
#61960=CARTESIAN_POINT('Ctrl Pts',(152.145407933657,-21.2399178381014,19.8920470393006));
#61961=CARTESIAN_POINT('Ctrl Pts',(149.999999911593,-21.1486749600368,19.9885854285569));
#61962=CARTESIAN_POINT('Origin',(165.,-21.4437464396264,21.122872404884));
#61963=CARTESIAN_POINT('',(166.,-21.4437464396264,21.122872404884));
#61964=CARTESIAN_POINT('Origin',(165.,-21.4437464396264,21.122872404884));
#61965=CARTESIAN_POINT('Origin',(165.,-21.4437464396264,21.122872404884));
#61966=CARTESIAN_POINT('Origin',(155.,-2.16262821021008E-15,3.7457819379656E-15));
#61967=CARTESIAN_POINT('Origin',(133.079689783217,-7.42462120245876,12.8598211496117));
#61968=CARTESIAN_POINT('',(127.849160658792,-4.87571718501769,18.4228377223367));
#61969=CARTESIAN_POINT('Ctrl Pts',(127.849390667086,-4.87581470104128,18.4225978737216));
#61970=CARTESIAN_POINT('Ctrl Pts',(127.719628690952,-4.82503943619891,18.2775158074239));
#61971=CARTESIAN_POINT('Ctrl Pts',(127.591474106961,-4.77365180285337,18.131227740728));
#61972=CARTESIAN_POINT('Ctrl Pts',(127.46495979063,-4.72165726175225,17.9837590795965));
#61973=CARTESIAN_POINT('',(150.052788176347,-7.63914239096105,28.5431800801744));
#61974=CARTESIAN_POINT('Ctrl Pts',(150.052788176357,-7.63914239116796,28.5431800803631));
#61975=CARTESIAN_POINT('Ctrl Pts',(146.270211473775,-7.81947858844008,28.4368505439217));
#61976=CARTESIAN_POINT('Ctrl Pts',(137.824456097629,-7.57922352157927,26.6726941211179));
#61977=CARTESIAN_POINT('Ctrl Pts',(130.853617533383,-6.0513548656332,21.7815128222562));
#61978=CARTESIAN_POINT('Ctrl Pts',(127.849390667086,-4.87581470104129,18.4225978737216));
#61979=CARTESIAN_POINT('',(164.848300728221,-8.1174407140519,28.3085740825534));
#61980=CARTESIAN_POINT('Ctrl Pts',(164.848300728217,-8.11744071408804,28.3085740825782));
#61981=CARTESIAN_POINT('Ctrl Pts',(162.79928054118,-7.77413038830263,28.4582180905047));
#61982=CARTESIAN_POINT('Ctrl Pts',(157.868876531342,-7.48949828735272,28.6380029652797));
#61983=CARTESIAN_POINT('Ctrl Pts',(152.874076231524,-7.50458485181733,28.6224409171841));
#61984=CARTESIAN_POINT('Ctrl Pts',(150.052788176347,-7.63914239096105,28.5431800801744));
#61985=CARTESIAN_POINT('Ctrl Pts',(164.848300728225,-20.4572239433766,21.1841969133291));
#61986=CARTESIAN_POINT('Ctrl Pts',(164.823285605772,-20.5140374352135,22.0362707934392));
#61987=CARTESIAN_POINT('Ctrl Pts',(164.75934857031,-20.3154311261898,24.6124011045219));
#61988=CARTESIAN_POINT('Ctrl Pts',(164.707290846802,-17.981646634823,28.4204658567131));
#61989=CARTESIAN_POINT('Ctrl Pts',(164.727957731471,-12.9552328630782,30.2918070911301));
#61990=CARTESIAN_POINT('Ctrl Pts',(164.798266641053,-9.53657145358806,29.2591248126568));
#61991=CARTESIAN_POINT('Ctrl Pts',(164.848300728224,-8.11744071405221,28.3085740825531));
#61992=CARTESIAN_POINT('Origin',(133.079689783217,-7.42462120245876,12.8598211496117));
#61993=CARTESIAN_POINT('Origin',(165.,0.,0.));
#61994=CARTESIAN_POINT('',(166.,21.4437464433745,21.1228723912929));
#61995=CARTESIAN_POINT('',(164.999999999999,20.7313296143898,20.4211158465821));
#61996=CARTESIAN_POINT('Origin',(165.,21.443746448267,21.1228723961122));
#61997=CARTESIAN_POINT('',(165.,28.05086990396,7.74330017699907));
#61998=CARTESIAN_POINT('Origin',(165.,0.,0.));
#61999=CARTESIAN_POINT('',(166.,29.0148173225344,8.00939296740403));
#62000=CARTESIAN_POINT('Origin',(165.,29.01481732334,8.00939296658667));
#62001=CARTESIAN_POINT('Origin',(166.,0.,0.));
#62002=CARTESIAN_POINT('Origin',(165.,29.0148173233401,8.00939296658655));
#62003=CARTESIAN_POINT('',(164.848300728223,28.5746646574706,7.12437716917368));
#62004=CARTESIAN_POINT('Origin',(165.,29.0148173233401,8.00939296658655));
#62005=CARTESIAN_POINT('Origin',(165.,29.0148173233401,8.00939296658655));
#62006=CARTESIAN_POINT('Origin',(165.,21.4437464396264,21.122872404884));
#62007=CARTESIAN_POINT('',(164.848300728223,20.4572239433816,21.1841969134041));
#62008=CARTESIAN_POINT('Origin',(165.,21.4437464396264,21.122872404884));
#62009=CARTESIAN_POINT('Origin',(165.,21.4437464396264,21.122872404884));
#62010=CARTESIAN_POINT('Ctrl Pts',(164.848300728252,28.5746646565963,7.1243771696036));
#62011=CARTESIAN_POINT('Ctrl Pts',(164.798268611144,30.1073707543423,6.37067894077189));
#62012=CARTESIAN_POINT('Ctrl Pts',(164.745477438778,32.0467280643695,4.53577823360106));
#62013=CARTESIAN_POINT('Ctrl Pts',(164.71073409437,33.4494761918939,0.472503961020967));
#62014=CARTESIAN_POINT('Ctrl Pts',(164.727959708039,32.7124405641852,-3.92265740596007));
#62015=CARTESIAN_POINT('Ctrl Pts',(164.798272182662,30.1072613429598,-6.37073274289246));
#62016=CARTESIAN_POINT('Ctrl Pts',(164.848300728223,28.5746646574706,-7.12437716917367));
#62017=CARTESIAN_POINT('Ctrl Pts',(165.010504706359,28.5635790515523,7.10208732257682));
#62018=CARTESIAN_POINT('Ctrl Pts',(164.963970790674,30.0878567187018,6.34256556658988));
#62019=CARTESIAN_POINT('Ctrl Pts',(164.913918379619,32.0092710212895,4.50839673351639));
#62020=CARTESIAN_POINT('Ctrl Pts',(164.880672535368,33.3956678994461,0.468713022336729));
#62021=CARTESIAN_POINT('Ctrl Pts',(164.897255208906,32.6682235041391,-3.89559855012971));
#62022=CARTESIAN_POINT('Ctrl Pts',(164.963974112475,30.0877479089765,-6.3426197844215));
#62023=CARTESIAN_POINT('Ctrl Pts',(165.010504706333,28.5635790524218,-7.10208732214358));
#62024=CARTESIAN_POINT('Ctrl Pts',(165.346644572289,28.577851547278,7.13078505672422));
#62025=CARTESIAN_POINT('Ctrl Pts',(165.311962519107,30.1017315158216,6.35628737215189));
#62026=CARTESIAN_POINT('Ctrl Pts',(165.27352501266,32.0121197971322,4.50723425184124));
#62027=CARTESIAN_POINT('Ctrl Pts',(165.247690070806,33.3854773884748,0.467146747979118));
#62028=CARTESIAN_POINT('Ctrl Pts',(165.260681136784,32.6663942515384,-3.88951477984603));
#62029=CARTESIAN_POINT('Ctrl Pts',(165.311964994867,30.1016227344833,-6.35634265903258));
#62030=CARTESIAN_POINT('Ctrl Pts',(165.346644572269,28.5778515481473,-7.13078505628244));
#62031=CARTESIAN_POINT('Ctrl Pts',(165.840927381351,28.7234819136511,7.42360430980067));
#62032=CARTESIAN_POINT('Ctrl Pts',(165.831141900203,30.3032763857957,6.61671644918394));
#62033=CARTESIAN_POINT('Ctrl Pts',(165.819970059155,32.2849054071351,4.69111567585252));
#62034=CARTESIAN_POINT('Ctrl Pts',(165.812323799273,33.7094564748683,0.48607004647879));
#62035=CARTESIAN_POINT('Ctrl Pts',(165.816209773846,32.9635803020626,-4.04779114102858));
#62036=CARTESIAN_POINT('Ctrl Pts',(165.831142598734,30.3031636130314,-6.61677404821087));
#62037=CARTESIAN_POINT('Ctrl Pts',(165.840927381346,28.7234819145522,-7.42360430934041));
#62038=CARTESIAN_POINT('Ctrl Pts',(166.,28.9052030350057,7.78899131217205));
#62039=CARTESIAN_POINT('Ctrl Pts',(166.000188635531,30.5621552739351,6.956775645154));
#62040=CARTESIAN_POINT('Ctrl Pts',(166.000248809185,32.6561147616383,4.94534548943256));
#62041=CARTESIAN_POINT('Ctrl Pts',(166.000445127974,34.1682512183075,0.514208821390161));
#62042=CARTESIAN_POINT('Ctrl Pts',(166.000316497984,33.3744506319377,-4.27334134716541));
#62043=CARTESIAN_POINT('Ctrl Pts',(166.000188622065,30.5620369933097,-6.9568350521799));
#62044=CARTESIAN_POINT('Ctrl Pts',(166.,28.9052030359509,-7.78899131169735));
#62045=CARTESIAN_POINT('Ctrl Pts',(166.,29.0148173223682,8.00939296706988));
#62046=CARTESIAN_POINT('Ctrl Pts',(166.,30.7185359819187,7.16206762906653));
#62047=CARTESIAN_POINT('Ctrl Pts',(166.,32.8805796900273,5.09922894584964));
#62048=CARTESIAN_POINT('Ctrl Pts',(166.,34.4460945651226,0.53120010524718));
#62049=CARTESIAN_POINT('Ctrl Pts',(166.,33.623029138765,-4.40994404024084));
#62050=CARTESIAN_POINT('Ctrl Pts',(166.,30.7184143629002,-7.16212811468035));
#62051=CARTESIAN_POINT('Ctrl Pts',(166.,29.0148173233401,-8.00939296658655));
#62052=CARTESIAN_POINT('',(164.848300728223,28.5746646574706,-7.12437716917367));
#62053=CARTESIAN_POINT('Ctrl Pts',(164.848300728223,28.5746646574706,7.12437716917368));
#62054=CARTESIAN_POINT('Ctrl Pts',(164.798268611131,30.1073707548339,6.3706789403067));
#62055=CARTESIAN_POINT('Ctrl Pts',(164.745477438776,32.0467280644762,4.53577823329202));
#62056=CARTESIAN_POINT('Ctrl Pts',(164.71073409437,33.4494761918939,0.472503961020967));
#62057=CARTESIAN_POINT('Ctrl Pts',(164.727959708039,32.7124405641852,-3.92265740596007));
#62058=CARTESIAN_POINT('Ctrl Pts',(164.798272182662,30.1072613429598,-6.37073274289246));
#62059=CARTESIAN_POINT('Ctrl Pts',(164.848300728223,28.5746646574706,-7.12437716917367));
#62060=CARTESIAN_POINT('',(166.,29.0148173233401,-8.00939296658655));
#62061=CARTESIAN_POINT('Origin',(165.,29.0148173233401,-8.00939296658655));
#62062=CARTESIAN_POINT('Ctrl Pts',(166.,29.0148173233401,-8.00939296658655));
#62063=CARTESIAN_POINT('Ctrl Pts',(166.,29.2779405522766,-7.87853158421673));
#62064=CARTESIAN_POINT('Ctrl Pts',(165.999999999834,29.5348160207278,-7.73518558482659));
#62065=CARTESIAN_POINT('Ctrl Pts',(166.000000000558,29.7844451870542,-7.58018506587251));
#62066=CARTESIAN_POINT('Ctrl Pts',(166.000000001295,30.0387454607129,-7.42228414841437));
#62067=CARTESIAN_POINT('Ctrl Pts',(166.000000003029,30.2855264780886,-7.25228806925218));
#62068=CARTESIAN_POINT('Ctrl Pts',(166.000000008263,30.5237126111613,-7.07102476511263));
#62069=CARTESIAN_POINT('Ctrl Pts',(166.000000013488,30.7615305489849,-6.89004166321052));
#62070=CARTESIAN_POINT('Ctrl Pts',(166.000000022271,30.9907808708886,-6.69782558012293));
#62071=CARTESIAN_POINT('Ctrl Pts',(166.000000037377,31.2103620662109,-6.49515910612427));
#62072=CARTESIAN_POINT('Ctrl Pts',(166.000000052225,31.4261910975295,-6.29595576041124));
#62073=CARTESIAN_POINT('Ctrl Pts',(166.000000073236,31.6326791969929,-6.08665551654678));
#62074=CARTESIAN_POINT('Ctrl Pts',(166.000000102371,31.8287411524828,-5.86797018386466));
#62075=CARTESIAN_POINT('Ctrl Pts',(166.000000107604,31.8639598400705,-5.82868764997117));
#62076=CARTESIAN_POINT('Ctrl Pts',(166.000000113097,31.8988419899412,-5.78910221730036));
#62077=CARTESIAN_POINT('Ctrl Pts',(166.000000118856,31.9333811531801,-5.74921792481992));
#62078=CARTESIAN_POINT('Ctrl Pts',(166.000000150119,32.1208901948591,-5.53269080720172));
#62079=CARTESIAN_POINT('Ctrl Pts',(166.000000203264,32.2983248359122,-5.30728279530615));
#62080=CARTESIAN_POINT('Ctrl Pts',(166.000000259834,32.4644907268496,-5.07385980318402));
#62081=CARTESIAN_POINT('Ctrl Pts',(166.00000031578,32.6288270671585,-4.84300688834743));
#62082=CARTESIAN_POINT('Ctrl Pts',(166.000000374415,32.7821409155448,-4.60431516859615));
#62083=CARTESIAN_POINT('Ctrl Pts',(166.000000422852,32.9233174446329,-4.35865268397587));
#62084=CARTESIAN_POINT('Ctrl Pts',(166.000000439074,32.9705981111956,-4.27637919207654));
#62085=CARTESIAN_POINT('Ctrl Pts',(166.000000454219,33.016517816017,-4.19332406369326));
#62086=CARTESIAN_POINT('Ctrl Pts',(166.000000467925,33.0610358659454,-4.10952048734535));
#62087=CARTESIAN_POINT('Ctrl Pts',(166.000000508826,33.1938876393192,-3.8594319558217));
#62088=CARTESIAN_POINT('Ctrl Pts',(166.000000538461,33.3142530323205,-3.60267716809763));
#62089=CARTESIAN_POINT('Ctrl Pts',(166.000000537731,33.4218645463685,-3.34071640263126));
#62090=CARTESIAN_POINT('Ctrl Pts',(166.000000537162,33.5059572485412,-3.13600793043694));
#62091=CARTESIAN_POINT('Ctrl Pts',(166.000000518585,33.5822626879903,-2.92812087607298));
#62092=CARTESIAN_POINT('Ctrl Pts',(166.000000455263,33.6506752218466,-2.71775448647747));
#62093=CARTESIAN_POINT('Ctrl Pts',(166.000000353886,33.7602003951459,-2.38096802385069));
#62094=CARTESIAN_POINT('Ctrl Pts',(166.000000250275,33.8494373207654,-2.03761856383257));
#62095=CARTESIAN_POINT('Ctrl Pts',(166.000000223102,33.9179520110566,-1.69019854210206));
#62096=CARTESIAN_POINT('Ctrl Pts',(166.00000019574,33.9869464827998,-1.34034567448453));
#62097=CARTESIAN_POINT('Ctrl Pts',(166.000000253222,34.0349275014748,-0.98636389626493));
#62098=CARTESIAN_POINT('Ctrl Pts',(166.000000400104,34.0613996253686,-0.630791481156381));
#62099=CARTESIAN_POINT('Ctrl Pts',(166.000000545298,34.0875676422193,-0.279303818604428));
#62100=CARTESIAN_POINT('Ctrl Pts',(166.000000786734,34.0927179512093,0.0737391630793566));
#62101=CARTESIAN_POINT('Ctrl Pts',(166.000000933819,34.0763223621711,0.42587626995759));
#62102=CARTESIAN_POINT('Ctrl Pts',(166.000000963239,34.0730429342587,0.496310351623806));
#62103=CARTESIAN_POINT('Ctrl Pts',(166.000000987998,34.0689013512222,0.566708133430982));
#62104=CARTESIAN_POINT('Ctrl Pts',(166.000001005107,34.0638931529613,0.637049820705425));
#62105=CARTESIAN_POINT('Ctrl Pts',(166.000001068865,34.045230072821,0.8991785301562));
#62106=CARTESIAN_POINT('Ctrl Pts',(166.000001002328,34.0147464243236,1.16038934196729));
#62107=CARTESIAN_POINT('Ctrl Pts',(166.000000968828,33.9722068619048,1.41967593394773));
#62108=CARTESIAN_POINT('Ctrl Pts',(166.000000925617,33.917336559996,1.7541206901679));
#62109=CARTESIAN_POINT('Ctrl Pts',(166.000000911493,33.8424085104102,2.0853658354223));
#62110=CARTESIAN_POINT('Ctrl Pts',(166.000000866665,33.7483792760101,2.41118811046363));
#62111=CARTESIAN_POINT('Ctrl Pts',(166.000000821343,33.6533159245128,2.74059372197889));
#62112=CARTESIAN_POINT('Ctrl Pts',(166.000000722415,33.5387277277513,3.06445673881697));
#62113=CARTESIAN_POINT('Ctrl Pts',(166.00000059145,33.405591800304,3.38042788805837));
#62114=CARTESIAN_POINT('Ctrl Pts',(166.00000052028,33.3332422910688,3.55213478955678));
#62115=CARTESIAN_POINT('Ctrl Pts',(166.000000444077,33.2554153371555,3.72151020748592));
#62116=CARTESIAN_POINT('Ctrl Pts',(166.000000386217,33.1722681870036,3.88817069316723));
#62117=CARTESIAN_POINT('Ctrl Pts',(166.00000036034,33.1350815110168,3.96270781764493));
#62118=CARTESIAN_POINT('Ctrl Pts',(166.000000335624,33.096831207137,4.03670871533531));
#62119=CARTESIAN_POINT('Ctrl Pts',(166.000000312295,33.0575332450514,4.110137780025));
#62120=CARTESIAN_POINT('Ctrl Pts',(166.00000021507,32.8937548398777,4.41616115808443));
#62121=CARTESIAN_POINT('Ctrl Pts',(166.000000143239,32.7117760742564,4.71225017109213));
#62122=CARTESIAN_POINT('Ctrl Pts',(166.00000009573,32.5133545836433,4.99691960166852));
#62123=CARTESIAN_POINT('Ctrl Pts',(166.000000045979,32.3055675195109,5.29502554293996));
#62124=CARTESIAN_POINT('Ctrl Pts',(166.000000022042,32.0797494852521,5.58060758080239));
#62125=CARTESIAN_POINT('Ctrl Pts',(166.000000010733,31.8379651039827,5.85199820701714));
#62126=CARTESIAN_POINT('Ctrl Pts',(165.999999999424,31.5961807227133,6.12338883323189));
#62127=CARTESIAN_POINT('Ctrl Pts',(166.,31.3384309655619,6.38058745243609));
#62128=CARTESIAN_POINT('Ctrl Pts',(166.,31.066813053308,6.62197450199632));
#62129=CARTESIAN_POINT('Ctrl Pts',(166.,30.6870642909768,6.95945752199541));
#62130=CARTESIAN_POINT('Ctrl Pts',(166.,30.27986428636,7.26635662931013));
#62131=CARTESIAN_POINT('Ctrl Pts',(166.,29.8504861606935,7.53837384064591));
#62132=CARTESIAN_POINT('Ctrl Pts',(166.,29.5802763661585,7.70955562749388));
#62133=CARTESIAN_POINT('Ctrl Pts',(166.,29.3012829815096,7.86692248927261));
#62134=CARTESIAN_POINT('Ctrl Pts',(166.,29.0148173223682,8.00939296706988));
#62135=CARTESIAN_POINT('Ctrl Pts',(150.052765342888,28.5386902386737,7.65589740253316));
#62136=CARTESIAN_POINT('Ctrl Pts',(151.463535576227,28.5393718199376,7.73398522097764));
#62137=CARTESIAN_POINT('Ctrl Pts',(154.303415022433,28.5469263529835,7.80605724763739));
#62138=CARTESIAN_POINT('Ctrl Pts',(159.273936712259,28.5392128490756,7.74348475067158));
#62139=CARTESIAN_POINT('Ctrl Pts',(162.799309686014,28.5326056052138,7.49650934344482));
#62140=CARTESIAN_POINT('Ctrl Pts',(164.848300728223,28.5746646574706,7.12437716917367));
#62141=CARTESIAN_POINT('Ctrl Pts',(150.041092860165,28.2301728106309,7.75403434833187));
#62142=CARTESIAN_POINT('Ctrl Pts',(151.45652206661,28.2200183619936,7.82609674557885));
#62143=CARTESIAN_POINT('Ctrl Pts',(154.30239251393,28.2148684396789,7.88948644418225));
#62144=CARTESIAN_POINT('Ctrl Pts',(159.281437973002,28.2182367984682,7.83463011613248));
#62145=CARTESIAN_POINT('Ctrl Pts',(162.820950710754,28.2486979386063,7.60855897109714));
#62146=CARTESIAN_POINT('Ctrl Pts',(164.886050420652,28.3206281744635,7.24424874059929));
#62147=CARTESIAN_POINT('Ctrl Pts',(150.020682003358,27.9774059754965,8.0111969323667));
#62148=CARTESIAN_POINT('Ctrl Pts',(151.443593918575,27.9553483654748,8.08775316583496));
#62149=CARTESIAN_POINT('Ctrl Pts',(154.30032819293,27.9354599116904,8.15604967867608));
#62150=CARTESIAN_POINT('Ctrl Pts',(159.295845511547,27.9520686413908,8.09687445201866));
#62151=CARTESIAN_POINT('Ctrl Pts',(162.857432768203,28.0234904089809,7.85599253660053));
#62152=CARTESIAN_POINT('Ctrl Pts',(164.942784454705,28.1247340937979,7.47571985177045));
#62153=CARTESIAN_POINT('Ctrl Pts',(149.999976847469,27.8849606552027,8.32099568908657));
#62154=CARTESIAN_POINT('Ctrl Pts',(151.43046103203,27.8596345886838,8.40586730719782));
#62155=CARTESIAN_POINT('Ctrl Pts',(154.298213256523,27.836322938964,8.48420051774229));
#62156=CARTESIAN_POINT('Ctrl Pts',(159.310547400486,27.8561240953706,8.41619209885521));
#62157=CARTESIAN_POINT('Ctrl Pts',(162.894363670138,27.9392205603659,8.14776095475912));
#62158=CARTESIAN_POINT('Ctrl Pts',(165.,28.05086990396,7.74330017699896));
#62159=CARTESIAN_POINT('',(150.,27.884960655152,8.32099568925641));
#62160=CARTESIAN_POINT('Ctrl Pts',(165.,28.05086990396,7.74330017699896));
#62161=CARTESIAN_POINT('Ctrl Pts',(162.894363670138,27.9392205603659,8.14776095475912));
#62162=CARTESIAN_POINT('Ctrl Pts',(159.310547400486,27.8561240953706,8.41619209885521));
#62163=CARTESIAN_POINT('Ctrl Pts',(154.298220953224,27.8363229693697,8.48420041331181));
#62164=CARTESIAN_POINT('Ctrl Pts',(151.430476444572,27.8596344633972,8.40586772819356));
#62165=CARTESIAN_POINT('Ctrl Pts',(149.999999911594,27.8849602468642,8.32099705749306));
#62166=CARTESIAN_POINT('',(150.052765342883,28.5386902383977,7.65589740262126));
#62167=CARTESIAN_POINT('Origin',(149.99997684747,28.843206725519,8.60694055822639));
#62168=CARTESIAN_POINT('Ctrl Pts',(150.052765342888,28.5386902386737,7.65589740253316));
#62169=CARTESIAN_POINT('Ctrl Pts',(151.463535576227,28.5393718199376,7.73398522097764));
#62170=CARTESIAN_POINT('Ctrl Pts',(154.303415022433,28.5469263529835,7.80605724763739));
#62171=CARTESIAN_POINT('Ctrl Pts',(159.273936712259,28.5392128490756,7.74348475067158));
#62172=CARTESIAN_POINT('Ctrl Pts',(162.799309686014,28.5326056052138,7.49650934344482));
#62173=CARTESIAN_POINT('Ctrl Pts',(164.848300728223,28.5746646574706,7.12437716917367));
#62174=CARTESIAN_POINT('Origin',(158.5,0.,0.));
#62175=CARTESIAN_POINT('',(150.,21.1486749637962,19.9885854245792));
#62176=CARTESIAN_POINT('Ctrl Pts',(150.,21.1486749637962,19.9885854245792));
#62177=CARTESIAN_POINT('Ctrl Pts',(152.860759052554,21.2703411716063,19.8598580019829));
#62178=CARTESIAN_POINT('Ctrl Pts',(157.882937220706,21.2859263327888,19.8416871554431));
#62179=CARTESIAN_POINT('Ctrl Pts',(162.893784247538,21.0258592764475,20.1221120335091));
#62180=CARTESIAN_POINT('Ctrl Pts',(165.,20.7313296143896,20.4211158465822));
#62181=CARTESIAN_POINT('Origin',(150.,0.,0.));
#62182=CARTESIAN_POINT('Ctrl Pts',(164.848300728217,-8.11744071408804,28.3085740825782));
#62183=CARTESIAN_POINT('Ctrl Pts',(162.79928054118,-7.77413038830263,28.4582180905047));
#62184=CARTESIAN_POINT('Ctrl Pts',(157.868876531342,-7.48949828735272,28.6380029652797));
#62185=CARTESIAN_POINT('Ctrl Pts',(152.874076231524,-7.50458485181733,28.6224409171841));
#62186=CARTESIAN_POINT('Ctrl Pts',(150.052788176347,-7.63914239096105,28.5431800801744));
#62187=CARTESIAN_POINT('Ctrl Pts',(164.886050420646,-7.88661064653829,28.1485078205187));
#62188=CARTESIAN_POINT('Ctrl Pts',(162.820921336791,-7.53513861487702,28.2683712291266));
#62189=CARTESIAN_POINT('Ctrl Pts',(157.870873056087,-7.25091052829838,28.3876462723107));
#62190=CARTESIAN_POINT('Ctrl Pts',(152.871720898814,-7.26493740471161,28.3795336075116));
#62191=CARTESIAN_POINT('Ctrl Pts',(150.041115769415,-7.39989458347469,28.3250644260708));
#62192=CARTESIAN_POINT('Ctrl Pts',(164.942784454699,-7.58820374368897,28.0945941257968));
#62193=CARTESIAN_POINT('Ctrl Pts',(162.857403106176,-7.20825069148137,28.1970523225311));
#62194=CARTESIAN_POINT('Ctrl Pts',(157.876626739393,-6.87707398921055,28.2763380277607));
#62195=CARTESIAN_POINT('Ctrl Pts',(152.866274197288,-6.89615963400192,28.2730907279766));
#62196=CARTESIAN_POINT('Ctrl Pts',(150.020705033617,-7.05080167669811,28.2347430874533));
#62197=CARTESIAN_POINT('Ctrl Pts',(164.999999999994,-7.31954028956917,28.1644160235815));
#62198=CARTESIAN_POINT('Ctrl Pts',(162.894333719583,-6.91343653306442,28.2699567457819));
#62199=CARTESIAN_POINT('Ctrl Pts',(157.882563753503,-6.54036960639615,28.3550152717686));
#62200=CARTESIAN_POINT('Ctrl Pts',(152.860712303346,-6.56397377534704,28.3505841327236));
#62201=CARTESIAN_POINT('Ctrl Pts',(150.,-6.73628528150281,28.3095824873171));
#62202=CARTESIAN_POINT('',(150.,-6.73628528150281,28.3095824873171));
#62203=CARTESIAN_POINT('Origin',(150.,-6.96777274822112,29.2824203734792));
#62204=CARTESIAN_POINT('',(164.999999999997,-7.31954028956918,28.1644160235815));
#62205=CARTESIAN_POINT('Ctrl Pts',(150.,-6.73628528150281,28.3095824873171));
#62206=CARTESIAN_POINT('Ctrl Pts',(152.860712303346,-6.56397377534704,28.3505841327236));
#62207=CARTESIAN_POINT('Ctrl Pts',(157.882563753503,-6.54036960639615,28.3550152717686));
#62208=CARTESIAN_POINT('Ctrl Pts',(162.894333719583,-6.91343653306442,28.2699567457819));
#62209=CARTESIAN_POINT('Ctrl Pts',(164.999999999994,-7.31954028956917,28.1644160235815));
#62210=CARTESIAN_POINT('',(164.948224876257,-7.57107088371366,28.1336066026404));
#62211=CARTESIAN_POINT('Origin',(164.999999999994,-7.57107088371244,29.1322653714709));
#62212=CARTESIAN_POINT('Origin',(164.999999999994,-7.57107088371244,29.1322653714709));
#62213=CARTESIAN_POINT('Ctrl Pts',(150.052788176357,-7.63914239116796,28.5431800803631));
#62214=CARTESIAN_POINT('Ctrl Pts',(146.270211473775,-7.81947858844008,28.4368505439217));
#62215=CARTESIAN_POINT('Ctrl Pts',(137.492178872596,-7.56977128393313,26.6032877773883));
#62216=CARTESIAN_POINT('Ctrl Pts',(130.307399870729,-5.92914147533666,21.3918099998411));
#62217=CARTESIAN_POINT('Ctrl Pts',(127.223161057304,-4.62069507309359,17.6980789259149));
#62218=CARTESIAN_POINT('Ctrl Pts',(150.041124530135,-7.39989439113668,28.3250648769978));
#62219=CARTESIAN_POINT('Ctrl Pts',(146.296085686373,-7.57964096967742,28.254623709958));
#62220=CARTESIAN_POINT('Ctrl Pts',(137.573627387529,-7.35172410484308,26.513206346242));
#62221=CARTESIAN_POINT('Ctrl Pts',(130.379397801599,-5.75870424283385,21.3658595958733));
#62222=CARTESIAN_POINT('Ctrl Pts',(127.284956078127,-4.47631553952171,17.6939861612586));
#62223=CARTESIAN_POINT('Ctrl Pts',(150.020722457357,-7.05080162839576,28.2347435757426));
#62224=CARTESIAN_POINT('Ctrl Pts',(146.304992405092,-7.25777004098844,28.1861302631782));
#62225=CARTESIAN_POINT('Ctrl Pts',(137.620797822779,-7.09907364073984,26.4971349531861));
#62226=CARTESIAN_POINT('Ctrl Pts',(130.42098757313,-5.57091977784276,21.3784706223794));
#62227=CARTESIAN_POINT('Ctrl Pts',(127.32129741028,-4.32046304628093,17.7152141200869));
#62228=CARTESIAN_POINT('Ctrl Pts',(150.000022383365,-6.73628528178715,28.3095824877733));
#62229=CARTESIAN_POINT('Ctrl Pts',(146.292010364484,-6.96723340941604,28.2545429014872));
#62230=CARTESIAN_POINT('Ctrl Pts',(137.621331204298,-6.86523720575822,26.555107107419));
#62231=CARTESIAN_POINT('Ctrl Pts',(130.426320557845,-5.39188507650232,21.4274847111616));
#62232=CARTESIAN_POINT('Ctrl Pts',(127.328278974586,-4.16988910307943,17.7594811554977));
#62233=CARTESIAN_POINT('',(128.0192689799,-4.43015359136868,18.5470144164462));
#62234=CARTESIAN_POINT('Ctrl Pts',(128.0192689799,-4.43015359136868,18.5470144164462));
#62235=CARTESIAN_POINT('Ctrl Pts',(131.026195153218,-5.51184022730075,21.8472743364665));
#62236=CARTESIAN_POINT('Ctrl Pts',(137.98124612881,-6.86946986657121,26.6256466535098));
#62237=CARTESIAN_POINT('Ctrl Pts',(146.291995471137,-6.96723323421941,28.2545399824182));
#62238=CARTESIAN_POINT('Ctrl Pts',(150.000000091398,-6.73628667020654,28.3095821568761));
#62239=CARTESIAN_POINT('Ctrl Pts',(128.0192689799,-4.43015359136868,18.5470144164462));
#62240=CARTESIAN_POINT('Ctrl Pts',(127.783727172056,-4.34542173861877,18.2884948708677));
#62241=CARTESIAN_POINT('Ctrl Pts',(127.55332925096,-4.25865825744875,18.0259350399143));
#62242=CARTESIAN_POINT('Ctrl Pts',(127.328278974586,-4.16988910307943,17.7594811554977));
#62243=CARTESIAN_POINT('Origin',(165.,-7.57107088371366,29.1322653714706));
#62244=CARTESIAN_POINT('',(166.,-7.57107088371365,29.1322653714706));
#62245=CARTESIAN_POINT('Origin',(165.,-7.57107088371366,29.1322653714706));
#62246=CARTESIAN_POINT('Origin',(165.,-7.57107088371366,29.1322653714706));
#62247=CARTESIAN_POINT('',(165.,-7.57107088371366,28.1322653714706));
#62248=CARTESIAN_POINT('Origin',(165.,-7.57107088371366,29.1322653714706));
#62249=CARTESIAN_POINT('Ctrl Pts',(120.9,0.,-4.94531715924951E-16));
#62250=CARTESIAN_POINT('Ctrl Pts',(120.9,4.94531715924951E-16,-4.94531715924951E-16));
#62251=CARTESIAN_POINT('Ctrl Pts',(120.9,4.94531715924951E-16,0.));
#62252=CARTESIAN_POINT('Ctrl Pts',(120.9,4.94531715924951E-16,4.94531715924951E-16));
#62253=CARTESIAN_POINT('Ctrl Pts',(120.9,0.,4.94531715924951E-16));
#62254=CARTESIAN_POINT('Ctrl Pts',(120.9,-4.94531715924951E-16,4.94531715924951E-16));
#62255=CARTESIAN_POINT('Ctrl Pts',(120.9,-4.94531715924951E-16,0.));
#62256=CARTESIAN_POINT('Ctrl Pts',(120.9,-4.94531715924951E-16,-4.94531715924951E-16));
#62257=CARTESIAN_POINT('Ctrl Pts',(120.9,0.,-4.94531715924951E-16));
#62258=CARTESIAN_POINT('Ctrl Pts',(120.90067372303,0.,29.0993263683664));
#62259=CARTESIAN_POINT('Ctrl Pts',(120.90067372303,-29.0993263683664,29.0993263683664));
#62260=CARTESIAN_POINT('Ctrl Pts',(120.90067372303,-29.0993263683664,0.));
#62261=CARTESIAN_POINT('Ctrl Pts',(120.90067372303,-29.0993263683664,-29.0993263683664));
#62262=CARTESIAN_POINT('Ctrl Pts',(120.90067372303,0.,-29.0993263683664));
#62263=CARTESIAN_POINT('Ctrl Pts',(120.90067372303,29.0993263683664,-29.0993263683664));
#62264=CARTESIAN_POINT('Ctrl Pts',(120.90067372303,29.0993263683664,0.));
#62265=CARTESIAN_POINT('Ctrl Pts',(120.90067372303,29.0993263683664,29.0993263683664));
#62266=CARTESIAN_POINT('Ctrl Pts',(120.90067372303,0.,29.0993263683664));
#62267=CARTESIAN_POINT('Ctrl Pts',(150.000000091398,0.,29.1000000000021));
#62268=CARTESIAN_POINT('Ctrl Pts',(150.000000091398,-29.1000000000021,29.1000000000021));
#62269=CARTESIAN_POINT('Ctrl Pts',(150.000000091398,-29.1000000000021,0.));
#62270=CARTESIAN_POINT('Ctrl Pts',(150.000000091398,-29.1000000000021,-29.1000000000021));
#62271=CARTESIAN_POINT('Ctrl Pts',(150.000000091398,0.,-29.1000000000021));
#62272=CARTESIAN_POINT('Ctrl Pts',(150.000000091398,29.1000000000021,-29.1000000000021));
#62273=CARTESIAN_POINT('Ctrl Pts',(150.000000091398,29.1000000000021,0.));
#62274=CARTESIAN_POINT('Ctrl Pts',(150.000000091398,29.1000000000021,29.1000000000021));
#62275=CARTESIAN_POINT('Ctrl Pts',(150.000000091398,0.,29.1000000000021));
#62276=CARTESIAN_POINT('',(120.9,1.27041389560989E-15,0.));
#62277=CARTESIAN_POINT('',(150.,-3.5637221855188E-15,29.1));
#62278=CARTESIAN_POINT('Origin',(150.000673754225,8.25110955088359E-20,
-0.000673754225024581));
#62279=CARTESIAN_POINT('Origin',(150.,0.,0.));
#62280=CARTESIAN_POINT('',(150.,-27.884960245299,8.32099706273789));
#62281=CARTESIAN_POINT('Origin',(150.,0.,0.));
#62282=CARTESIAN_POINT('',(128.01926933882,-18.2772621694713,5.43688145130374));
#62283=CARTESIAN_POINT('Ctrl Pts',(128.01926933882,-18.2772621694713,5.43688145130374));
#62284=CARTESIAN_POINT('Ctrl Pts',(131.026197307027,-21.6762107575019,6.15024132943591));
#62285=CARTESIAN_POINT('Ctrl Pts',(137.981270709504,-26.4931729493197,7.36366140502901));
#62286=CARTESIAN_POINT('Ctrl Pts',(146.291995471181,-27.9527660140403,8.09346901623637));
#62287=CARTESIAN_POINT('Ctrl Pts',(150.000000091398,-27.8849606534806,8.32099569486468));
#62288=CARTESIAN_POINT('',(127.328278974586,-17.4651063902315,5.26851068351907));
#62289=CARTESIAN_POINT('Ctrl Pts',(128.01926933882,-18.2772621694713,5.43688145130374));
#62290=CARTESIAN_POINT('Ctrl Pts',(127.783727340199,-18.0110119792102,5.38100175840513));
#62291=CARTESIAN_POINT('Ctrl Pts',(127.553329295421,-17.7402468546151,5.32486129410282));
#62292=CARTESIAN_POINT('Ctrl Pts',(127.328278974586,-17.4651063902317,5.26851068351816));
#62293=CARTESIAN_POINT('',(127.328278974586,-17.4651063902316,-5.26851068351812));
#62294=CARTESIAN_POINT('Ctrl Pts',(127.328278974586,-17.4651063902316,-5.26851068351812));
#62295=CARTESIAN_POINT('Ctrl Pts',(126.797908811484,-17.8243881888135,-1.79519278499075));
#62296=CARTESIAN_POINT('Ctrl Pts',(126.797908769232,-17.8243882174359,1.7951925082875));
#62297=CARTESIAN_POINT('Ctrl Pts',(127.328278974586,-17.4651063902315,5.26851068351907));
#62298=CARTESIAN_POINT('',(150.,-27.884960655152,-8.32099568925641));
#62299=CARTESIAN_POINT('Ctrl Pts',(150.,-27.884960655152,-8.32099568925641));
#62300=CARTESIAN_POINT('Ctrl Pts',(145.055988199056,-27.9753679280975,-8.01762643934787));
#62301=CARTESIAN_POINT('Ctrl Pts',(136.392549868564,-25.8653195043127,-7.16627842991105));
#62302=CARTESIAN_POINT('Ctrl Pts',(129.651808158315,-20.3057906258596,-5.85030184794966));
#62303=CARTESIAN_POINT('Ctrl Pts',(127.328278974586,-17.4651063902316,-5.26851068351812));
#62304=CARTESIAN_POINT('',(150.,-21.1486749637962,-19.9885854245792));
#62305=CARTESIAN_POINT('Origin',(150.,0.,0.));
#62306=CARTESIAN_POINT('',(128.019268748281,-13.8471090561928,-13.1101328489569));
#62307=CARTESIAN_POINT('Ctrl Pts',(128.019268748281,-13.8471090561928,-13.1101328489569));
#62308=CARTESIAN_POINT('Ctrl Pts',(131.026193763323,-16.1643769533533,-15.697032322276));
#62309=CARTESIAN_POINT('Ctrl Pts',(137.981230266414,-19.6237818841348,-19.2619772258016));
#62310=CARTESIAN_POINT('Ctrl Pts',(146.291995471109,-20.9855327799621,-20.1610709661675));
#62311=CARTESIAN_POINT('Ctrl Pts',(150.000000091398,-21.1486739832741,-19.9885864620114));
#62312=CARTESIAN_POINT('Ctrl Pts',(128.019268748281,-13.8471090561928,-13.1101328489569));
#62313=CARTESIAN_POINT('Ctrl Pts',(127.78372706355,-13.6655903346621,-12.9074930567686));
#62314=CARTESIAN_POINT('Ctrl Pts',(127.553329222269,-13.481588519049,-12.701073730158));
#62315=CARTESIAN_POINT('Ctrl Pts',(127.328278974586,-13.2952172871523,-12.4909704719795));
#62316=CARTESIAN_POINT('',(128.019268979856,-4.4301535913557,-18.5470144164053));
#62317=CARTESIAN_POINT('Ctrl Pts',(127.328278974584,-4.16988910307848,-17.7594811554948));
#62318=CARTESIAN_POINT('Ctrl Pts',(127.553329250947,-4.25865825744348,-18.0259350398984));
#62319=CARTESIAN_POINT('Ctrl Pts',(127.783727172029,-4.3454217386095,-18.2884948708391));
#62320=CARTESIAN_POINT('Ctrl Pts',(128.019268979856,-4.4301535913557,-18.5470144164053));
#62321=CARTESIAN_POINT('',(150.,-6.73628528150283,-28.3095824873171));
#62322=CARTESIAN_POINT('Ctrl Pts',(150.000000091398,-6.73628667020657,-28.3095821568761));
#62323=CARTESIAN_POINT('Ctrl Pts',(146.291995471133,-6.96723323421973,-28.2545399824181));
#62324=CARTESIAN_POINT('Ctrl Pts',(137.981246128019,-6.86946986660485,-26.6256466534606));
#62325=CARTESIAN_POINT('Ctrl Pts',(131.026195153116,-5.51184022729479,-21.8472743364333));
#62326=CARTESIAN_POINT('Ctrl Pts',(128.019268979856,-4.4301535913557,-18.5470144164053));
#62327=CARTESIAN_POINT('',(150.000000091398,6.73628667020652,-28.3095821568761));
#62328=CARTESIAN_POINT('Origin',(150.,0.,0.));
#62329=CARTESIAN_POINT('',(127.328278974586,4.16988910307942,-17.7594811554977));
#62330=CARTESIAN_POINT('Ctrl Pts',(127.328278974586,4.16988910307942,-17.7594811554977));
#62331=CARTESIAN_POINT('Ctrl Pts',(130.426320545001,5.39188507143624,-21.4274846959551));
#62332=CARTESIAN_POINT('Ctrl Pts',(137.621325010283,6.86523594041587,-26.5551027011384));
#62333=CARTESIAN_POINT('Ctrl Pts',(146.291995473394,6.96723323407881,-28.2545399824517));
#62334=CARTESIAN_POINT('Ctrl Pts',(150.000000091398,6.73628667020652,-28.3095821568761));
#62335=CARTESIAN_POINT('',(127.29181331856,13.0956191208171,-12.6347324681699));
#62336=CARTESIAN_POINT('Ctrl Pts',(127.29181331856,13.0956191208171,-12.6347324681699));
#62337=CARTESIAN_POINT('Ctrl Pts',(126.798200893053,10.3208848946384,-14.6228364954609));
#62338=CARTESIAN_POINT('Ctrl Pts',(126.810356111728,7.28270096923409,-16.3674248222649));
#62339=CARTESIAN_POINT('Ctrl Pts',(127.328278974586,4.16988910307852,-17.759481155498));
#62340=CARTESIAN_POINT('',(127.328278974581,13.2952172871479,-12.4909704719746));
#62341=CARTESIAN_POINT('Ctrl Pts',(127.29181331856,13.0956191208171,-12.6347324681699));
#62342=CARTESIAN_POINT('Ctrl Pts',(127.303676408344,13.1623048838804,-12.5869519518026));
#62343=CARTESIAN_POINT('Ctrl Pts',(127.31583162702,13.2288384796996,-12.5390307819704));
#62344=CARTESIAN_POINT('Ctrl Pts',(127.328278974586,13.295217287153,-12.4909704719789));
#62345=CARTESIAN_POINT('',(150.,21.1486749637962,-19.9885854245792));
#62346=CARTESIAN_POINT('Ctrl Pts',(150.000000091398,21.148673983274,-19.9885864620114));
#62347=CARTESIAN_POINT('Ctrl Pts',(146.291995471108,20.985532779962,-20.1610709661675));
#62348=CARTESIAN_POINT('Ctrl Pts',(137.621308523486,19.5648073199654,-19.2230393689233));
#62349=CARTESIAN_POINT('Ctrl Pts',(130.426320557839,15.8608035608144,-15.3832518061148));
#62350=CARTESIAN_POINT('Ctrl Pts',(127.328278974581,13.2952172871479,-12.4909704719746));
#62351=CARTESIAN_POINT('',(150.,27.884960245299,-8.32099706273788));
#62352=CARTESIAN_POINT('Origin',(150.,0.,0.));
#62353=CARTESIAN_POINT('',(128.019269338873,18.2772621694247,-5.43688145130243));
#62354=CARTESIAN_POINT('Ctrl Pts',(128.019269338873,18.2772621694247,-5.43688145130243));
#62355=CARTESIAN_POINT('Ctrl Pts',(131.026197296283,21.6762107444127,-6.15024132676383));
#62356=CARTESIAN_POINT('Ctrl Pts',(137.981270696745,26.4931729473759,-7.36366140391153));
#62357=CARTESIAN_POINT('Ctrl Pts',(146.29199547345,27.9527660139988,-8.0934690163756));
#62358=CARTESIAN_POINT('Ctrl Pts',(150.000000091398,27.8849606534806,-8.32099569486468));
#62359=CARTESIAN_POINT('',(127.328278974586,17.4651063902315,-5.26851068351906));
#62360=CARTESIAN_POINT('Ctrl Pts',(128.019269338873,18.2772621694247,-5.43688145130243));
#62361=CARTESIAN_POINT('Ctrl Pts',(127.783727340134,18.0110119790964,-5.38100175838451));
#62362=CARTESIAN_POINT('Ctrl Pts',(127.553329295338,17.7402468545128,-5.32486129408186));
#62363=CARTESIAN_POINT('Ctrl Pts',(127.328278974586,17.4651063902317,-5.26851068351815));
#62364=CARTESIAN_POINT('',(127.328278974586,17.4651063902316,5.26851068351812));
#62365=CARTESIAN_POINT('Ctrl Pts',(127.328278974586,17.4651063902316,5.26851068351812));
#62366=CARTESIAN_POINT('Ctrl Pts',(126.797908811472,17.8243881888213,1.79519278491536));
#62367=CARTESIAN_POINT('Ctrl Pts',(126.797908769233,17.8243882174352,-1.79519250829358));
#62368=CARTESIAN_POINT('Ctrl Pts',(127.328278974586,17.4651063902315,-5.26851068351905));
#62369=CARTESIAN_POINT('Ctrl Pts',(150.,27.884960655152,8.32099568925642));
#62370=CARTESIAN_POINT('Ctrl Pts',(145.055988202077,27.9753679280423,8.01762643953326));
#62371=CARTESIAN_POINT('Ctrl Pts',(136.392549858192,25.8653195016249,7.16627842882971));
#62372=CARTESIAN_POINT('Ctrl Pts',(129.65180814865,20.3057906140435,5.85030184552965));
#62373=CARTESIAN_POINT('Ctrl Pts',(127.328278974586,17.4651063902316,5.26851068351813));
#62374=CARTESIAN_POINT('',(127.328278974586,13.2952172871523,12.4909704719795));
#62375=CARTESIAN_POINT('Ctrl Pts',(127.328278974586,13.2952172871523,12.4909704719795));
#62376=CARTESIAN_POINT('Ctrl Pts',(130.426320545001,15.8608035501812,15.3832517941273));
#62377=CARTESIAN_POINT('Ctrl Pts',(137.621308508834,19.5648073178329,19.2230393677456));
#62378=CARTESIAN_POINT('Ctrl Pts',(146.291995473366,20.9855327800614,20.1610709660625));
#62379=CARTESIAN_POINT('Ctrl Pts',(150.000000091398,21.1486739832741,19.9885864620114));
#62380=CARTESIAN_POINT('',(127.328278974586,4.16988910307941,17.7594811554976));
#62381=CARTESIAN_POINT('Ctrl Pts',(127.328278974586,4.1698891030794,17.7594811554976));
#62382=CARTESIAN_POINT('Ctrl Pts',(126.797908763857,7.35751182416156,16.3339692429127));
#62383=CARTESIAN_POINT('Ctrl Pts',(126.797908763857,10.4668763969161,14.5387767698241));
#62384=CARTESIAN_POINT('Ctrl Pts',(127.328278974586,13.295217287153,12.4909704719789));
#62385=CARTESIAN_POINT('',(150.,6.73628667589916,28.3095821555194));
#62386=CARTESIAN_POINT('Ctrl Pts',(150.,6.73628667589916,28.3095821555194));
#62387=CARTESIAN_POINT('Ctrl Pts',(145.055988202065,7.0442157893323,28.2361925256675));
#62388=CARTESIAN_POINT('Ctrl Pts',(136.392518944088,6.72647599839076,25.9832187747262));
#62389=CARTESIAN_POINT('Ctrl Pts',(129.651808148682,5.08638528899869,20.510481438492));
#62390=CARTESIAN_POINT('Ctrl Pts',(127.328278974586,4.1698891030794,17.7594811554976));
#62391=CARTESIAN_POINT('Origin',(150.,0.,0.));
#62392=CARTESIAN_POINT('Ctrl Pts',(127.110025063046,14.1660632471973,13.6372179765762));
#62393=CARTESIAN_POINT('Ctrl Pts',(126.561429493857,11.2405277823209,15.7553971673589));
#62394=CARTESIAN_POINT('Ctrl Pts',(126.561429493857,8.02431030248663,17.6122811951136));
#62395=CARTESIAN_POINT('Ctrl Pts',(127.110025063046,4.72714558106307,19.0867796319776));
#62396=CARTESIAN_POINT('Ctrl Pts',(127.362931194533,14.0316094882686,13.5170175430695));
#62397=CARTESIAN_POINT('Ctrl Pts',(126.820035970083,11.1364717038076,15.6131877334421));
#62398=CARTESIAN_POINT('Ctrl Pts',(126.820035970083,7.95318135931358,17.4510612707445));
#62399=CARTESIAN_POINT('Ctrl Pts',(127.362931194533,4.69027583156468,18.9102390443577));
#62400=CARTESIAN_POINT('Ctrl Pts',(127.647216190801,13.68668967427,13.1142576336319));
#62401=CARTESIAN_POINT('Ctrl Pts',(127.114082771185,10.8436088537942,15.1727363627013));
#62402=CARTESIAN_POINT('Ctrl Pts',(127.114082771185,7.71817070812703,16.9772089174379));
#62403=CARTESIAN_POINT('Ctrl Pts',(127.647216190801,4.51393542536509,18.4101497684475));
#62404=CARTESIAN_POINT('Ctrl Pts',(127.47007422846,13.3854383233912,12.6523038901745));
#62405=CARTESIAN_POINT('Ctrl Pts',(126.93997655279,10.5585493016116,14.6990589472656));
#62406=CARTESIAN_POINT('Ctrl Pts',(126.93997655279,7.45048380925201,16.4935013959384));
#62407=CARTESIAN_POINT('Ctrl Pts',(127.47007422846,4.26449742359709,17.9182815739334));
#62408=CARTESIAN_POINT('Ctrl Pts',(127.328278974586,13.295217287153,12.4909704719789));
#62409=CARTESIAN_POINT('Ctrl Pts',(126.797908763857,10.4668763969161,14.5387767698241));
#62410=CARTESIAN_POINT('Ctrl Pts',(126.797908763857,7.35751182416156,16.3339692429127));
#62411=CARTESIAN_POINT('Ctrl Pts',(127.328278974586,4.1698891030794,17.7594811554976));
#62412=CARTESIAN_POINT('',(127.464921070561,13.2136059641945,13.0809596303012));
#62413=CARTESIAN_POINT('Ctrl Pts',(127.328278974586,13.295217287153,12.4909704719789));
#62414=CARTESIAN_POINT('Ctrl Pts',(127.328985683102,13.2947964472831,12.4927011093439));
#62415=CARTESIAN_POINT('Ctrl Pts',(127.329689950248,13.2943770553819,12.4944330979285));
#62416=CARTESIAN_POINT('Ctrl Pts',(127.404564207147,13.2497887223447,12.679354422203));
#62417=CARTESIAN_POINT('Ctrl Pts',(127.452250527053,13.2213365014775,12.87955910642));
#62418=CARTESIAN_POINT('Ctrl Pts',(127.464921070561,13.2136059641945,13.0809596303012));
#62419=CARTESIAN_POINT('',(126.797085404885,11.8793261399438,15.2022528231739));
#62420=CARTESIAN_POINT('Ctrl Pts',(127.464921070561,13.2136059641945,13.0809596303012));
#62421=CARTESIAN_POINT('Ctrl Pts',(127.468732908105,13.2112802903014,13.1415494603879));
#62422=CARTESIAN_POINT('Ctrl Pts',(127.468147645086,13.2041296276702,13.2063365920774));
#62423=CARTESIAN_POINT('Ctrl Pts',(127.449450455234,13.157374753389,13.4631550642539));
#62424=CARTESIAN_POINT('Ctrl Pts',(127.402566273023,13.0839127203925,13.6767330303382));
#62425=CARTESIAN_POINT('Ctrl Pts',(127.213715884126,12.7703267036052,14.2701257571167));
#62426=CARTESIAN_POINT('Ctrl Pts',(127.0433252609,12.4761107319414,14.6464349243858));
#62427=CARTESIAN_POINT('Ctrl Pts',(126.846608678515,12.0058525467556,15.0894641383699));
#62428=CARTESIAN_POINT('Ctrl Pts',(126.821477307792,11.9431296392106,15.1463361069293));
#62429=CARTESIAN_POINT('Ctrl Pts',(126.797085404885,11.8793261399438,15.2022528231739));
#62430=CARTESIAN_POINT('',(126.797085404885,7.22587406965037,17.8889246286188));
#62431=CARTESIAN_POINT('Ctrl Pts',(126.797739711379,11.8790433321593,15.201904292993));
#62432=CARTESIAN_POINT('Ctrl Pts',(126.665524611079,10.3768517946564,16.1726158137204));
#62433=CARTESIAN_POINT('Ctrl Pts',(126.665524611079,8.81747024299962,17.0729251723388));
#62434=CARTESIAN_POINT('Ctrl Pts',(126.797739711379,7.22571363755198,17.8885054448026));
#62435=CARTESIAN_POINT('',(127.464921070561,4.72164036362229,17.9837982557406));
#62436=CARTESIAN_POINT('Ctrl Pts',(126.797085404885,7.22587406965035,17.8889246286188));
#62437=CARTESIAN_POINT('Ctrl Pts',(126.91366853489,6.84194426602849,18.0193933569079));
#62438=CARTESIAN_POINT('Ctrl Pts',(127.036712870258,6.48459473410042,18.1063632325042));
#62439=CARTESIAN_POINT('Ctrl Pts',(127.242195869014,5.86018690005478,18.1870904290044));
#62440=CARTESIAN_POINT('Ctrl Pts',(127.32299954319,5.60156722060403,18.1899973333732));
#62441=CARTESIAN_POINT('Ctrl Pts',(127.427486401576,5.18000926912787,18.1447123913596));
#62442=CARTESIAN_POINT('Ctrl Pts',(127.456769053802,5.01340235795799,18.1047856321497));
#62443=CARTESIAN_POINT('Ctrl Pts',(127.468025475808,4.82171990225562,18.0321668235628));
#62444=CARTESIAN_POINT('Ctrl Pts',(127.468398488078,4.77057001346659,18.0095979457834));
#62445=CARTESIAN_POINT('Ctrl Pts',(127.464921070561,4.7216403636223,17.9837982557406));
#62446=CARTESIAN_POINT('Ctrl Pts',(127.464921070561,4.72164036362229,17.9837982557406));
#62447=CARTESIAN_POINT('Ctrl Pts',(127.452250527053,4.54335712496464,17.8897928354722));
#62448=CARTESIAN_POINT('Ctrl Pts',(127.404564207145,4.35574867204235,17.8143308394271));
#62449=CARTESIAN_POINT('Ctrl Pts',(127.329689950249,4.17330794100252,17.7604848064147));
#62450=CARTESIAN_POINT('Ctrl Pts',(127.328985683102,4.17159829893694,17.7599820161618));
#62451=CARTESIAN_POINT('Ctrl Pts',(127.328278974586,4.1698891030794,17.7594811554976));
#62452=CARTESIAN_POINT('Ctrl Pts',(164.848300728223,8.11744071408904,28.3085740825778));
#62453=CARTESIAN_POINT('Ctrl Pts',(164.798272182631,9.53641427628355,29.2590195334092));
#62454=CARTESIAN_POINT('Ctrl Pts',(164.745477688401,12.0952706508999,30.0211439647892));
#62455=CARTESIAN_POINT('Ctrl Pts',(164.710734443168,16.315539691088,29.2043188966142));
#62456=CARTESIAN_POINT('Ctrl Pts',(164.727960074229,19.7533321894811,26.3684531320398));
#62457=CARTESIAN_POINT('Ctrl Pts',(164.798268611372,20.5708551807295,22.8884084339971));
#62458=CARTESIAN_POINT('Ctrl Pts',(164.848300728574,20.4572239425854,21.1841969014631));
#62459=CARTESIAN_POINT('Ctrl Pts',(165.010504706333,8.13120148533914,28.2878287434741));
#62460=CARTESIAN_POINT('Ctrl Pts',(164.963974112446,9.55100409550378,29.2280639246229));
#62461=CARTESIAN_POINT('Ctrl Pts',(164.913918487071,12.100253465697,29.9750124490936));
#62462=CARTESIAN_POINT('Ctrl Pts',(164.880672746118,16.2919170078553,29.1558227187027));
#62463=CARTESIAN_POINT('Ctrl Pts',(164.897255418794,19.7077886489462,26.3436868844839));
#62464=CARTESIAN_POINT('Ctrl Pts',(164.963970790889,20.5367512667223,22.8855654705432));
#62465=CARTESIAN_POINT('Ctrl Pts',(165.010504706659,20.4323775663511,21.1857414094199));
#62466=CARTESIAN_POINT('Ctrl Pts',(165.346643666359,8.1134843469509,28.3145385867765));
#62467=CARTESIAN_POINT('Ctrl Pts',(165.311964088936,9.54605673078314,29.2469419456448));
#62468=CARTESIAN_POINT('Ctrl Pts',(165.273525810695,12.1026828348789,29.9768978845671));
#62469=CARTESIAN_POINT('Ctrl Pts',(165.247690695636,16.2881769576474,29.1462143071605));
#62470=CARTESIAN_POINT('Ctrl Pts',(165.260682170683,19.701605365211,26.3451428070365));
#62471=CARTESIAN_POINT('Ctrl Pts',(165.311961613361,20.5555728549281,22.8907204474521));
#62472=CARTESIAN_POINT('Ctrl Pts',(165.346643666603,20.4643675384684,21.1837528390945));
#62473=CARTESIAN_POINT('Ctrl Pts',(165.840925930751,7.93271062991558,28.5870677926451));
#62474=CARTESIAN_POINT('Ctrl Pts',(165.831141148134,9.42128698274788,29.551697143448));
#62475=CARTESIAN_POINT('Ctrl Pts',(165.819968147143,12.0798299978231,30.3050779710485));
#62476=CARTESIAN_POINT('Ctrl Pts',(165.812321983518,16.4337788939504,29.4362498950202));
#62477=CARTESIAN_POINT('Ctrl Pts',(165.816207843869,19.9872703168054,26.5233751293306));
#62478=CARTESIAN_POINT('Ctrl Pts',(165.831140449655,20.8818834655985,22.9350488872553));
#62479=CARTESIAN_POINT('Ctrl Pts',(165.84092593082,20.7907716125423,21.1634628102871));
#62480=CARTESIAN_POINT('Ctrl Pts',(166.,7.70713717218928,28.9271357865293));
#62481=CARTESIAN_POINT('Ctrl Pts',(166.000188622065,9.25622261247859,29.9459179543204));
#62482=CARTESIAN_POINT('Ctrl Pts',(166.000254403677,12.045266137773,30.7536647731228));
#62483=CARTESIAN_POINT('Ctrl Pts',(166.000449856426,16.6388072410634,29.8476424898111));
#62484=CARTESIAN_POINT('Ctrl Pts',(166.000322616219,20.3880342485358,26.7664214513262));
#62485=CARTESIAN_POINT('Ctrl Pts',(166.000188635531,21.3058220758124,22.9892150281585));
#62486=CARTESIAN_POINT('Ctrl Pts',(166.,21.1980658630061,21.1381444618613));
#62487=CARTESIAN_POINT('Ctrl Pts',(166.,7.57107088371366,29.1322653714706));
#62488=CARTESIAN_POINT('Ctrl Pts',(166.,9.15662228995011,30.1839912602332));
#62489=CARTESIAN_POINT('Ctrl Pts',(166.,12.0242343247742,31.0250024159159));
#62490=CARTESIAN_POINT('Ctrl Pts',(166.,16.7630166327018,30.0967599181513));
#62491=CARTESIAN_POINT('Ctrl Pts',(166.,20.6306277104266,26.9133994060884));
#62492=CARTESIAN_POINT('Ctrl Pts',(166.,21.5618005030748,23.0219987016644));
#62493=CARTESIAN_POINT('Ctrl Pts',(166.,21.4437464387992,21.1228723915773));
#62494=CARTESIAN_POINT('',(166.,7.57107088371367,29.1322653714706));
#62495=CARTESIAN_POINT('Ctrl Pts',(166.,21.4437464387992,21.1228723915773));
#62496=CARTESIAN_POINT('Ctrl Pts',(166.,21.4621686307353,21.4192287229753));
#62497=CARTESIAN_POINT('Ctrl Pts',(166.,21.4663647218671,21.7164281670279));
#62498=CARTESIAN_POINT('Ctrl Pts',(166.,21.4565635257071,22.0131479146322));
#62499=CARTESIAN_POINT('Ctrl Pts',(166.,21.4466079928545,22.3145400250508));
#62500=CARTESIAN_POINT('Ctrl Pts',(166.,21.4222109065277,22.6154380858716));
#62501=CARTESIAN_POINT('Ctrl Pts',(166.,21.3835590222112,22.914464494951));
#62502=CARTESIAN_POINT('Ctrl Pts',(166.,21.3541085048082,23.1423054558845));
#62503=CARTESIAN_POINT('Ctrl Pts',(166.,21.3163811755797,23.3690601001961));
#62504=CARTESIAN_POINT('Ctrl Pts',(166.,21.2704394020836,23.5941175144741));
#62505=CARTESIAN_POINT('Ctrl Pts',(166.,21.2092887413406,23.8936795152614));
#62506=CARTESIAN_POINT('Ctrl Pts',(166.000000182997,21.1333324966942,24.1904004508523));
#62507=CARTESIAN_POINT('Ctrl Pts',(166.000000315222,21.0428321916662,24.4826093434109));
#62508=CARTESIAN_POINT('Ctrl Pts',(166.00000044687,20.9527260420472,24.7735455804189));
#62509=CARTESIAN_POINT('Ctrl Pts',(166.000000481393,20.8482033305631,25.0600085816412));
#62510=CARTESIAN_POINT('Ctrl Pts',(166.000000403152,20.7295399477617,25.3403974056223));
#62511=CARTESIAN_POINT('Ctrl Pts',(166.000000325642,20.6119849291697,25.6181672840627));
#62512=CARTESIAN_POINT('Ctrl Pts',(166.000000173335,20.480553262582,25.8899758742135));
#62513=CARTESIAN_POINT('Ctrl Pts',(166.000000221777,20.3355143928098,26.1543175082492));
#62514=CARTESIAN_POINT('Ctrl Pts',(166.000000247965,20.257101679808,26.2972291616328));
#62515=CARTESIAN_POINT('Ctrl Pts',(166.000000336743,20.17471173203,26.4379592383969));
#62516=CARTESIAN_POINT('Ctrl Pts',(166.000000457868,20.0883855303905,26.5762759943601));
#62517=CARTESIAN_POINT('Ctrl Pts',(166.0000005192,20.0446736960014,26.6463135845133));
#62518=CARTESIAN_POINT('Ctrl Pts',(166.000000587215,19.9999525905503,26.7157324739482));
#62519=CARTESIAN_POINT('Ctrl Pts',(166.000000643046,19.9542491979835,26.7845126653514));
#62520=CARTESIAN_POINT('Ctrl Pts',(166.000000883843,19.7571309572189,27.081160891389));
#62521=CARTESIAN_POINT('Ctrl Pts',(166.000000697529,19.5414571535571,27.3652951332236));
#62522=CARTESIAN_POINT('Ctrl Pts',(166.000000530134,19.3093359639014,27.6352769313963));
#62523=CARTESIAN_POINT('Ctrl Pts',(166.000000361028,19.0748423996141,27.9080180552897));
#62524=CARTESIAN_POINT('Ctrl Pts',(166.000000192139,18.8235635193579,28.1663167108179));
#62525=CARTESIAN_POINT('Ctrl Pts',(166.000000105436,18.5576199011917,28.4084907649282));
#62526=CARTESIAN_POINT('Ctrl Pts',(166.000000017884,18.2890717748359,28.653036540953));
#62527=CARTESIAN_POINT('Ctrl Pts',(166.000000001753,18.0055701089825,28.8811412702077));
#62528=CARTESIAN_POINT('Ctrl Pts',(166.000000000218,17.709246017533,29.0910674138255));
#62529=CARTESIAN_POINT('Ctrl Pts',(166.,17.6671352503958,29.1209001247152));
#62530=CARTESIAN_POINT('Ctrl Pts',(166.,17.6247654464966,29.1503656887051));
#62531=CARTESIAN_POINT('Ctrl Pts',(166.,17.5821426410779,29.1794590922125));
#62532=CARTESIAN_POINT('Ctrl Pts',(166.,17.3227076772513,29.3565437775678));
#62533=CARTESIAN_POINT('Ctrl Pts',(166.000000199173,17.0537093426507,29.5198118647934));
#62534=CARTESIAN_POINT('Ctrl Pts',(166.00000039802,16.776662920222,29.6680605547367));
#62535=CARTESIAN_POINT('Ctrl Pts',(166.000000596805,16.499702213626,29.8162633777823));
#62536=CARTESIAN_POINT('Ctrl Pts',(166.00000077823,16.2146992805161,29.9494563134435));
#62537=CARTESIAN_POINT('Ctrl Pts',(166.000000858664,15.9231554041651,30.0664880534137));
#62538=CARTESIAN_POINT('Ctrl Pts',(166.000000873894,15.8679556353844,30.0886463819206));
#62539=CARTESIAN_POINT('Ctrl Pts',(166.000000886098,15.8125213282913,30.1102255003819));
#62540=CARTESIAN_POINT('Ctrl Pts',(166.000000895473,15.7568625837656,30.1312177854691));
#62541=CARTESIAN_POINT('Ctrl Pts',(166.000000945381,15.46058885506,30.2429605606578));
#62542=CARTESIAN_POINT('Ctrl Pts',(166.000000921655,15.1579584946294,30.3380723749196));
#62543=CARTESIAN_POINT('Ctrl Pts',(166.000000860768,14.8510970562341,30.4164678512046));
#62544=CARTESIAN_POINT('Ctrl Pts',(166.000000835849,14.7255066155903,30.448553089619));
#62545=CARTESIAN_POINT('Ctrl Pts',(166.000000803469,14.5992070393624,30.4778387046225));
#62546=CARTESIAN_POINT('Ctrl Pts',(166.000000748424,14.4723421877687,30.5043205455331));
#62547=CARTESIAN_POINT('Ctrl Pts',(166.000000591922,14.1116427516536,30.5796131499363));
#62548=CARTESIAN_POINT('Ctrl Pts',(166.000000407613,13.745908175493,30.631983158851));
#62549=CARTESIAN_POINT('Ctrl Pts',(166.000000281907,13.3784662732673,30.6610967056782));
#62550=CARTESIAN_POINT('Ctrl Pts',(166.000000235305,13.2422491376513,30.6718896063583));
#62551=CARTESIAN_POINT('Ctrl Pts',(166.000000195175,13.1057974421341,30.6794868558029));
#62552=CARTESIAN_POINT('Ctrl Pts',(166.000000161682,12.969280832816,30.6838732411217));
#62553=CARTESIAN_POINT('Ctrl Pts',(166.000000069129,12.5920454553611,30.6959941085357));
#62554=CARTESIAN_POINT('Ctrl Pts',(166.000000028569,12.214315574293,30.6835936914797));
#62555=CARTESIAN_POINT('Ctrl Pts',(166.000000012119,11.8388348293787,30.6477178836999));
#62556=CARTESIAN_POINT('Ctrl Pts',(165.999999999626,11.5536816128353,30.6204725399025));
#62557=CARTESIAN_POINT('Ctrl Pts',(166.,11.2698254594428,30.5796891992455));
#62558=CARTESIAN_POINT('Ctrl Pts',(166.,10.9884598690122,30.5258441976976));
#62559=CARTESIAN_POINT('Ctrl Pts',(166.,10.5780587367051,30.4473056330829));
#62560=CARTESIAN_POINT('Ctrl Pts',(166.,10.1729585399023,30.3409857422123));
#62561=CARTESIAN_POINT('Ctrl Pts',(166.,9.77663239436923,30.2082790684448));
#62562=CARTESIAN_POINT('Ctrl Pts',(166.,9.37915096488819,30.0751855569888));
#62563=CARTESIAN_POINT('Ctrl Pts',(166.,8.99049371169764,29.9155508029567));
#62564=CARTESIAN_POINT('Ctrl Pts',(166.,8.61417539414345,29.7307310367179));
#62565=CARTESIAN_POINT('Ctrl Pts',(166.,8.25414706838941,29.5539117114253));
#62566=CARTESIAN_POINT('Ctrl Pts',(166.,7.90541178106159,29.3540399389995));
#62567=CARTESIAN_POINT('Ctrl Pts',(166.,7.57107088371366,29.1322653714706));
#62568=CARTESIAN_POINT('',(164.848300728756,8.11744071417838,28.3085740825388));
#62569=CARTESIAN_POINT('Origin',(165.,7.57107088371367,29.1322653714706));
#62570=CARTESIAN_POINT('Ctrl Pts',(164.848300728223,8.11744071408904,28.3085740825778));
#62571=CARTESIAN_POINT('Ctrl Pts',(164.798272182631,9.53641427628355,29.2590195334092));
#62572=CARTESIAN_POINT('Ctrl Pts',(164.745477688401,12.0952706508999,30.0211439647892));
#62573=CARTESIAN_POINT('Ctrl Pts',(164.710734443168,16.315539691088,29.2043188966142));
#62574=CARTESIAN_POINT('Ctrl Pts',(164.727960074212,19.7533321862694,26.3684531346892));
#62575=CARTESIAN_POINT('Ctrl Pts',(164.798268611208,20.5708551788201,22.8884084421251));
#62576=CARTESIAN_POINT('Ctrl Pts',(164.848300728223,20.4572239433816,21.1841969134041));
#62577=CARTESIAN_POINT('Ctrl Pts',(164.848300728223,20.4572239433816,21.1841969134041));
#62578=CARTESIAN_POINT('Ctrl Pts',(162.798745850892,20.7585532298029,20.9616453943524));
#62579=CARTESIAN_POINT('Ctrl Pts',(157.869241198012,21.056434491268,20.8051355149715));
#62580=CARTESIAN_POINT('Ctrl Pts',(152.874122336469,21.0354707478812,20.8103803284396));
#62581=CARTESIAN_POINT('Ctrl Pts',(150.052788176347,20.8995478587445,20.8872814137861));
#62582=CARTESIAN_POINT('Ctrl Pts',(164.886050420652,20.4340175279241,20.904259079919));
#62583=CARTESIAN_POINT('Ctrl Pts',(162.820382442898,20.7136312465506,20.6597432865156));
#62584=CARTESIAN_POINT('Ctrl Pts',(157.871240162951,20.9589192079952,20.4733382920777));
#62585=CARTESIAN_POINT('Ctrl Pts',(152.871767156017,20.9449302228963,20.4813856882316));
#62586=CARTESIAN_POINT('Ctrl Pts',(150.041115769415,20.8302780650708,20.5710289076513));
#62587=CARTESIAN_POINT('Ctrl Pts',(164.942784454705,20.5365303501078,20.618874274026));
#62588=CARTESIAN_POINT('Ctrl Pts',(162.856858927469,20.8153110060362,20.34098188004));
#62589=CARTESIAN_POINT('Ctrl Pts',(157.876997023201,21.0494420975234,20.0939392476401));
#62590=CARTESIAN_POINT('Ctrl Pts',(152.86632069903,21.0371368032061,20.1087929203625));
#62591=CARTESIAN_POINT('Ctrl Pts',(150.020705033617,20.9266039447126,20.2235449127931));
#62592=CARTESIAN_POINT('Ctrl Pts',(165.,20.7313296143896,20.4211158465822));
#62593=CARTESIAN_POINT('Ctrl Pts',(162.893784247538,21.0258592764475,20.1221120335091));
#62594=CARTESIAN_POINT('Ctrl Pts',(157.882937220706,21.2859263327888,19.8416871554431));
#62595=CARTESIAN_POINT('Ctrl Pts',(152.860759052554,21.2703411716063,19.8598580019829));
#62596=CARTESIAN_POINT('Ctrl Pts',(150.,21.1486749637962,19.9885854245792));
#62597=CARTESIAN_POINT('',(150.052788176347,20.8995478587445,20.8872814137861));
#62598=CARTESIAN_POINT('Ctrl Pts',(164.848300728223,20.4572239433816,21.1841969134041));
#62599=CARTESIAN_POINT('Ctrl Pts',(162.798745850892,20.7585532298029,20.9616453943524));
#62600=CARTESIAN_POINT('Ctrl Pts',(157.869241198012,21.056434491268,20.8051355149715));
#62601=CARTESIAN_POINT('Ctrl Pts',(152.874122336469,21.0354707478812,20.8103803284396));
#62602=CARTESIAN_POINT('Ctrl Pts',(150.052788176347,20.8995478587445,20.8872814137861));
#62603=CARTESIAN_POINT('Origin',(150.,21.8754335536174,20.675478394496));
#62604=CARTESIAN_POINT('Ctrl Pts',(150.052788176357,20.8995478588044,20.8872814140596));
#62605=CARTESIAN_POINT('Ctrl Pts',(146.270211476078,20.7172956805484,20.9902923738357));
#62606=CARTESIAN_POINT('Ctrl Pts',(137.492160023873,19.2542660925959,19.8572749780016));
#62607=CARTESIAN_POINT('Ctrl Pts',(130.307399857943,15.5612801445746,15.8306921278397));
#62608=CARTESIAN_POINT('Ctrl Pts',(127.223161057304,13.0166384114775,12.8506787793981));
#62609=CARTESIAN_POINT('Ctrl Pts',(150.041124530135,20.8302785517541,20.5710289665452));
#62610=CARTESIAN_POINT('Ctrl Pts',(146.296085688653,20.6794014224469,20.6914734862116));
#62611=CARTESIAN_POINT('Ctrl Pts',(137.573606580749,19.285264282887,19.6233996664196));
#62612=CARTESIAN_POINT('Ctrl Pts',(130.379397788771,15.6240250517759,15.6701139528965));
#62613=CARTESIAN_POINT('Ctrl Pts',(127.284956078127,13.0852837400994,12.7235960532101));
#62614=CARTESIAN_POINT('Ctrl Pts',(150.020722457357,20.9266043917347,20.2235451151067));
#62615=CARTESIAN_POINT('Ctrl Pts',(146.304992407354,20.7810198218841,20.3784783618164));
#62616=CARTESIAN_POINT('Ctrl Pts',(137.620776897837,19.3976728540394,19.3965609983574));
#62617=CARTESIAN_POINT('Ctrl Pts',(130.420987560279,15.7288387535583,15.5137933491637));
#62618=CARTESIAN_POINT('Ctrl Pts',(127.32129741028,13.1815939383356,12.5992378142346));
#62619=CARTESIAN_POINT('Ctrl Pts',(150.000022383365,21.1486749640491,19.9885854250535));
#62620=CARTESIAN_POINT('Ctrl Pts',(146.292010366741,20.9855352203964,20.1610725772885));
#62621=CARTESIAN_POINT('Ctrl Pts',(137.62131468814,19.56481049896,19.2230426654884));
#62622=CARTESIAN_POINT('Ctrl Pts',(130.426320545001,15.8608035501812,15.3832517941273));
#62623=CARTESIAN_POINT('Ctrl Pts',(127.328278974586,13.2952172871523,12.4909704719795));
#62624=CARTESIAN_POINT('',(127.849160658792,13.516786884833,13.433913805062));
#62625=CARTESIAN_POINT('Ctrl Pts',(150.052788176357,20.8995478588044,20.8872814140596));
#62626=CARTESIAN_POINT('Ctrl Pts',(146.270211476078,20.7172956805484,20.9902923738357));
#62627=CARTESIAN_POINT('Ctrl Pts',(137.824437935169,19.3096465398735,19.9001633861864));
#62628=CARTESIAN_POINT('Ctrl Pts',(130.853616103513,15.8376680620727,16.1313846441183));
#62629=CARTESIAN_POINT('Ctrl Pts',(127.849390477171,13.5165305749893,13.4338784035216));
#62630=CARTESIAN_POINT('Ctrl Pts',(127.464959760401,13.2135636128055,13.0809546870671));
#62631=CARTESIAN_POINT('Ctrl Pts',(127.591474039885,13.3152779704247,13.1997176167124));
#62632=CARTESIAN_POINT('Ctrl Pts',(127.719628570138,13.416273382531,13.3173646666896));
#62633=CARTESIAN_POINT('Ctrl Pts',(127.849390477171,13.5165305749893,13.4338784035216));
#62634=CARTESIAN_POINT('Ctrl Pts',(127.223161057304,4.62069507309356,17.6980789259147));
#62635=CARTESIAN_POINT('Ctrl Pts',(129.536338162995,5.60202902444579,20.4683748308861));
#62636=CARTESIAN_POINT('Ctrl Pts',(136.26237808218,7.40494313500673,26.0127509394373));
#62637=CARTESIAN_POINT('Ctrl Pts',(145.009334199416,7.87959000871871,28.40140323231));
#62638=CARTESIAN_POINT('Ctrl Pts',(150.052765342883,7.63914347976157,28.5431794384981));
#62639=CARTESIAN_POINT('Ctrl Pts',(127.284956078127,4.47631553952168,17.6939861612584));
#62640=CARTESIAN_POINT('Ctrl Pts',(129.605785359723,5.43810623361003,20.447888850951));
#62641=CARTESIAN_POINT('Ctrl Pts',(136.344272439013,7.19418974794387,25.9357158412589));
#62642=CARTESIAN_POINT('Ctrl Pts',(145.047721144697,7.63955590095541,28.2311393820031));
#62643=CARTESIAN_POINT('Ctrl Pts',(150.04110192192,7.39989547846868,28.3250644474042));
#62644=CARTESIAN_POINT('Ctrl Pts',(127.321297410279,4.3204630462809,17.7152141200868));
#62645=CARTESIAN_POINT('Ctrl Pts',(129.646063017998,5.25830478230839,20.4626541161376));
#62646=CARTESIAN_POINT('Ctrl Pts',(136.39103938847,6.95203943573214,25.9261288558874));
#62647=CARTESIAN_POINT('Ctrl Pts',(145.066397536229,7.32675906387257,28.169921998372));
#62648=CARTESIAN_POINT('Ctrl Pts',(150.020700025828,7.05080287918935,28.2347432775899));
#62649=CARTESIAN_POINT('Ctrl Pts',(127.328278974586,4.1698891030794,17.7594811554976));
#62650=CARTESIAN_POINT('Ctrl Pts',(129.651808148682,5.08638528899869,20.510481438492));
#62651=CARTESIAN_POINT('Ctrl Pts',(136.392518944088,6.72647599839076,25.9832187747262));
#62652=CARTESIAN_POINT('Ctrl Pts',(145.055988202065,7.0442157893323,28.2361925256675));
#62653=CARTESIAN_POINT('Ctrl Pts',(150.,6.73628667589916,28.3095821555194));
#62654=CARTESIAN_POINT('',(127.849160658776,4.87571718501569,18.4228377223213));
#62655=CARTESIAN_POINT('',(150.052765342883,7.63914347976157,28.5431794384981));
#62656=CARTESIAN_POINT('Ctrl Pts',(127.849241699155,4.87579936496748,18.422737486504));
#62657=CARTESIAN_POINT('Ctrl Pts',(130.04840826906,5.7366102401665,20.8835740463298));
#62658=CARTESIAN_POINT('Ctrl Pts',(136.593459162601,7.42290899623439,26.1031638295071));
#62659=CARTESIAN_POINT('Ctrl Pts',(145.009334199416,7.87959000871871,28.40140323231));
#62660=CARTESIAN_POINT('Ctrl Pts',(150.052765342883,7.63914347976157,28.5431794384981));
#62661=CARTESIAN_POINT('Origin',(149.99997684747,6.96777419047282,29.2824200300188));
#62662=CARTESIAN_POINT('Ctrl Pts',(127.849241699155,4.87579936496749,18.422737486504));
#62663=CARTESIAN_POINT('Ctrl Pts',(127.719533634134,4.82502826172371,18.2775959802282));
#62664=CARTESIAN_POINT('Ctrl Pts',(127.591421328901,4.77364483852168,18.1312675183373));
#62665=CARTESIAN_POINT('Ctrl Pts',(127.464935601762,4.72165458526838,17.9837809392299));
#62666=CARTESIAN_POINT('Ctrl Pts',(150.052765342888,7.63914347997585,28.543179438693));
#62667=CARTESIAN_POINT('Ctrl Pts',(152.873899737654,7.50459235942636,28.6224363823327));
#62668=CARTESIAN_POINT('Ctrl Pts',(157.868054239131,7.48947070771599,28.6380213444408));
#62669=CARTESIAN_POINT('Ctrl Pts',(162.799391993723,7.77414906196946,28.4582099509193));
#62670=CARTESIAN_POINT('Ctrl Pts',(164.848300728756,8.11744071417838,28.3085740825388));
#62671=CARTESIAN_POINT('Ctrl Pts',(150.041092860165,7.39989567784295,28.3250639813971));
#62672=CARTESIAN_POINT('Ctrl Pts',(152.871543860118,7.26494492056672,28.3795305178101));
#62673=CARTESIAN_POINT('Ctrl Pts',(157.870048819568,7.25088318119086,28.3876583063541));
#62674=CARTESIAN_POINT('Ctrl Pts',(162.821033665546,7.53515773248278,28.2683647093993));
#62675=CARTESIAN_POINT('Ctrl Pts',(164.88605042119,7.88661064663083,28.148507820487));
#62676=CARTESIAN_POINT('Ctrl Pts',(150.020682003358,7.05080292959874,28.2347427729539));
#62677=CARTESIAN_POINT('Ctrl Pts',(152.866096267055,6.89616829156458,28.2730885857043));
#62678=CARTESIAN_POINT('Ctrl Pts',(157.875799048708,6.87704176638768,28.2763458416187));
#62679=CARTESIAN_POINT('Ctrl Pts',(162.857516536512,7.20827135825618,28.1970467495269));
#62680=CARTESIAN_POINT('Ctrl Pts',(164.942784455248,7.58820374378898,28.0945941257697));
#62681=CARTESIAN_POINT('Ctrl Pts',(149.999976847469,6.73628667607159,28.3095821554784));
#62682=CARTESIAN_POINT('Ctrl Pts',(152.860533470273,6.56398345605622,28.3505818381604));
#62683=CARTESIAN_POINT('Ctrl Pts',(157.881732552083,6.54033302449913,28.3550238051405));
#62684=CARTESIAN_POINT('Ctrl Pts',(162.894448253278,6.9134586222552,28.2699510051099));
#62685=CARTESIAN_POINT('Ctrl Pts',(165.000000000548,7.31954028967603,28.1644160235537));
#62686=CARTESIAN_POINT('Ctrl Pts',(150.052765342888,7.63914347997585,28.543179438693));
#62687=CARTESIAN_POINT('Ctrl Pts',(152.873899737654,7.50459235942636,28.6224363823327));
#62688=CARTESIAN_POINT('Ctrl Pts',(157.868054239131,7.48947070771599,28.6380213444408));
#62689=CARTESIAN_POINT('Ctrl Pts',(162.799391993723,7.77414906196946,28.4582099509193));
#62690=CARTESIAN_POINT('Ctrl Pts',(164.848300728756,8.11744071417838,28.3085740825388));
#62691=CARTESIAN_POINT('',(164.9482248766,7.57107088382297,28.1336066026226));
#62692=CARTESIAN_POINT('Origin',(165.000000000548,7.57107088382297,29.1322653714422));
#62693=CARTESIAN_POINT('',(165.000000000274,7.31954028967603,28.1644160235537));
#62694=CARTESIAN_POINT('Origin',(165.000000000548,7.57107088382297,29.1322653714422));
#62695=CARTESIAN_POINT('Ctrl Pts',(165.000000000548,7.31954028967603,28.1644160235537));
#62696=CARTESIAN_POINT('Ctrl Pts',(162.894448253278,6.9134586222552,28.2699510051099));
#62697=CARTESIAN_POINT('Ctrl Pts',(157.881740250478,6.54033359753546,28.355023674488));
#62698=CARTESIAN_POINT('Ctrl Pts',(152.86054889312,6.56398338341375,28.3505818518039));
#62699=CARTESIAN_POINT('Ctrl Pts',(149.999999911594,6.73628528682695,28.3095824860502));
#62700=CARTESIAN_POINT('Origin',(165.,7.57107088382297,29.1322653714422));
#62701=CARTESIAN_POINT('Origin',(165.,7.57107088382297,29.1322653714422));
#62702=CARTESIAN_POINT('',(165.,7.57107088382297,28.1322653714422));
#62703=CARTESIAN_POINT('Origin',(165.,7.57107088382297,29.1322653714422));
#62704=CARTESIAN_POINT('Origin',(158.5,0.,0.));
#62705=CARTESIAN_POINT('Origin',(165.,0.,0.));
#62706=CARTESIAN_POINT('Origin',(165.,0.,0.));
#62707=CARTESIAN_POINT('Origin',(166.,0.,0.));
#62708=CARTESIAN_POINT('Origin',(166.,0.,0.));
#62709=CARTESIAN_POINT('',(166.,-4.77612251667468E-15,39.));
#62710=CARTESIAN_POINT('Origin',(166.,0.,0.));
#62711=CARTESIAN_POINT('',(166.,21.4437464396283,-21.1228724048769));
#62712=CARTESIAN_POINT('Origin',(166.,0.,0.));
#62713=CARTESIAN_POINT('',(166.,7.57107088371365,-29.1322653714706));
#62714=CARTESIAN_POINT('Ctrl Pts',(166.,7.57107088371365,-29.1322653714706));
#62715=CARTESIAN_POINT('Ctrl Pts',(166.,7.83004053020818,-29.3040447792846));
#62716=CARTESIAN_POINT('Ctrl Pts',(166.,8.09758144625251,-29.4628272998432));
#62717=CARTESIAN_POINT('Ctrl Pts',(166.,8.37226172741755,-29.6080560830666));
#62718=CARTESIAN_POINT('Ctrl Pts',(166.,8.65151782956149,-29.7557041914421));
#62719=CARTESIAN_POINT('Ctrl Pts',(166.,8.93815390120195,-29.8893437091583));
#62720=CARTESIAN_POINT('Ctrl Pts',(166.,9.23069869083415,-30.0083479991698));
#62721=CARTESIAN_POINT('Ctrl Pts',(166.,9.29469045482918,-30.0343792077598));
#62722=CARTESIAN_POINT('Ctrl Pts',(166.,9.35896503860058,-30.0597099793644));
#62723=CARTESIAN_POINT('Ctrl Pts',(166.,9.42350719522099,-30.0843334608257));
#62724=CARTESIAN_POINT('Ctrl Pts',(166.,9.74517827870872,-30.207054212279));
#62725=CARTESIAN_POINT('Ctrl Pts',(166.000000159105,10.0737946755819,-30.312108388683));
#62726=CARTESIAN_POINT('Ctrl Pts',(166.000000291074,10.4072025190414,-30.3986003326517));
#62727=CARTESIAN_POINT('Ctrl Pts',(166.000000422447,10.7391037489439,-30.4847014341796));
#62728=CARTESIAN_POINT('Ctrl Pts',(166.000000483618,11.075752167306,-30.5524085248586));
#62729=CARTESIAN_POINT('Ctrl Pts',(166.00000044277,11.4150550044157,-30.6008782566214));
#62730=CARTESIAN_POINT('Ctrl Pts',(166.000000402416,11.7502480494005,-30.6487609006853));
#62731=CARTESIAN_POINT('Ctrl Pts',(166.000000290454,12.088030947372,-30.6778704752216));
#62732=CARTESIAN_POINT('Ctrl Pts',(166.000000335807,12.4264299077261,-30.6874188265614));
#62733=CARTESIAN_POINT('Ctrl Pts',(166.000000358569,12.5962741233716,-30.6922111942516));
#62734=CARTESIAN_POINT('Ctrl Pts',(166.000000423249,12.7662742867479,-30.69207621128));
#62735=CARTESIAN_POINT('Ctrl Pts',(166.00000051567,12.9361857334605,-30.6869152176631));
#62736=CARTESIAN_POINT('Ctrl Pts',(166.000000522059,12.9479317733612,-30.6865584363036));
#62737=CARTESIAN_POINT('Ctrl Pts',(166.00000052853,12.9596769619444,-30.6861776146845));
#62738=CARTESIAN_POINT('Ctrl Pts',(166.000000535057,12.9714212220908,-30.6857727098352));
#62739=CARTESIAN_POINT('Ctrl Pts',(166.00000069439,13.2581246423604,-30.6758880850285));
#62740=CARTESIAN_POINT('Ctrl Pts',(166.000000856491,13.5442788051857,-30.6516525281821));
#62741=CARTESIAN_POINT('Ctrl Pts',(166.000000781528,13.8285584126196,-30.6134264603874));
#62742=CARTESIAN_POINT('Ctrl Pts',(166.000000706633,14.1125777565279,-30.5752353893033));
#62743=CARTESIAN_POINT('Ctrl Pts',(166.000000393888,14.394726170477,-30.5230782585526));
#62744=CARTESIAN_POINT('Ctrl Pts',(166.000000175973,14.6736310564209,-30.4573056218602));
#62745=CARTESIAN_POINT('Ctrl Pts',(166.000000073066,14.8053400716756,-30.4262453943559));
#62746=CARTESIAN_POINT('Ctrl Pts',(166.,14.9363250021618,-30.3921487914719));
#62747=CARTESIAN_POINT('Ctrl Pts',(166.,15.0664372627468,-30.3550531378469));
#62748=CARTESIAN_POINT('Ctrl Pts',(166.,15.3339756489133,-30.2787766112536));
#62749=CARTESIAN_POINT('Ctrl Pts',(166.000000002737,15.5979488938777,-30.1900046692528));
#62750=CARTESIAN_POINT('Ctrl Pts',(166.000000127251,15.8571799519466,-30.0890423037444));
#62751=CARTESIAN_POINT('Ctrl Pts',(166.000000250915,16.1146424441111,-29.9887687391792));
#62752=CARTESIAN_POINT('Ctrl Pts',(166.000000528009,16.367427574929,-29.8764697667648));
#62753=CARTESIAN_POINT('Ctrl Pts',(166.000000806601,16.614335295693,-29.7524238352534));
#62754=CARTESIAN_POINT('Ctrl Pts',(166.000000970618,16.7596980311003,-29.6793938957081));
#62755=CARTESIAN_POINT('Ctrl Pts',(166.000001129098,16.9030226986056,-29.602292055648));
#62756=CARTESIAN_POINT('Ctrl Pts',(166.00000110863,17.0440561282011,-29.5211733572009));
#62757=CARTESIAN_POINT('Ctrl Pts',(166.000001073423,17.286656561197,-29.381636004789));
#62758=CARTESIAN_POINT('Ctrl Pts',(166.000000588789,17.5227450134798,-29.2305789697212));
#62759=CARTESIAN_POINT('Ctrl Pts',(166.000000325308,17.7509155586326,-29.0683867660758));
#62760=CARTESIAN_POINT('Ctrl Pts',(166.000000140464,17.9109867821603,-28.954602121056));
#62761=CARTESIAN_POINT('Ctrl Pts',(166.000000036969,18.0671608568786,-28.8353382434822));
#62762=CARTESIAN_POINT('Ctrl Pts',(166.00000003186,18.2189526914256,-28.7107432283143));
#62763=CARTESIAN_POINT('Ctrl Pts',(166.000000024651,18.4331800450233,-28.5348993797271));
#62764=CARTESIAN_POINT('Ctrl Pts',(166.000000207213,18.6386776232909,-28.3484347663401));
#62765=CARTESIAN_POINT('Ctrl Pts',(166.000000406871,18.8347637893741,-28.1525130754886));
#62766=CARTESIAN_POINT('Ctrl Pts',(166.000000608185,19.0324762725667,-27.9549664316672));
#62767=CARTESIAN_POINT('Ctrl Pts',(166.000000810431,19.2206198910017,-27.747805587876));
#62768=CARTESIAN_POINT('Ctrl Pts',(166.000000870095,19.3985194120509,-27.5322706372802));
#62769=CARTESIAN_POINT('Ctrl Pts',(166.000000890677,19.4598876247081,-27.4579197081422));
#62770=CARTESIAN_POINT('Ctrl Pts',(166.000000895603,19.5200370689442,-27.382572663073));
#62771=CARTESIAN_POINT('Ctrl Pts',(166.000000883847,19.5789409024478,-27.3062815474031));
#62772=CARTESIAN_POINT('Ctrl Pts',(166.000000845523,19.770965835375,-27.0575745363636));
#62773=CARTESIAN_POINT('Ctrl Pts',(166.000000681352,19.9496915008844,-26.7986294338229));
#62774=CARTESIAN_POINT('Ctrl Pts',(166.000000634525,20.1144114968893,-26.5310493135424));
#62775=CARTESIAN_POINT('Ctrl Pts',(166.000000587307,20.2805107765448,-26.2612286098833));
#62776=CARTESIAN_POINT('Ctrl Pts',(166.00000064022,20.4323695370564,-25.9826270218258));
#62777=CARTESIAN_POINT('Ctrl Pts',(166.00000057971,20.5692332852027,-25.6968442162184));
#62778=CARTESIAN_POINT('Ctrl Pts',(166.000000519663,20.7050484978224,-25.4132508393577));
#62779=CARTESIAN_POINT('Ctrl Pts',(166.000000331685,20.82609817904,-25.1225850541402));
#62780=CARTESIAN_POINT('Ctrl Pts',(165.999999620488,20.9316059215766,-24.8263779294654));
#62781=CARTESIAN_POINT('Ctrl Pts',(165.999999157238,21.0003300972401,-24.6334386249221));
#62782=CARTESIAN_POINT('Ctrl Pts',(165.999998469154,21.0624593578499,-24.4381476220006));
#62783=CARTESIAN_POINT('Ctrl Pts',(165.999997448035,21.1177682304653,-24.2409231385358));
#62784=CARTESIAN_POINT('Ctrl Pts',(165.999996954395,21.1445061940392,-24.1455789233059));
#62785=CARTESIAN_POINT('Ctrl Pts',(165.999996561405,21.1697129928577,-24.0498155701719));
#62786=CARTESIAN_POINT('Ctrl Pts',(165.999996314061,21.1933528657877,-23.9536778109361));
#62787=CARTESIAN_POINT('Ctrl Pts',(165.999995700107,21.2520315470248,-23.7150455244703));
#62788=CARTESIAN_POINT('Ctrl Pts',(165.999996042829,21.3010563042617,-23.4741026935105));
#62789=CARTESIAN_POINT('Ctrl Pts',(165.999996747874,21.3404743469592,-23.2315544115253));
#62790=CARTESIAN_POINT('Ctrl Pts',(165.999997458547,21.3802069773542,-22.9870703990887));
#62791=CARTESIAN_POINT('Ctrl Pts',(165.999998430315,21.410178121117,-22.7409553237713));
#62792=CARTESIAN_POINT('Ctrl Pts',(165.999999046094,21.4304371697996,-22.4939848489898));
#62793=CARTESIAN_POINT('Ctrl Pts',(165.999999670447,21.450978268046,-22.2435760136133));
#62794=CARTESIAN_POINT('Ctrl Pts',(165.999999930442,21.4615341907363,-21.9922880212504));
#62795=CARTESIAN_POINT('Ctrl Pts',(165.999999988173,21.4621696368845,-21.7409817270757));
#62796=CARTESIAN_POINT('Ctrl Pts',(166.000000035541,21.4626910071418,-21.5347901754403));
#62797=CARTESIAN_POINT('Ctrl Pts',(166.,21.4565341578357,-21.3285874117133));
#62798=CARTESIAN_POINT('Ctrl Pts',(166.,21.4437464396259,-21.122872404877));
#62799=CARTESIAN_POINT('',(166.,-7.57107088371367,-29.1322653714706));
#62800=CARTESIAN_POINT('Origin',(166.,0.,0.));
#62801=CARTESIAN_POINT('',(166.,-21.4437464396264,-21.122872404884));
#62802=CARTESIAN_POINT('Ctrl Pts',(166.,-21.4437464396264,-21.122872404884));
#62803=CARTESIAN_POINT('Ctrl Pts',(166.,-21.4730902429887,-21.5949238381669));
#62804=CARTESIAN_POINT('Ctrl Pts',(166.,-21.4660747258147,-22.0691189640469));
#62805=CARTESIAN_POINT('Ctrl Pts',(166.,-21.4236081971921,-22.5400060170313));
#62806=CARTESIAN_POINT('Ctrl Pts',(166.,-21.4109501846545,-22.6803634800453));
#62807=CARTESIAN_POINT('Ctrl Pts',(166.,-21.3951423877454,-22.8204271371756));
#62808=CARTESIAN_POINT('Ctrl Pts',(166.,-21.376208592825,-22.9600528541274));
#62809=CARTESIAN_POINT('Ctrl Pts',(166.,-21.3642721852941,-23.0480769119745));
#62810=CARTESIAN_POINT('Ctrl Pts',(166.,-21.3510936663369,-23.1359251753596));
#62811=CARTESIAN_POINT('Ctrl Pts',(166.,-21.3366780668093,-23.223567006887));
#62812=CARTESIAN_POINT('Ctrl Pts',(166.,-21.2691471910605,-23.6341312448807));
#62813=CARTESIAN_POINT('Ctrl Pts',(166.,-21.1744310943715,-24.0403583096884));
#62814=CARTESIAN_POINT('Ctrl Pts',(166.,-21.0530750066224,-24.4384050249842));
#62815=CARTESIAN_POINT('Ctrl Pts',(166.,-20.9320358347896,-24.8354122593454));
#62816=CARTESIAN_POINT('Ctrl Pts',(166.,-20.7844958260855,-25.2242806659143));
#62817=CARTESIAN_POINT('Ctrl Pts',(166.,-20.6110468351356,-25.6012005910559));
#62818=CARTESIAN_POINT('Ctrl Pts',(166.,-20.4617479644695,-25.9256401790118));
#62819=CARTESIAN_POINT('Ctrl Pts',(166.,-20.2932535703279,-26.2412265712482));
#62820=CARTESIAN_POINT('Ctrl Pts',(166.,-20.1059697568712,-26.5455419852988));
#62821=CARTESIAN_POINT('Ctrl Pts',(166.,-20.1001525156399,-26.5549943567625));
#62822=CARTESIAN_POINT('Ctrl Pts',(166.000000000186,-20.0943171161851,-26.5644355966982));
#62823=CARTESIAN_POINT('Ctrl Pts',(166.000000000555,-20.0884635728741,-26.5738656418205));
#62824=CARTESIAN_POINT('Ctrl Pts',(166.000000010114,-19.9368020374074,-26.8181920347077));
#62825=CARTESIAN_POINT('Ctrl Pts',(166.000000149751,-19.7729649448078,-27.0550028229082));
#62826=CARTESIAN_POINT('Ctrl Pts',(166.000000307122,-19.5978664987802,-27.2831783580798));
#62827=CARTESIAN_POINT('Ctrl Pts',(166.000000464033,-19.4232787574551,-27.5106883800989));
#62828=CARTESIAN_POINT('Ctrl Pts',(166.000000627557,-19.2374952261309,-27.729614318751));
#62829=CARTESIAN_POINT('Ctrl Pts',(166.000000737599,-19.0413707124309,-27.9388457161969));
#62830=CARTESIAN_POINT('Ctrl Pts',(166.00000078943,-18.9489936376693,-28.0373962955186));
#62831=CARTESIAN_POINT('Ctrl Pts',(166.000000831221,-18.854321650251,-28.1337960260855));
#62832=CARTESIAN_POINT('Ctrl Pts',(166.000000864069,-18.7574401582065,-28.2279279316741));
#62833=CARTESIAN_POINT('Ctrl Pts',(166.000000922928,-18.5838399404868,-28.3966012144624));
#62834=CARTESIAN_POINT('Ctrl Pts',(166.000000927263,-18.40321617359,-28.5580944632899));
#62835=CARTESIAN_POINT('Ctrl Pts',(166.000000855042,-18.2160373229752,-28.7115457683194));
#62836=CARTESIAN_POINT('Ctrl Pts',(166.000000778403,-18.017408917564,-28.8743835458042));
#62837=CARTESIAN_POINT('Ctrl Pts',(166.000000581255,-17.8113982127703,-29.028164757989));
#62838=CARTESIAN_POINT('Ctrl Pts',(166.000000364475,-17.5989289637878,-29.1724110415025));
#62839=CARTESIAN_POINT('Ctrl Pts',(166.000000180024,-17.4181460424616,-29.2951453414019));
#62840=CARTESIAN_POINT('Ctrl Pts',(166.,-17.2326881513708,-29.4109761553419));
#62841=CARTESIAN_POINT('Ctrl Pts',(166.,-17.0431540821677,-29.5196079817917));
#62842=CARTESIAN_POINT('Ctrl Pts',(166.,-16.7509530058835,-29.6870836063103));
#62843=CARTESIAN_POINT('Ctrl Pts',(166.000000001485,-16.4491709339976,-29.8377114671915));
#62844=CARTESIAN_POINT('Ctrl Pts',(166.000000058288,-16.1398333007634,-29.9707755422833));
#62845=CARTESIAN_POINT('Ctrl Pts',(166.000000115169,-15.8300685390054,-30.1040233501507));
#62846=CARTESIAN_POINT('Ctrl Pts',(166.000000234944,-15.5127262816327,-30.219658815692));
#62847=CARTESIAN_POINT('Ctrl Pts',(166.000000399126,-15.1898376465784,-30.3169109067421));
#62848=CARTESIAN_POINT('Ctrl Pts',(166.000000561094,-14.8713033264944,-30.4128515046333));
#62849=CARTESIAN_POINT('Ctrl Pts',(166.000000778141,-14.5473703407301,-30.4909010346141));
#62850=CARTESIAN_POINT('Ctrl Pts',(166.000000817451,-14.2200003703573,-30.550270223197));
#62851=CARTESIAN_POINT('Ctrl Pts',(166.000000831876,-14.0998744017677,-30.5720553040789));
#62852=CARTESIAN_POINT('Ctrl Pts',(166.000000819335,-13.9792858317496,-30.5913246679811));
#62853=CARTESIAN_POINT('Ctrl Pts',(166.000000755466,-13.8583323190612,-30.6080377018107));
#62854=CARTESIAN_POINT('Ctrl Pts',(166.000000611996,-13.5866299184372,-30.6455808149646));
#62855=CARTESIAN_POINT('Ctrl Pts',(166.000000400635,-13.3131780594187,-30.6705576589936));
#62856=CARTESIAN_POINT('Ctrl Pts',(166.000000386486,-13.0391717726041,-30.6824342864098));
#62857=CARTESIAN_POINT('Ctrl Pts',(166.000000385323,-13.0166374831848,-30.6834110207856));
#62858=CARTESIAN_POINT('Ctrl Pts',(166.000000384991,-12.9940994691275,-30.6842991675762));
#62859=CARTESIAN_POINT('Ctrl Pts',(166.000000385417,-12.9715584083925,-30.6850984382124));
#62860=CARTESIAN_POINT('Ctrl Pts',(166.000000390602,-12.6968779520138,-30.6948381760945));
#62861=CARTESIAN_POINT('Ctrl Pts',(166.000000509378,-12.4217419519583,-30.6913773585857));
#62862=CARTESIAN_POINT('Ctrl Pts',(166.000000541215,-12.1473047666949,-30.6750903619261));
#62863=CARTESIAN_POINT('Ctrl Pts',(166.000000574714,-11.8585542992748,-30.6579539163172));
#62864=CARTESIAN_POINT('Ctrl Pts',(166.00000048955,-11.5705779645419,-30.6266175841477));
#62865=CARTESIAN_POINT('Ctrl Pts',(166.000000336381,-11.2847581981821,-30.5815663641647));
#62866=CARTESIAN_POINT('Ctrl Pts',(166.000000183212,-10.9989384318223,-30.5365151441817));
#62867=CARTESIAN_POINT('Ctrl Pts',(166.,-10.7152763081471,-30.4777486389399));
#62868=CARTESIAN_POINT('Ctrl Pts',(166.,-10.4351784858912,-30.4058090618878));
#62869=CARTESIAN_POINT('Ctrl Pts',(166.,-10.1471083995595,-30.3318219098094));
#62870=CARTESIAN_POINT('Ctrl Pts',(166.,-9.86257911748525,-30.2440540838133));
#62871=CARTESIAN_POINT('Ctrl Pts',(166.,-9.58279349157084,-30.1430848782976));
#62872=CARTESIAN_POINT('Ctrl Pts',(166.,-9.30214716915257,-30.0418050641082));
#62873=CARTESIAN_POINT('Ctrl Pts',(166.,-9.0262728955537,-29.9272421830346));
#62874=CARTESIAN_POINT('Ctrl Pts',(166.,-8.75639934231564,-29.7999305363866));
#62875=CARTESIAN_POINT('Ctrl Pts',(166.,-8.49014435239758,-29.6743259308668));
#62876=CARTESIAN_POINT('Ctrl Pts',(166.,-8.22972950154706,-29.5363117066743));
#62877=CARTESIAN_POINT('Ctrl Pts',(166.,-7.97636062282865,-29.3863580367982));
#62878=CARTESIAN_POINT('Ctrl Pts',(166.,-7.8391312538349,-29.3051402976684));
#62879=CARTESIAN_POINT('Ctrl Pts',(166.,-7.70396934312996,-29.2204194040645));
#62880=CARTESIAN_POINT('Ctrl Pts',(166.,-7.57107088371367,-29.1322653714706));
#62881=CARTESIAN_POINT('',(166.,-29.0148173233401,-8.00939296658655));
#62882=CARTESIAN_POINT('Origin',(166.,0.,0.));
#62883=CARTESIAN_POINT('',(166.,-29.0148173233401,8.00939296658655));
#62884=CARTESIAN_POINT('Ctrl Pts',(166.,-29.0148173233401,8.00939296658655));
#62885=CARTESIAN_POINT('Ctrl Pts',(166.,-29.293093946098,7.87099521401071));
#62886=CARTESIAN_POINT('Ctrl Pts',(166.,-29.5643994941033,7.71867387250682));
#62887=CARTESIAN_POINT('Ctrl Pts',(166.,-29.8275353737714,7.55339060593392));
#62888=CARTESIAN_POINT('Ctrl Pts',(166.,-30.0950457426212,7.38535959601848));
#62889=CARTESIAN_POINT('Ctrl Pts',(166.,-30.3541133506983,7.20393169429305));
#62890=CARTESIAN_POINT('Ctrl Pts',(166.,-30.6034595798187,7.01006765798923));
#62891=CARTESIAN_POINT('Ctrl Pts',(166.,-30.6579600229528,6.9676941441664));
#62892=CARTESIAN_POINT('Ctrl Pts',(166.,-30.7119959355182,6.92472633093575));
#62893=CARTESIAN_POINT('Ctrl Pts',(166.,-30.7655537869963,6.88117397281331));
#62894=CARTESIAN_POINT('Ctrl Pts',(166.,-31.0322558723588,6.6642962524954));
#62895=CARTESIAN_POINT('Ctrl Pts',(166.000000158692,-31.2871670140499,6.43261545973507));
#62896=CARTESIAN_POINT('Ctrl Pts',(166.000000288096,-31.5284431714344,6.18754302714617));
#62897=CARTESIAN_POINT('Ctrl Pts',(166.000000416912,-31.7686244030884,5.94358274801323));
#62898=CARTESIAN_POINT('Ctrl Pts',(166.000000473135,-31.9952943240445,5.68635342611851));
#62899=CARTESIAN_POINT('Ctrl Pts',(166.000000425645,-32.2066847316412,5.41723973717625));
#62900=CARTESIAN_POINT('Ctrl Pts',(166.00000037873,-32.4155204913965,5.15137828050124));
#62901=CARTESIAN_POINT('Ctrl Pts',(166.000000258431,-32.609444425045,4.87391907202096));
#62902=CARTESIAN_POINT('Ctrl Pts',(166.000000299509,-32.7867951988191,4.58617171689115));
#62903=CARTESIAN_POINT('Ctrl Pts',(166.000000320352,-32.8767810021532,4.44017192023056));
#62904=CARTESIAN_POINT('Ctrl Pts',(166.000000385309,-32.9625007992022,4.29152299581416));
#62905=CARTESIAN_POINT('Ctrl Pts',(166.000000480688,-33.0437410090145,4.1403921355856));
#62906=CARTESIAN_POINT('Ctrl Pts',(166.000000487214,-33.0493003801265,4.13005005817798));
#62907=CARTESIAN_POINT('Ctrl Pts',(166.000000493832,-33.0548385430632,4.11969671755402));
#62908=CARTESIAN_POINT('Ctrl Pts',(166.000000500513,-33.0603554221985,4.10933215884169));
#62909=CARTESIAN_POINT('Ctrl Pts',(166.000000663467,-33.1949054221804,3.85655312555729));
#62910=CARTESIAN_POINT('Ctrl Pts',(166.000000834147,-33.3167989647159,3.59709872522229));
#62911=CARTESIAN_POINT('Ctrl Pts',(166.000000766845,-33.4256866809306,3.33228920628611));
#62912=CARTESIAN_POINT('Ctrl Pts',(166.000000699609,-33.534467987921,3.06773846929978));
#62913=CARTESIAN_POINT('Ctrl Pts',(166.00000039332,-33.6302679753089,2.79784233206316));
#62914=CARTESIAN_POINT('Ctrl Pts',(166.000000176938,-33.7127051805426,2.52395687836087));
#62915=CARTESIAN_POINT('Ctrl Pts',(166.000000073764,-33.7520125507797,2.39336393915683));
#62916=CARTESIAN_POINT('Ctrl Pts',(166.,-33.7882814458652,2.26186466737644));
#62917=CARTESIAN_POINT('Ctrl Pts',(166.,-33.8214687969989,2.12960988893744));
#62918=CARTESIAN_POINT('Ctrl Pts',(166.,-33.8891925373905,1.85972428569978));
#62919=CARTESIAN_POINT('Ctrl Pts',(166.000000002729,-33.9443074633459,1.58667737475891));
#62920=CARTESIAN_POINT('Ctrl Pts',(166.000000125327,-33.9864892592845,1.31164169793362));
#62921=CARTESIAN_POINT('Ctrl Pts',(166.000000247087,-34.0283829088393,1.03848480635044));
#62922=CARTESIAN_POINT('Ctrl Pts',(166.00000052026,-34.0575190389966,0.763365555152333));
#62923=CARTESIAN_POINT('Ctrl Pts',(166.000000792151,-34.0735388057827,0.48746302572961));
#62924=CARTESIAN_POINT('Ctrl Pts',(166.00000095209,-34.0829623947314,0.325164032123184));
#62925=CARTESIAN_POINT('Ctrl Pts',(166.000001105543,-34.0878465174028,0.162594627370444));
#62926=CARTESIAN_POINT('Ctrl Pts',(166.000001079992,-34.0881124511405,1.08249490214136E-6));
#62927=CARTESIAN_POINT('Ctrl Pts',(166.000001036017,-34.0885701328409,-0.279828361977705));
#62928=CARTESIAN_POINT('Ctrl Pts',(166.000000548897,-34.0757989238753,-0.559778156892051));
#62929=CARTESIAN_POINT('Ctrl Pts',(166.000000285027,-34.0494289016247,-0.838438953656794));
#62930=CARTESIAN_POINT('Ctrl Pts',(166.000000099859,-34.0309240606458,-1.0339857636749));
#62931=CARTESIAN_POINT('Ctrl Pts',(165.999999997169,-34.0057234665799,-1.2288970643696));
#62932=CARTESIAN_POINT('Ctrl Pts',(165.999999993221,-33.973712744161,-1.4226784498747));
#62933=CARTESIAN_POINT('Ctrl Pts',(165.99999998765,-33.9285479936293,-1.6960895844161));
#62934=CARTESIAN_POINT('Ctrl Pts',(166.000000172381,-33.86982394846,-1.96725146028262));
#62935=CARTESIAN_POINT('Ctrl Pts',(166.000000374259,-33.7982072336778,-2.234992328549));
#62936=CARTESIAN_POINT('Ctrl Pts',(166.000000577811,-33.7259967976075,-2.50495283860762));
#62937=CARTESIAN_POINT('Ctrl Pts',(166.000000782421,-33.6406790391978,-2.77143458587085));
#62938=CARTESIAN_POINT('Ctrl Pts',(166.000000845274,-33.5429899376099,-3.03323316113975));
#62939=CARTESIAN_POINT('Ctrl Pts',(166.000000866978,-33.5092565235904,-3.12363587327143));
#62940=CARTESIAN_POINT('Ctrl Pts',(166.000000873097,-33.4740483856741,-3.21348018362735));
#62941=CARTESIAN_POINT('Ctrl Pts',(166.000000862634,-33.437397258621,-3.30271668758227));
#62942=CARTESIAN_POINT('Ctrl Pts',(166.00000082854,-33.3179655528545,-3.59350359485862));
#62943=CARTESIAN_POINT('Ctrl Pts',(166.000000667342,-33.1830048840627,-3.87788651140105));
#62944=CARTESIAN_POINT('Ctrl Pts',(166.000000621168,-33.0335509229236,-4.15445021336676));
#62945=CARTESIAN_POINT('Ctrl Pts',(166.000000574607,-32.8828427407664,-4.43333484416701));
#62946=CARTESIAN_POINT('Ctrl Pts',(166.000000626397,-32.7173967623218,-4.70426938994011));
#62947=CARTESIAN_POINT('Ctrl Pts',(166.000000565636,-32.5382217626078,-4.96579820917569));
#62948=CARTESIAN_POINT('Ctrl Pts',(166.000000505344,-32.3604291866264,-5.22530920423366));
#62949=CARTESIAN_POINT('Ctrl Pts',(166.000000318355,-32.1691182254539,-5.47555997247503));
#62950=CARTESIAN_POINT('Ctrl Pts',(165.999999608718,-31.9652272364457,-5.71511017354509));
#62951=CARTESIAN_POINT('Ctrl Pts',(165.999999147669,-31.8327597577851,-5.87074535537798));
#62952=CARTESIAN_POINT('Ctrl Pts',(165.999998463085,-31.6949812140268,-6.02186335697795));
#62953=CARTESIAN_POINT('Ctrl Pts',(165.999997445813,-31.5521393643907,-6.16806218954705));
#62954=CARTESIAN_POINT('Ctrl Pts',(165.999996952992,-31.4829389674645,-6.23888889243354));
#62955=CARTESIAN_POINT('Ctrl Pts',(165.99999656061,-31.4126100279098,-6.30859916958569));
#62956=CARTESIAN_POINT('Ctrl Pts',(165.999996313701,-31.3411734115551,-6.37713969415401));
#62957=CARTESIAN_POINT('Ctrl Pts',(165.999995700682,-31.1638120550652,-6.54731069373769));
#62958=CARTESIAN_POINT('Ctrl Pts',(165.999996043762,-30.9796197037463,-6.71027326435898));
#62959=CARTESIAN_POINT('Ctrl Pts',(165.999996748922,-30.7892310653985,-6.86571551012216));
#62960=CARTESIAN_POINT('Ctrl Pts',(165.999997459713,-30.5973222246221,-7.0223989207025));
#62961=CARTESIAN_POINT('Ctrl Pts',(165.999998431312,-30.3991174400365,-7.17144066174681));
#62962=CARTESIAN_POINT('Ctrl Pts',(165.999999046835,-30.195313645535,-7.31249543383105));
#62963=CARTESIAN_POINT('Ctrl Pts',(165.999999670923,-29.9886740948589,-7.45551286290045));
#62964=CARTESIAN_POINT('Ctrl Pts',(165.99999993059,-29.7762784496636,-7.59031873148697));
#62965=CARTESIAN_POINT('Ctrl Pts',(165.9999999882,-29.5589050785219,-7.7165384034869));
#62966=CARTESIAN_POINT('Ctrl Pts',(166.000000035419,-29.3807341173718,-7.81999486716584));
#62967=CARTESIAN_POINT('Ctrl Pts',(166.,-29.1992199712598,-7.91768238095348));
#62968=CARTESIAN_POINT('Ctrl Pts',(166.,-29.0148173233401,-8.00939296658655));
#62969=CARTESIAN_POINT('Origin',(166.,0.,0.));
#62970=CARTESIAN_POINT('Ctrl Pts',(166.,-7.57107088371365,29.1322653714706));
#62971=CARTESIAN_POINT('Ctrl Pts',(166.,-7.83004053021588,29.3040447792896));
#62972=CARTESIAN_POINT('Ctrl Pts',(166.,-8.09758144626839,29.4628272998525));
#62973=CARTESIAN_POINT('Ctrl Pts',(166.,-8.37226172744199,29.6080560830794));
#62974=CARTESIAN_POINT('Ctrl Pts',(166.,-8.65151782958523,29.7557041914535));
#62975=CARTESIAN_POINT('Ctrl Pts',(166.,-8.93815390122485,29.8893437091684));
#62976=CARTESIAN_POINT('Ctrl Pts',(166.,-9.23069869085615,30.0083479991787));
#62977=CARTESIAN_POINT('Ctrl Pts',(166.,-9.29469045484391,30.0343792077655));
#62978=CARTESIAN_POINT('Ctrl Pts',(166.,-9.35896503860798,30.0597099793672));
#62979=CARTESIAN_POINT('Ctrl Pts',(166.,-9.42350719522099,30.0843334608256));
#62980=CARTESIAN_POINT('Ctrl Pts',(166.,-9.74517827869988,30.2070542122755));
#62981=CARTESIAN_POINT('Ctrl Pts',(166.000000159105,-10.0737946755639,30.3121083886772));
#62982=CARTESIAN_POINT('Ctrl Pts',(166.000000291074,-10.407202519014,30.3986003326446));
#62983=CARTESIAN_POINT('Ctrl Pts',(166.000000422447,-10.7391037489178,30.4847014341739));
#62984=CARTESIAN_POINT('Ctrl Pts',(166.000000483618,-11.0757521672813,30.5524085248542));
#62985=CARTESIAN_POINT('Ctrl Pts',(166.00000044277,-11.4150550043925,30.6008782566181));
#62986=CARTESIAN_POINT('Ctrl Pts',(166.000000402416,-11.750248049374,30.6487609006824));
#62987=CARTESIAN_POINT('Ctrl Pts',(166.000000290454,-12.0880309473421,30.6778704752194));
#62988=CARTESIAN_POINT('Ctrl Pts',(166.000000335807,-12.4264299076929,30.6874188265604));
#62989=CARTESIAN_POINT('Ctrl Pts',(166.000000358569,-12.5962741233494,30.6922111942516));
#62990=CARTESIAN_POINT('Ctrl Pts',(166.000000423249,-12.7662742867368,30.6920762112804));
#62991=CARTESIAN_POINT('Ctrl Pts',(166.00000051567,-12.9361857334605,30.6869152176631));
#62992=CARTESIAN_POINT('Ctrl Pts',(166.000000522059,-12.9479317733491,30.6865584363039));
#62993=CARTESIAN_POINT('Ctrl Pts',(166.00000052853,-12.9596769619201,30.6861776146853));
#62994=CARTESIAN_POINT('Ctrl Pts',(166.000000535057,-12.9714212220544,30.6857727098364));
#62995=CARTESIAN_POINT('Ctrl Pts',(166.00000069439,-13.2581246423201,30.6758880850311));
#62996=CARTESIAN_POINT('Ctrl Pts',(166.000000856491,-13.5442788051414,30.6516525281864));
#62997=CARTESIAN_POINT('Ctrl Pts',(166.000000781528,-13.8285584125716,30.6134264603938));
#62998=CARTESIAN_POINT('Ctrl Pts',(166.000000706633,-14.1125777565082,30.5752353893075));
#62999=CARTESIAN_POINT('Ctrl Pts',(166.000000393888,-14.3947261704853,30.5230782585517));
#63000=CARTESIAN_POINT('Ctrl Pts',(166.000000175973,-14.6736310564565,30.4573056218517));
#63001=CARTESIAN_POINT('Ctrl Pts',(166.000000073066,-14.8053400716992,30.4262453943497));
#63002=CARTESIAN_POINT('Ctrl Pts',(166.,-14.9363250021735,30.3921487914685));
#63003=CARTESIAN_POINT('Ctrl Pts',(166.,-15.0664372627468,30.3550531378468));
#63004=CARTESIAN_POINT('Ctrl Pts',(166.,-15.3339756489358,30.2787766112471));
#63005=CARTESIAN_POINT('Ctrl Pts',(166.000000002737,-15.5979488939222,30.1900046692378));
#63006=CARTESIAN_POINT('Ctrl Pts',(166.000000127251,-15.8571799520121,30.0890423037189));
#63007=CARTESIAN_POINT('Ctrl Pts',(166.000000250915,-16.114642444159,29.9887687391582));
#63008=CARTESIAN_POINT('Ctrl Pts',(166.000000528008,-16.3674275749598,29.8764697667499));
#63009=CARTESIAN_POINT('Ctrl Pts',(166.000000806601,-16.6143352957075,29.7524238352461));
#63010=CARTESIAN_POINT('Ctrl Pts',(166.000000970618,-16.7596980311098,29.6793938957031));
#63011=CARTESIAN_POINT('Ctrl Pts',(166.000001129098,-16.9030226986103,29.6022920556453));
#63012=CARTESIAN_POINT('Ctrl Pts',(166.00000110863,-17.0440561282011,29.5211733572009));
#63013=CARTESIAN_POINT('Ctrl Pts',(166.000001073423,-17.2866565611994,29.3816360047877));
#63014=CARTESIAN_POINT('Ctrl Pts',(166.000000588789,-17.5227450134843,29.2305789697184));
#63015=CARTESIAN_POINT('Ctrl Pts',(166.000000325308,-17.7509155586392,29.0683867660711));
#63016=CARTESIAN_POINT('Ctrl Pts',(166.000000140464,-17.9109867821582,28.9546021210574));
#63017=CARTESIAN_POINT('Ctrl Pts',(166.000000036969,-18.0671608568681,28.8353382434901));
#63018=CARTESIAN_POINT('Ctrl Pts',(166.00000003186,-18.2189526914074,28.7107432283293));
#63019=CARTESIAN_POINT('Ctrl Pts',(166.000000024651,-18.4331800449988,28.5348993797482));
#63020=CARTESIAN_POINT('Ctrl Pts',(166.000000207213,-18.6386776232607,28.3484347663679));
#63021=CARTESIAN_POINT('Ctrl Pts',(166.000000406871,-18.834763789339,28.1525130755237));
#63022=CARTESIAN_POINT('Ctrl Pts',(166.000000608185,-19.0324762725291,27.954966431707));
#63023=CARTESIAN_POINT('Ctrl Pts',(166.000000810431,-19.220619890962,27.7478055879208));
#63024=CARTESIAN_POINT('Ctrl Pts',(166.000000870095,-19.3985194120096,27.5322706373302));
#63025=CARTESIAN_POINT('Ctrl Pts',(166.000000890677,-19.4598876246811,27.457919708176));
#63026=CARTESIAN_POINT('Ctrl Pts',(166.000000895603,-19.520037068931,27.3825726630901));
#63027=CARTESIAN_POINT('Ctrl Pts',(166.000000883847,-19.5789409024478,27.3062815474031));
#63028=CARTESIAN_POINT('Ctrl Pts',(166.000000845523,-19.770965835378,27.0575745363597));
#63029=CARTESIAN_POINT('Ctrl Pts',(166.000000681352,-19.9496915008899,26.7986294338149));
#63030=CARTESIAN_POINT('Ctrl Pts',(166.000000634525,-20.1144114968969,26.53104931353));
#63031=CARTESIAN_POINT('Ctrl Pts',(166.000000587306,-20.2805107765499,26.2612286098741));
#63032=CARTESIAN_POINT('Ctrl Pts',(166.00000064022,-20.4323695370592,25.9826270218199));
#63033=CARTESIAN_POINT('Ctrl Pts',(166.00000057971,-20.5692332852037,25.6968442162162));
#63034=CARTESIAN_POINT('Ctrl Pts',(166.000000519663,-20.7050484978224,25.4132508393575));
#63035=CARTESIAN_POINT('Ctrl Pts',(166.000000331685,-20.8260981790392,25.1225850541421));
#63036=CARTESIAN_POINT('Ctrl Pts',(165.999999620488,-20.9316059215751,24.8263779294695));
#63037=CARTESIAN_POINT('Ctrl Pts',(165.999999157238,-21.0003300972392,24.6334386249249));
#63038=CARTESIAN_POINT('Ctrl Pts',(165.999998469154,-21.0624593578495,24.438147622002));
#63039=CARTESIAN_POINT('Ctrl Pts',(165.999997448035,-21.1177682304653,24.2409231385358));
#63040=CARTESIAN_POINT('Ctrl Pts',(165.999996954395,-21.1445061940382,24.1455789233094));
#63041=CARTESIAN_POINT('Ctrl Pts',(165.999996561405,-21.1697129928559,24.0498155701788));
#63042=CARTESIAN_POINT('Ctrl Pts',(165.999996314061,-21.1933528657851,23.9536778109465));
#63043=CARTESIAN_POINT('Ctrl Pts',(165.999995700107,-21.2520315470221,23.7150455244821));
#63044=CARTESIAN_POINT('Ctrl Pts',(165.999996042829,-21.3010563042592,23.4741026935237));
#63045=CARTESIAN_POINT('Ctrl Pts',(165.999996747874,-21.3404743469568,23.2315544115399));
#63046=CARTESIAN_POINT('Ctrl Pts',(165.999997458547,-21.3802069773521,22.9870703991039));
#63047=CARTESIAN_POINT('Ctrl Pts',(165.999998430315,-21.4101781211153,22.7409553237872));
#63048=CARTESIAN_POINT('Ctrl Pts',(165.999999046094,-21.4304371697983,22.4939848490062));
#63049=CARTESIAN_POINT('Ctrl Pts',(165.999999670447,-21.4509782680453,22.2435760136275));
#63050=CARTESIAN_POINT('Ctrl Pts',(165.999999930442,-21.4615341907361,21.9922880212625));
#63051=CARTESIAN_POINT('Ctrl Pts',(165.999999988173,-21.4621696368845,21.7409817270857));
#63052=CARTESIAN_POINT('Ctrl Pts',(166.000000035541,-21.462691007142,21.5347901754492));
#63053=CARTESIAN_POINT('Ctrl Pts',(166.,-21.4565341578361,21.3285874117213));
#63054=CARTESIAN_POINT('Ctrl Pts',(166.,-21.4437464396264,21.122872404884));
#63055=CARTESIAN_POINT('Origin',(155.,2.16262821021008E-15,3.7457819379656E-15));
#63056=CARTESIAN_POINT('Origin',(133.079689783217,7.42462120245876,12.8598211496117));
#63057=CARTESIAN_POINT('Ctrl Pts',(127.110025063046,18.8932088282594,-5.44956165540179));
#63058=CARTESIAN_POINT('Ctrl Pts',(126.561429499417,19.2648380810399,-1.85688406416955));
#63059=CARTESIAN_POINT('Ctrl Pts',(126.561429543109,19.2648380514426,1.85688435029735));
#63060=CARTESIAN_POINT('Ctrl Pts',(127.110025063046,18.8932088282595,5.44956165540082));
#63061=CARTESIAN_POINT('Ctrl Pts',(127.362931194533,18.7218853198324,-5.39322150128863));
#63062=CARTESIAN_POINT('Ctrl Pts',(126.820035975586,19.0896530593927,-1.83787357333886));
#63063=CARTESIAN_POINT('Ctrl Pts',(126.820036018823,19.0896530301029,1.83787385649365));
#63064=CARTESIAN_POINT('Ctrl Pts',(127.362931194533,18.7218853198325,5.39322150128767));
#63065=CARTESIAN_POINT('Ctrl Pts',(127.647218583474,18.2006252760714,-5.29589178770982));
#63066=CARTESIAN_POINT('Ctrl Pts',(127.114085169262,18.561779734697,-1.8044722430188));
#63067=CARTESIAN_POINT('Ctrl Pts',(127.114085211722,18.5617797059339,1.8044725210822));
#63068=CARTESIAN_POINT('Ctrl Pts',(127.647218583474,18.2006252760715,5.29589178770888));
#63069=CARTESIAN_POINT('Ctrl Pts',(127.47007422846,17.6499357469874,-5.26597768375926));
#63070=CARTESIAN_POINT('Ctrl Pts',(126.939976558163,18.009033107223,-1.79444248385979));
#63071=CARTESIAN_POINT('Ctrl Pts',(126.939976600381,18.0090330786238,1.79444276033958));
#63072=CARTESIAN_POINT('Ctrl Pts',(127.47007422846,17.6499357469875,5.26597768375833));
#63073=CARTESIAN_POINT('Ctrl Pts',(127.328278974586,17.4651063902315,-5.26851068351905));
#63074=CARTESIAN_POINT('Ctrl Pts',(126.797908769233,17.8243882174352,-1.79519250829358));
#63075=CARTESIAN_POINT('Ctrl Pts',(126.797908811472,17.8243881888213,1.79519278491536));
#63076=CARTESIAN_POINT('Ctrl Pts',(127.328278974586,17.4651063902316,5.26851068351812));
#63077=CARTESIAN_POINT('',(127.464921070561,17.9352463278168,-4.90283862543942));
#63078=CARTESIAN_POINT('Ctrl Pts',(127.464921070561,17.9352463278168,-4.90283862543941));
#63079=CARTESIAN_POINT('Ctrl Pts',(127.45225052721,17.7646936285484,-5.01023372772536));
#63080=CARTESIAN_POINT('Ctrl Pts',(127.404564208301,17.6055373983108,-5.13497641413359));
#63081=CARTESIAN_POINT('Ctrl Pts',(127.329689952113,17.4676849997989,-5.26605170523142));
#63082=CARTESIAN_POINT('Ctrl Pts',(127.328985684036,17.4663947479232,-5.26728090519197));
#63083=CARTESIAN_POINT('Ctrl Pts',(127.328278974586,17.4651063902315,-5.26851068351905));
#63084=CARTESIAN_POINT('',(126.797085404885,19.1052002095942,-2.68667180544493));
#63085=CARTESIAN_POINT('Ctrl Pts',(126.797085404885,19.1052002095942,-2.68667180544497));
#63086=CARTESIAN_POINT('Ctrl Pts',(126.969476253353,18.9884193122445,-3.27478906922211));
#63087=CARTESIAN_POINT('Ctrl Pts',(127.153613972947,18.8183199434291,-3.7599139578563));
#63088=CARTESIAN_POINT('Ctrl Pts',(127.375160466542,18.4547272249797,-4.40330387330635));
#63089=CARTESIAN_POINT('Ctrl Pts',(127.435582157733,18.2965217635359,-4.60168518403203));
#63090=CARTESIAN_POINT('Ctrl Pts',(127.46744820753,18.0691174589434,-4.80945859098079));
#63091=CARTESIAN_POINT('Ctrl Pts',(127.469817708987,18.0011578580281,-4.86133488167436));
#63092=CARTESIAN_POINT('Ctrl Pts',(127.464921070561,17.9352463278168,-4.90283862543942));
#63093=CARTESIAN_POINT('',(126.797085404885,19.1052002095942,2.68667180544505));
#63094=CARTESIAN_POINT('Ctrl Pts',(126.797739723097,19.1047569617733,-2.68660115054962));
#63095=CARTESIAN_POINT('Ctrl Pts',(126.665524631944,19.1943220235221,-0.900309345120119));
#63096=CARTESIAN_POINT('Ctrl Pts',(126.665524637164,19.1943220199857,0.900309413191638));
#63097=CARTESIAN_POINT('Ctrl Pts',(126.79773972325,19.1047569616696,2.68660115053324));
#63098=CARTESIAN_POINT('',(127.464921070561,17.9352463278167,4.90283862543941));
#63099=CARTESIAN_POINT('Ctrl Pts',(126.797085404885,19.1052002095942,2.68667180544503));
#63100=CARTESIAN_POINT('Ctrl Pts',(126.91366890947,19.0262242871335,3.08440041068748));
#63101=CARTESIAN_POINT('Ctrl Pts',(127.036713649653,18.9228672387061,3.43736008146732));
#63102=CARTESIAN_POINT('Ctrl Pts',(127.242196284738,18.6805750668838,4.0184756344589));
#63103=CARTESIAN_POINT('Ctrl Pts',(127.322999453864,18.5537833666843,4.24389900144219));
#63104=CARTESIAN_POINT('Ctrl Pts',(127.427486245652,18.303787089057,4.58633594558102));
#63105=CARTESIAN_POINT('Ctrl Pts',(127.456769006299,18.1859058434825,4.71065867847017));
#63106=CARTESIAN_POINT('Ctrl Pts',(127.468025474849,18.0271746270173,4.84035139768563));
#63107=CARTESIAN_POINT('Ctrl Pts',(127.468398492744,17.9820544025211,4.87336411115589));
#63108=CARTESIAN_POINT('Ctrl Pts',(127.464921070561,17.9352463278168,4.90283862543944));
#63109=CARTESIAN_POINT('Ctrl Pts',(127.464921070561,17.9352463278167,4.90283862543944));
#63110=CARTESIAN_POINT('Ctrl Pts',(127.45225052721,17.7646936285574,5.01023372771974));
#63111=CARTESIAN_POINT('Ctrl Pts',(127.404564208346,17.6055373983733,5.13497641412251));
#63112=CARTESIAN_POINT('Ctrl Pts',(127.329689952112,17.4676849997981,5.26605170523029));
#63113=CARTESIAN_POINT('Ctrl Pts',(127.328985684037,17.4663947479244,5.26728090519003));
#63114=CARTESIAN_POINT('Ctrl Pts',(127.328278974586,17.4651063902316,5.26851068351812));
#63115=CARTESIAN_POINT('Ctrl Pts',(127.223161057304,17.637333484571,4.84740014651676));
#63116=CARTESIAN_POINT('Ctrl Pts',(129.536338162963,20.5271470899125,5.38268796752789));
#63117=CARTESIAN_POINT('Ctrl Pts',(136.262411348692,26.2301344742948,6.5934772821786));
#63118=CARTESIAN_POINT('Ctrl Pts',(145.009334199428,28.5361317066653,7.37677649719925));
#63119=CARTESIAN_POINT('Ctrl Pts',(150.052765342883,28.5386902383977,7.65589740262126));
#63120=CARTESIAN_POINT('Ctrl Pts',(127.284956078127,17.5615992796209,4.9703901080484));
#63121=CARTESIAN_POINT('Ctrl Pts',(129.605785359691,20.4274443154497,5.51440627868322));
#63122=CARTESIAN_POINT('Ctrl Pts',(136.344308947184,26.0580483552802,6.73748831063584));
#63123=CARTESIAN_POINT('Ctrl Pts',(145.047721144709,28.2686618330716,7.49952020714348));
#63124=CARTESIAN_POINT('Ctrl Pts',(150.04110192192,28.2301731145178,7.75403475399863));
#63125=CARTESIAN_POINT('Ctrl Pts',(127.321297410279,17.5020569846164,5.11597630585223));
#63126=CARTESIAN_POINT('Ctrl Pts',(129.646063017966,20.3503306845444,5.67750153574081));
#63127=CARTESIAN_POINT('Ctrl Pts',(136.391076354387,25.9286703820878,6.94240078127363));
#63128=CARTESIAN_POINT('Ctrl Pts',(145.066397536241,28.0592476051524,7.73980152246514));
#63129=CARTESIAN_POINT('Ctrl Pts',(150.020700025828,27.9774063873195,8.01119722834055));
#63130=CARTESIAN_POINT('Ctrl Pts',(127.328278974586,17.4651063902316,5.26851068351813));
#63131=CARTESIAN_POINT('Ctrl Pts',(129.65180814865,20.3057906140435,5.85030184552965));
#63132=CARTESIAN_POINT('Ctrl Pts',(136.392549858192,25.8653195016249,7.16627842882971));
#63133=CARTESIAN_POINT('Ctrl Pts',(145.055988202077,27.9753679280423,8.01762643953326));
#63134=CARTESIAN_POINT('Ctrl Pts',(150.,27.884960655152,8.32099568925642));
#63135=CARTESIAN_POINT('',(127.849160658777,18.3925040698363,4.98892391726874));
#63136=CARTESIAN_POINT('Ctrl Pts',(127.849242092347,18.392458062281,4.98880236862972));
#63137=CARTESIAN_POINT('Ctrl Pts',(130.048410754748,20.9540078872094,5.4737346990744));
#63138=CARTESIAN_POINT('Ctrl Pts',(136.593491210251,26.3174187978766,6.62312594835455));
#63139=CARTESIAN_POINT('Ctrl Pts',(145.009334199428,28.5361317066653,7.37677649719925));
#63140=CARTESIAN_POINT('Ctrl Pts',(150.052765342883,28.5386902383977,7.65589740262126));
#63141=CARTESIAN_POINT('Ctrl Pts',(127.849242092347,18.392458062281,4.98880236862972));
#63142=CARTESIAN_POINT('Ctrl Pts',(127.719533880909,18.2413764049341,4.96020078552886));
#63143=CARTESIAN_POINT('Ctrl Pts',(127.591421464243,18.0889606117714,4.93153597886479));
#63144=CARTESIAN_POINT('Ctrl Pts',(127.464935664785,17.9352383975679,4.90281760981468));
#63145=CARTESIAN_POINT('Origin',(165.,29.0148173233401,-8.00939296658656));
#63146=CARTESIAN_POINT('',(165.,28.05086990396,-7.74330017699896));
#63147=CARTESIAN_POINT('Origin',(165.,29.0148173233401,-8.00939296658656));
#63148=CARTESIAN_POINT('Origin',(165.,29.0148173233401,-8.00939296658656));
#63149=CARTESIAN_POINT('Origin',(165.,0.,0.));
#63150=CARTESIAN_POINT('',(165.,20.731329614394,-20.4211158465778));
#63151=CARTESIAN_POINT('Origin',(165.,0.,0.));
#63152=CARTESIAN_POINT('Origin',(165.,21.4437464396309,-21.1228724048794));
#63153=CARTESIAN_POINT('Ctrl Pts',(164.848300728223,28.5746646574706,-7.12437716917367));
#63154=CARTESIAN_POINT('Ctrl Pts',(163.482308912768,28.5466253347185,-7.3724648834928));
#63155=CARTESIAN_POINT('Ctrl Pts',(160.687181858131,28.5326138897007,-7.66261315463168));
#63156=CARTESIAN_POINT('Ctrl Pts',(155.726343237302,28.5490214348333,-7.8189699002432));
#63157=CARTESIAN_POINT('Ctrl Pts',(152.168940472788,28.539712686299,-7.7730294750179));
#63158=CARTESIAN_POINT('Ctrl Pts',(150.052788176347,28.5386902497055,-7.65589866638835));
#63159=CARTESIAN_POINT('Ctrl Pts',(164.886050420652,28.3206281744635,-7.24424874059928));
#63160=CARTESIAN_POINT('Ctrl Pts',(163.5093195108,28.2726747615687,-7.48712183418305));
#63161=CARTESIAN_POINT('Ctrl Pts',(160.69940197879,28.2254086627087,-7.76242949758385));
#63162=CARTESIAN_POINT('Ctrl Pts',(155.727018894895,28.2140262371482,-7.90031199476649));
#63163=CARTESIAN_POINT('Ctrl Pts',(152.164256486615,28.2149411370325,-7.86212823426182));
#63164=CARTESIAN_POINT('Ctrl Pts',(150.041115769415,28.2301726485455,-7.75403551841943));
#63165=CARTESIAN_POINT('Ctrl Pts',(164.942784454705,28.1247340937978,-7.47571985177044));
#63166=CARTESIAN_POINT('Ctrl Pts',(163.552552248986,28.0572384132519,-7.72923456433801));
#63167=CARTESIAN_POINT('Ctrl Pts',(160.721537840974,27.9750232050359,-8.0193615297205));
#63168=CARTESIAN_POINT('Ctrl Pts',(155.728550806707,27.9313779407873,-8.16788990633514));
#63169=CARTESIAN_POINT('Ctrl Pts',(152.155069764412,27.944319466443,-8.12603160012519));
#63170=CARTESIAN_POINT('Ctrl Pts',(150.020705033617,27.9774056214107,-8.01119817466015));
#63171=CARTESIAN_POINT('Ctrl Pts',(165.,28.05086990396,-7.74330017699896));
#63172=CARTESIAN_POINT('Ctrl Pts',(163.596244720614,27.9764371287996,-8.01294025873278));
#63173=CARTESIAN_POINT('Ctrl Pts',(160.744041400418,27.8833028642094,-8.32829486530623));
#63174=CARTESIAN_POINT('Ctrl Pts',(155.730107343147,27.8315724021945,-8.49823494388704));
#63175=CARTESIAN_POINT('Ctrl Pts',(152.145723085267,27.8469714367605,-8.44830349102718));
#63176=CARTESIAN_POINT('Ctrl Pts',(150.,27.884960245299,-8.32099706273788));
#63177=CARTESIAN_POINT('',(150.052788176347,28.5386902497055,-7.65589866638835));
#63178=CARTESIAN_POINT('Ctrl Pts',(164.848300728223,28.5746646574706,-7.12437716917367));
#63179=CARTESIAN_POINT('Ctrl Pts',(163.482308912768,28.5466253347185,-7.3724648834928));
#63180=CARTESIAN_POINT('Ctrl Pts',(160.687181858131,28.5326138897007,-7.66261315463168));
#63181=CARTESIAN_POINT('Ctrl Pts',(155.726343237302,28.5490214348333,-7.8189699002432));
#63182=CARTESIAN_POINT('Ctrl Pts',(152.168940472788,28.539712686299,-7.7730294750179));
#63183=CARTESIAN_POINT('Ctrl Pts',(150.052788176347,28.5386902497055,-7.65589866638835));
#63184=CARTESIAN_POINT('Origin',(150.,28.8432063018385,-8.60694197898317));
#63185=CARTESIAN_POINT('Ctrl Pts',(150.,27.884960245299,-8.32099706273788));
#63186=CARTESIAN_POINT('Ctrl Pts',(152.145723085267,27.8469714367605,-8.44830349102718));
#63187=CARTESIAN_POINT('Ctrl Pts',(155.730107343147,27.8315724021945,-8.49823494388704));
#63188=CARTESIAN_POINT('Ctrl Pts',(160.744041400418,27.8833028642094,-8.32829486530623));
#63189=CARTESIAN_POINT('Ctrl Pts',(163.596244720614,27.9764371287996,-8.01294025873278));
#63190=CARTESIAN_POINT('Ctrl Pts',(165.,28.05086990396,-7.74330017699896));
#63191=CARTESIAN_POINT('Ctrl Pts',(150.052788176357,28.5386902499724,-7.65589866630348));
#63192=CARTESIAN_POINT('Ctrl Pts',(146.27021147609,28.5367742688787,-7.44655817015133));
#63193=CARTESIAN_POINT('Ctrl Pts',(137.492208043054,26.8239638200099,-6.7460042044279));
#63194=CARTESIAN_POINT('Ctrl Pts',(130.307399857886,21.4904216144153,-5.56111785667491));
#63195=CARTESIAN_POINT('Ctrl Pts',(127.223161057304,17.6373334845711,-4.84740014651678));
#63196=CARTESIAN_POINT('Ctrl Pts',(150.041124530135,28.2301729428908,-7.75403591045255));
#63197=CARTESIAN_POINT('Ctrl Pts',(146.296085688665,28.2590423920148,-7.56315022378985));
#63198=CARTESIAN_POINT('Ctrl Pts',(137.573659592423,26.6369374470922,-6.88981462845168));
#63199=CARTESIAN_POINT('Ctrl Pts',(130.379397788713,21.3827292892224,-5.69574562774071));
#63200=CARTESIAN_POINT('Ctrl Pts',(127.284956078127,17.5615992796211,-4.97039010804842));
#63201=CARTESIAN_POINT('Ctrl Pts',(150.020722457357,27.9774060201304,-8.01119846063586));
#63202=CARTESIAN_POINT('Ctrl Pts',(146.304992407366,28.0387898627464,-7.80765190139207));
#63203=CARTESIAN_POINT('Ctrl Pts',(137.620830210905,26.4966944406706,-7.10057757041368));
#63204=CARTESIAN_POINT('Ctrl Pts',(130.420987560222,21.2997585261465,-5.8646772580149));
#63205=CARTESIAN_POINT('Ctrl Pts',(127.32129741028,17.5020569846165,-5.11597630585225));
#63206=CARTESIAN_POINT('Ctrl Pts',(150.000022383365,27.8849602458363,-8.32099706271973));
#63207=CARTESIAN_POINT('Ctrl Pts',(146.292010366753,27.9527686296717,-8.09347032423286));
#63208=CARTESIAN_POINT('Ctrl Pts',(137.621356760532,26.4299654695285,-7.33205606798856));
#63209=CARTESIAN_POINT('Ctrl Pts',(130.426320544944,21.2526886215472,-6.04423290181325));
#63210=CARTESIAN_POINT('Ctrl Pts',(127.328278974586,17.4651063902317,-5.26851068351815));
#63211=CARTESIAN_POINT('',(127.849160658792,18.3925040698507,-4.98892391727468));
#63212=CARTESIAN_POINT('Ctrl Pts',(150.052788176357,28.5386902499724,-7.65589866630348));
#63213=CARTESIAN_POINT('Ctrl Pts',(146.27021147609,28.5367742688787,-7.44655817015133));
#63214=CARTESIAN_POINT('Ctrl Pts',(137.824484209527,26.8887993027237,-6.77252246543263));
#63215=CARTESIAN_POINT('Ctrl Pts',(130.853619721487,21.8890176410856,-5.65012752561999));
#63216=CARTESIAN_POINT('Ctrl Pts',(127.849390961495,18.3923448905147,-4.98871937797766));
#63217=CARTESIAN_POINT('Ctrl Pts',(127.849390961495,18.3923448905147,-4.98871937797766));
#63218=CARTESIAN_POINT('Ctrl Pts',(127.719628878171,18.2413126033397,-4.96015108107934));
#63219=CARTESIAN_POINT('Ctrl Pts',(127.591474210876,18.0889296686807,-4.93151009034075));
#63220=CARTESIAN_POINT('Ctrl Pts',(127.464959837491,17.9352208155325,-4.90280437755726));
#63221=CARTESIAN_POINT('Ctrl Pts',(150.052788176347,20.8995478587445,-20.8872814137861));
#63222=CARTESIAN_POINT('Ctrl Pts',(152.168660886943,21.0014838633252,-20.8296090862044));
#63223=CARTESIAN_POINT('Ctrl Pts',(155.727583550824,21.0459254437713,-20.8146988140623));
#63224=CARTESIAN_POINT('Ctrl Pts',(160.688246103924,20.9022416184807,-20.8787128106776));
#63225=CARTESIAN_POINT('Ctrl Pts',(163.482347522152,20.6580488685503,-21.0358744828481));
#63226=CARTESIAN_POINT('Ctrl Pts',(164.848300728212,20.4572239433831,-21.184196913403));
#63227=CARTESIAN_POINT('Ctrl Pts',(150.041115769415,20.8302780650708,-20.5710289076513));
#63228=CARTESIAN_POINT('Ctrl Pts',(152.16397597746,20.9162619855092,-20.5038005571989));
#63229=CARTESIAN_POINT('Ctrl Pts',(155.728261756486,20.9488744436001,-20.4839145541437));
#63230=CARTESIAN_POINT('Ctrl Pts',(160.700470758148,20.8350936776417,-20.562764456785));
#63231=CARTESIAN_POINT('Ctrl Pts',(163.509358423722,20.6203698230701,-20.7412982655356));
#63232=CARTESIAN_POINT('Ctrl Pts',(164.886050420642,20.4340175279256,-20.9042590799178));
#63233=CARTESIAN_POINT('Ctrl Pts',(150.020705033617,20.9266039447125,-20.2235449127931));
#63234=CARTESIAN_POINT('Ctrl Pts',(152.154787772342,21.0094985774067,-20.1374861209271));
#63235=CARTESIAN_POINT('Ctrl Pts',(155.729798323956,21.0392800208202,-20.1053474704887));
#63236=CARTESIAN_POINT('Ctrl Pts',(160.722613371139,20.9324125083846,-20.2174719595082));
#63237=CARTESIAN_POINT('Ctrl Pts',(163.552591543519,20.7223274394986,-20.4336691786634));
#63238=CARTESIAN_POINT('Ctrl Pts',(164.942784454694,20.5365303501092,-20.6188742740246));
#63239=CARTESIAN_POINT('Ctrl Pts',(150.,21.1486749637962,-19.9885854245792));
#63240=CARTESIAN_POINT('Ctrl Pts',(152.145439592532,21.2399191037303,-19.8920456936864));
#63241=CARTESIAN_POINT('Ctrl Pts',(155.731359600689,21.2754632200757,-19.8537421157224));
#63242=CARTESIAN_POINT('Ctrl Pts',(160.745123738616,21.154090253261,-19.9835809301406));
#63243=CARTESIAN_POINT('Ctrl Pts',(163.596284397372,20.9276228391379,-20.2218407641675));
#63244=CARTESIAN_POINT('Ctrl Pts',(164.999999999989,20.7313296143911,-20.4211158465807));
#63245=CARTESIAN_POINT('',(164.84830072822,20.4572239433771,-21.184196913325));
#63246=CARTESIAN_POINT('Origin',(164.999999999989,21.4437464396279,-21.1228724048824));
#63247=CARTESIAN_POINT('Ctrl Pts',(164.999999999989,20.7313296143911,-20.4211158465807));
#63248=CARTESIAN_POINT('Ctrl Pts',(163.596284397372,20.9276228391379,-20.2218407641675));
#63249=CARTESIAN_POINT('Ctrl Pts',(160.745123738616,21.154090253261,-19.9835809301406));
#63250=CARTESIAN_POINT('Ctrl Pts',(155.731359600689,21.2754632200757,-19.8537421157224));
#63251=CARTESIAN_POINT('Ctrl Pts',(152.145439592532,21.2399191037303,-19.8920456936864));
#63252=CARTESIAN_POINT('Ctrl Pts',(150.,21.1486749637962,-19.9885854245792));
#63253=CARTESIAN_POINT('',(150.052788176347,20.8995478587445,-20.8872814137861));
#63254=CARTESIAN_POINT('Origin',(150.,21.8754335536174,-20.675478394496));
#63255=CARTESIAN_POINT('Ctrl Pts',(150.052788176347,20.8995478587445,-20.8872814137861));
#63256=CARTESIAN_POINT('Ctrl Pts',(152.168660886943,21.0014838633252,-20.8296090862044));
#63257=CARTESIAN_POINT('Ctrl Pts',(155.727583550824,21.0459254437713,-20.8146988140623));
#63258=CARTESIAN_POINT('Ctrl Pts',(160.688246103924,20.9022416184807,-20.8787128106776));
#63259=CARTESIAN_POINT('Ctrl Pts',(163.482347522152,20.6580488685503,-21.0358744828481));
#63260=CARTESIAN_POINT('Ctrl Pts',(164.848300728212,20.4572239433831,-21.184196913403));
#63261=CARTESIAN_POINT('Ctrl Pts',(150.000022383365,21.1486749640491,-19.9885854250535));
#63262=CARTESIAN_POINT('Ctrl Pts',(146.292010364483,20.9855352202971,-20.1610725773936));
#63263=CARTESIAN_POINT('Ctrl Pts',(137.621314702792,19.5648105010924,-19.2230426666662));
#63264=CARTESIAN_POINT('Ctrl Pts',(130.426320557839,15.8608035608144,-15.3832518061148));
#63265=CARTESIAN_POINT('Ctrl Pts',(127.328278974581,13.2952172871479,-12.4909704719746));
#63266=CARTESIAN_POINT('Ctrl Pts',(150.020722457357,20.9266043917346,-20.2235451151067));
#63267=CARTESIAN_POINT('Ctrl Pts',(146.304992405091,20.7810198217954,-20.3784783619108));
#63268=CARTESIAN_POINT('Ctrl Pts',(137.620776912509,19.3976728561079,-19.3965609996052));
#63269=CARTESIAN_POINT('Ctrl Pts',(130.420987573124,15.7288387641155,-15.5137933612435));
#63270=CARTESIAN_POINT('Ctrl Pts',(127.321297410274,13.1815939383312,-12.5992378142297));
#63271=CARTESIAN_POINT('Ctrl Pts',(150.041124530135,20.8302785517541,-20.5710289665453));
#63272=CARTESIAN_POINT('Ctrl Pts',(146.296085686372,20.6794014223549,-20.691473486285));
#63273=CARTESIAN_POINT('Ctrl Pts',(137.57360659547,19.2852642849739,-19.6233996678108));
#63274=CARTESIAN_POINT('Ctrl Pts',(130.379397801594,15.6240250622979,-15.6701139651087));
#63275=CARTESIAN_POINT('Ctrl Pts',(127.284956078122,13.085283740095,-12.7235960532051));
#63276=CARTESIAN_POINT('Ctrl Pts',(150.052788176357,20.8995478588044,-20.8872814140596));
#63277=CARTESIAN_POINT('Ctrl Pts',(146.270211473774,20.7172956804373,-20.9902923738985));
#63278=CARTESIAN_POINT('Ctrl Pts',(137.492160038669,19.2542660948038,-19.857274979511));
#63279=CARTESIAN_POINT('Ctrl Pts',(130.307399870724,15.561280155121,-15.8306921401907));
#63280=CARTESIAN_POINT('Ctrl Pts',(127.223161057299,13.0166384114731,-12.850678779393));
#63281=CARTESIAN_POINT('',(127.464921070561,13.2136059641945,-13.0809596303012));
#63282=CARTESIAN_POINT('Ctrl Pts',(127.464921070561,13.2136059641945,-13.0809596303012));
#63283=CARTESIAN_POINT('Ctrl Pts',(127.452250527049,13.2213365014801,-12.8795591063511));
#63284=CARTESIAN_POINT('Ctrl Pts',(127.404564207044,13.2497887223202,-12.679354421998));
#63285=CARTESIAN_POINT('Ctrl Pts',(127.329689950212,13.2943770554065,-12.4944330978374));
#63286=CARTESIAN_POINT('Ctrl Pts',(127.328985683081,13.2947964472952,-12.4927011092939));
#63287=CARTESIAN_POINT('Ctrl Pts',(127.328278974586,13.295217287153,-12.4909704719789));
#63288=CARTESIAN_POINT('Ctrl Pts',(127.464959760394,13.2135636128086,-13.0809546870724));
#63289=CARTESIAN_POINT('Ctrl Pts',(130.520511156931,15.6701515076247,-15.9492967987681));
#63290=CARTESIAN_POINT('Ctrl Pts',(137.622132063752,19.2759284101145,-19.8740509765864));
#63291=CARTESIAN_POINT('Ctrl Pts',(146.270211473774,20.7172956804373,-20.9902923738985));
#63292=CARTESIAN_POINT('Ctrl Pts',(150.052788176357,20.8995478588044,-20.8872814140596));
#63293=CARTESIAN_POINT('Origin',(165.,21.4437464396263,-21.1228724048825));
#63294=CARTESIAN_POINT('Origin',(165.,21.4437464396263,-21.1228724048825));
#63295=CARTESIAN_POINT('Origin',(155.,4.32525642042015E-15,0.));
#63296=CARTESIAN_POINT('Origin',(133.079689783217,14.8492424049175,-1.48211107611438E-15));
#63297=CARTESIAN_POINT('Ctrl Pts',(164.848300728225,20.4572239433763,-21.1841969133252));
#63298=CARTESIAN_POINT('Ctrl Pts',(164.823285605772,20.5140374352135,-22.0362707934334));
#63299=CARTESIAN_POINT('Ctrl Pts',(164.759348570311,20.3154311261922,-24.6124011045103));
#63300=CARTESIAN_POINT('Ctrl Pts',(164.707290846802,17.9816466348386,-28.4204658566965));
#63301=CARTESIAN_POINT('Ctrl Pts',(164.727957731471,12.955232863113,-30.2918070911266));
#63302=CARTESIAN_POINT('Ctrl Pts',(164.798266641052,9.53657145362637,-29.259124812672));
#63303=CARTESIAN_POINT('Ctrl Pts',(164.848300728223,8.11744071408901,-28.3085740825778));
#63304=CARTESIAN_POINT('Ctrl Pts',(165.010504706335,20.4323775670778,-21.1857414212518));
#63305=CARTESIAN_POINT('Ctrl Pts',(164.987238619141,20.4845624632464,-22.0356216477319));
#63306=CARTESIAN_POINT('Ctrl Pts',(164.927238219583,20.2738925189318,-24.6009637976532));
#63307=CARTESIAN_POINT('Ctrl Pts',(164.877329245491,17.9446387756182,-28.3773780702233));
#63308=CARTESIAN_POINT('Ctrl Pts',(164.897259516306,12.9567274422478,-30.239877972682));
#63309=CARTESIAN_POINT('Ctrl Pts',(164.96396895833,9.55116136467888,-29.228168072911));
#63310=CARTESIAN_POINT('Ctrl Pts',(165.010504706333,8.13120148533912,-28.2878287434741));
#63311=CARTESIAN_POINT('Ctrl Pts',(165.34664366636,20.464367539104,-21.1837528509761));
#63312=CARTESIAN_POINT('Ctrl Pts',(165.32930328867,20.5099684897007,-22.0372047173979));
#63313=CARTESIAN_POINT('Ctrl Pts',(165.28395294769,20.279032164069,-24.6075978058809));
#63314=CARTESIAN_POINT('Ctrl Pts',(165.245038300777,17.9353899642948,-28.3689599675015));
#63315=CARTESIAN_POINT('Ctrl Pts',(165.260697889921,12.9613040248117,-30.235097428672));
#63316=CARTESIAN_POINT('Ctrl Pts',(165.311960247537,9.54621541444455,-29.2470452264155));
#63317=CARTESIAN_POINT('Ctrl Pts',(165.346643666359,8.11348434695059,-28.3145385867769));
#63318=CARTESIAN_POINT('Ctrl Pts',(165.840925930751,20.7907716131771,-21.1634628226183));
#63319=CARTESIAN_POINT('Ctrl Pts',(165.836033373262,20.8363258337756,-22.0492227143231));
#63320=CARTESIAN_POINT('Ctrl Pts',(165.823057804221,20.5908898164857,-24.7182659833104));
#63321=CARTESIAN_POINT('Ctrl Pts',(165.811521565886,18.1475857625388,-28.6271012887801));
#63322=CARTESIAN_POINT('Ctrl Pts',(165.816211733742,12.9727034529567,-30.5715985406038));
#63323=CARTESIAN_POINT('Ctrl Pts',(165.831140064288,9.42145186987588,-29.5518039938382));
#63324=CARTESIAN_POINT('Ctrl Pts',(165.84092593075,7.93271062991528,-28.5870677926455));
#63325=CARTESIAN_POINT('Ctrl Pts',(166.,21.1980658637566,-21.1381444747462));
#63326=CARTESIAN_POINT('Ctrl Pts',(166.000094314236,21.2519419527489,-22.0636451239711));
#63327=CARTESIAN_POINT('Ctrl Pts',(166.000254963943,21.0127093233117,-24.8616125503296));
#63328=CARTESIAN_POINT('Ctrl Pts',(166.000465818828,18.4514877713092,-28.9930318844147));
#63329=CARTESIAN_POINT('Ctrl Pts',(166.000340749714,12.982336781343,-31.04038024057));
#63330=CARTESIAN_POINT('Ctrl Pts',(166.000188642958,9.2563942020979,-29.9460308031277));
#63331=CARTESIAN_POINT('Ctrl Pts',(166.,7.70713717218925,-28.9271357865293));
#63332=CARTESIAN_POINT('Ctrl Pts',(166.,21.4437464396209,-21.1228724047961));
#63333=CARTESIAN_POINT('Ctrl Pts',(166.,21.5027712616354,-22.0724000267995));
#63334=CARTESIAN_POINT('Ctrl Pts',(166.,21.2677585367984,-24.9482212131057));
#63335=CARTESIAN_POINT('Ctrl Pts',(166.,18.6355842566287,-29.2146519968295));
#63336=CARTESIAN_POINT('Ctrl Pts',(166.,12.9880322538084,-31.3241061902595));
#63337=CARTESIAN_POINT('Ctrl Pts',(166.,9.15679791884385,-30.1841077581618));
#63338=CARTESIAN_POINT('Ctrl Pts',(166.,7.57107088371363,-29.1322653714706));
#63339=CARTESIAN_POINT('',(164.848300728223,8.11744071408902,-28.3085740825778));
#63340=CARTESIAN_POINT('Ctrl Pts',(164.848300728225,20.4572239433763,-21.1841969133252));
#63341=CARTESIAN_POINT('Ctrl Pts',(164.823285605772,20.5140374352135,-22.0362707934334));
#63342=CARTESIAN_POINT('Ctrl Pts',(164.759348570311,20.3154311261922,-24.6124011045103));
#63343=CARTESIAN_POINT('Ctrl Pts',(164.707290846802,17.9816466348386,-28.4204658566965));
#63344=CARTESIAN_POINT('Ctrl Pts',(164.727957731471,12.955232863113,-30.2918070911266));
#63345=CARTESIAN_POINT('Ctrl Pts',(164.798266641052,9.53657145362637,-29.259124812672));
#63346=CARTESIAN_POINT('Ctrl Pts',(164.848300728223,8.11744071408901,-28.3085740825778));
#63347=CARTESIAN_POINT('Origin',(165.,7.57107088371364,-29.1322653714706));
#63348=CARTESIAN_POINT('Ctrl Pts',(150.052788176347,-7.63914239096107,-28.5431800801744));
#63349=CARTESIAN_POINT('Ctrl Pts',(152.874076212133,-7.50458485274219,-28.6224409166393));
#63350=CARTESIAN_POINT('Ctrl Pts',(157.868876345628,-7.48949828100636,-28.638002969206));
#63351=CARTESIAN_POINT('Ctrl Pts',(162.799280555694,-7.77413039070069,-28.4582180894563));
#63352=CARTESIAN_POINT('Ctrl Pts',(164.848300728637,-8.11744071415836,-28.3085740825475));
#63353=CARTESIAN_POINT('Ctrl Pts',(150.041115769415,-7.39989458347471,-28.3250644260708));
#63354=CARTESIAN_POINT('Ctrl Pts',(152.871720879359,-7.26493740563922,-28.3795336071373));
#63355=CARTESIAN_POINT('Ctrl Pts',(157.870872869895,-7.25091052196209,-28.3876462749622));
#63356=CARTESIAN_POINT('Ctrl Pts',(162.820921351418,-7.53513861733173,-28.2683712282885));
#63357=CARTESIAN_POINT('Ctrl Pts',(164.886050421069,-7.88661064661032,-28.148507820494));
#63358=CARTESIAN_POINT('Ctrl Pts',(150.020705033617,-7.05080167669813,-28.2347430874533));
#63359=CARTESIAN_POINT('Ctrl Pts',(152.86627417773,-6.89615963506482,-28.273090727713));
#63360=CARTESIAN_POINT('Ctrl Pts',(157.876626552382,-6.87707398187386,-28.2763380295735));
#63361=CARTESIAN_POINT('Ctrl Pts',(162.857403120944,-7.20825069413645,-28.1970523218162));
#63362=CARTESIAN_POINT('Ctrl Pts',(164.942784455126,-7.58820374376682,-28.0945941257757));
#63363=CARTESIAN_POINT('Ctrl Pts',(150.,-6.73628528150283,-28.3095824873171));
#63364=CARTESIAN_POINT('Ctrl Pts',(152.860712283684,-6.56397377653139,-28.3505841324417));
#63365=CARTESIAN_POINT('Ctrl Pts',(157.882563565661,-6.5403695981628,-28.3550152737227));
#63366=CARTESIAN_POINT('Ctrl Pts',(162.894333734494,-6.91343653590341,-28.2699567450454));
#63367=CARTESIAN_POINT('Ctrl Pts',(165.000000000425,-7.31954028965235,-28.1644160235599));
#63368=CARTESIAN_POINT('',(164.848300728339,-8.11744071668738,-28.3085740842798));
#63369=CARTESIAN_POINT('',(164.948224876581,-7.57107088371367,-28.1336066026236));
#63370=CARTESIAN_POINT('Origin',(165.000000000425,-7.57107088379848,-29.1322653714485));
#63371=CARTESIAN_POINT('',(165.000000000213,-7.31954028965235,-28.1644160235599));
#63372=CARTESIAN_POINT('Origin',(165.000000000425,-7.57107088379848,-29.1322653714485));
#63373=CARTESIAN_POINT('Ctrl Pts',(165.000000000425,-7.31954028965235,-28.1644160235599));
#63374=CARTESIAN_POINT('Ctrl Pts',(162.894333734494,-6.91343653590341,-28.2699567450454));
#63375=CARTESIAN_POINT('Ctrl Pts',(157.882563565661,-6.5403695981628,-28.3550152737227));
#63376=CARTESIAN_POINT('Ctrl Pts',(152.860712283684,-6.56397377653139,-28.3505841324417));
#63377=CARTESIAN_POINT('Ctrl Pts',(150.,-6.73628528150283,-28.3095824873171));
#63378=CARTESIAN_POINT('',(150.052788176347,-7.63914239096107,-28.5431800801744));
#63379=CARTESIAN_POINT('Origin',(150.,-6.96777274822114,-29.2824203734792));
#63380=CARTESIAN_POINT('Ctrl Pts',(150.052788176347,-7.63914239096107,-28.5431800801744));
#63381=CARTESIAN_POINT('Ctrl Pts',(152.874076212133,-7.50458485274219,-28.6224409166393));
#63382=CARTESIAN_POINT('Ctrl Pts',(157.868876345628,-7.48949828100636,-28.638002969206));
#63383=CARTESIAN_POINT('Ctrl Pts',(162.799280555694,-7.77413039070069,-28.4582180894563));
#63384=CARTESIAN_POINT('Ctrl Pts',(164.848300728637,-8.11744071415836,-28.3085740825475));
#63385=CARTESIAN_POINT('Origin',(165.,-7.57107088371367,-29.1322653714706));
#63386=CARTESIAN_POINT('Origin',(165.,-7.57107088371367,-29.1322653714706));
#63387=CARTESIAN_POINT('Origin',(165.,-7.57107088371367,-29.1322653714706));
#63388=CARTESIAN_POINT('',(165.,-7.57107088371367,-28.1322653714706));
#63389=CARTESIAN_POINT('Origin',(165.,-7.57107088371367,-29.1322653714706));
#63390=CARTESIAN_POINT('Ctrl Pts',(127.223161057301,-4.62069507309258,-17.698078925912));
#63391=CARTESIAN_POINT('Ctrl Pts',(130.307399870719,-5.92914147533279,-21.3918099998299));
#63392=CARTESIAN_POINT('Ctrl Pts',(137.492178871774,-7.56977128395659,-26.6032877773287));
#63393=CARTESIAN_POINT('Ctrl Pts',(146.27021147377,-7.81947858844033,-28.4368505439215));
#63394=CARTESIAN_POINT('Ctrl Pts',(150.052788176357,-7.63914239116798,-28.5431800803631));
#63395=CARTESIAN_POINT('Ctrl Pts',(127.284956078124,-4.47631553952072,-17.6939861612557));
#63396=CARTESIAN_POINT('Ctrl Pts',(130.379397801589,-5.75870424283007,-21.3658595958622));
#63397=CARTESIAN_POINT('Ctrl Pts',(137.573627386715,-7.35172410486705,-26.5132063461906));
#63398=CARTESIAN_POINT('Ctrl Pts',(146.296085686368,-7.57964096967766,-28.2546237099579));
#63399=CARTESIAN_POINT('Ctrl Pts',(150.041124530135,-7.39989439113669,-28.3250648769978));
#63400=CARTESIAN_POINT('Ctrl Pts',(127.321297410277,-4.32046304627996,-17.715214120084));
#63401=CARTESIAN_POINT('Ctrl Pts',(130.420987573119,-5.57091977783908,-21.3784706223684));
#63402=CARTESIAN_POINT('Ctrl Pts',(137.62079782197,-7.09907364076991,-26.4971349531396));
#63403=CARTESIAN_POINT('Ctrl Pts',(146.304992405087,-7.25777004098873,-28.1861302631782));
#63404=CARTESIAN_POINT('Ctrl Pts',(150.020722457357,-7.05080162839578,-28.2347435757426));
#63405=CARTESIAN_POINT('Ctrl Pts',(127.328278974584,-4.16988910307848,-17.7594811554948));
#63406=CARTESIAN_POINT('Ctrl Pts',(130.426320557835,-5.39188507649873,-21.4274847111505));
#63407=CARTESIAN_POINT('Ctrl Pts',(137.62133120349,-6.86523720579351,-26.5551071073711));
#63408=CARTESIAN_POINT('Ctrl Pts',(146.292010364479,-6.96723340941636,-28.2545429014871));
#63409=CARTESIAN_POINT('Ctrl Pts',(150.000022383365,-6.73628528178718,-28.3095824877733));
#63410=CARTESIAN_POINT('',(127.849160658777,-4.87571718501567,-18.4228377223213));
#63411=CARTESIAN_POINT('Ctrl Pts',(127.849390667069,-4.87581470103703,-18.4225978737085));
#63412=CARTESIAN_POINT('Ctrl Pts',(130.853617533308,-6.05135486562993,-21.7815128222371));
#63413=CARTESIAN_POINT('Ctrl Pts',(137.824456096834,-7.57922352160175,-26.6726941210597));
#63414=CARTESIAN_POINT('Ctrl Pts',(146.27021147377,-7.81947858844033,-28.4368505439215));
#63415=CARTESIAN_POINT('Ctrl Pts',(150.052788176357,-7.63914239116798,-28.5431800803631));
#63416=CARTESIAN_POINT('Ctrl Pts',(127.464959790631,-4.7216572617532,-17.983759079599));
#63417=CARTESIAN_POINT('Ctrl Pts',(127.591474106957,-4.77365180285252,-18.1312277407253));
#63418=CARTESIAN_POINT('Ctrl Pts',(127.719628690941,-4.82503943619632,-18.277515807416));
#63419=CARTESIAN_POINT('Ctrl Pts',(127.849390667069,-4.87581470103703,-18.4225978737085));
#63420=CARTESIAN_POINT('Origin',(158.5,0.,0.));
#63421=CARTESIAN_POINT('',(165.,7.31954028957033,-28.1644160235812));
#63422=CARTESIAN_POINT('Origin',(165.,0.,0.));
#63423=CARTESIAN_POINT('Ctrl Pts',(150.,6.73628528150279,-28.3095824873171));
#63424=CARTESIAN_POINT('Ctrl Pts',(152.860692060566,6.56397499464613,-28.3505838425905));
#63425=CARTESIAN_POINT('Ctrl Pts',(157.882579751756,6.54039874786384,-28.3550078873843));
#63426=CARTESIAN_POINT('Ctrl Pts',(162.894354921365,6.91344062208961,-28.2699556831011));
#63427=CARTESIAN_POINT('Ctrl Pts',(165.,7.31954028957033,-28.1644160235812));
#63428=CARTESIAN_POINT('Origin',(165.,-21.4437464396264,-21.122872404884));
#63429=CARTESIAN_POINT('',(164.848300728223,-20.4572239433816,-21.1841969134041));
#63430=CARTESIAN_POINT('',(165.,-20.7313296143896,-20.4211158465822));
#63431=CARTESIAN_POINT('Origin',(165.,-21.4437464396264,-21.122872404884));
#63432=CARTESIAN_POINT('Origin',(165.,-21.4437464396264,-21.122872404884));
#63433=CARTESIAN_POINT('Origin',(165.,-21.4437464396264,-21.122872404884));
#63434=CARTESIAN_POINT('Ctrl Pts',(164.848300728804,-20.4572239432962,-21.1841969134672));
#63435=CARTESIAN_POINT('Ctrl Pts',(162.799367188007,-20.758461879727,-20.9617128623935));
#63436=CARTESIAN_POINT('Ctrl Pts',(157.868853335481,-21.0564796490984,-20.8051063645433));
#63437=CARTESIAN_POINT('Ctrl Pts',(152.873956928668,-21.0354627790605,-20.8103848369588));
#63438=CARTESIAN_POINT('Ctrl Pts',(150.052788176347,-20.8995478587445,-20.8872814137861));
#63439=CARTESIAN_POINT('Ctrl Pts',(164.886050421238,-20.4340175278447,-20.9042590799883));
#63440=CARTESIAN_POINT('Ctrl Pts',(162.821008664813,-20.7135464797034,-20.6598174131805));
#63441=CARTESIAN_POINT('Ctrl Pts',(157.870850327895,-20.9589589584795,-20.4733053331211));
#63442=CARTESIAN_POINT('Ctrl Pts',(152.87160120197,-20.9449235011256,-20.4813909437905));
#63443=CARTESIAN_POINT('Ctrl Pts',(150.041115769415,-20.8302780650708,-20.5710289076513));
#63444=CARTESIAN_POINT('Ctrl Pts',(164.942784455296,-20.5365303500286,-20.6188742741048));
#63445=CARTESIAN_POINT('Ctrl Pts',(162.857491290603,-20.8152264917387,-20.3410661250567));
#63446=CARTESIAN_POINT('Ctrl Pts',(157.876604437521,-21.0494810521585,-20.0938994608672));
#63447=CARTESIAN_POINT('Ctrl Pts',(152.866153867665,-21.0371303229397,-20.1087996479862));
#63448=CARTESIAN_POINT('Ctrl Pts',(150.020705033617,-20.9266039447126,-20.2235449127931));
#63449=CARTESIAN_POINT('Ctrl Pts',(165.000000000597,-20.7313296143061,-20.421115846667));
#63450=CARTESIAN_POINT('Ctrl Pts',(162.894422761796,-21.025769987728,-20.122202678601));
#63451=CARTESIAN_POINT('Ctrl Pts',(157.882541867759,-21.2859684563718,-19.8416434222251));
#63452=CARTESIAN_POINT('Ctrl Pts',(152.86059133337,-21.2703340386193,-19.8598655489513));
#63453=CARTESIAN_POINT('Ctrl Pts',(150.,-21.1486749637962,-19.9885854245792));
#63454=CARTESIAN_POINT('',(150.052788176347,-20.8995478587445,-20.8872814137861));
#63455=CARTESIAN_POINT('Origin',(150.,-21.8754335536174,-20.675478394496));
#63456=CARTESIAN_POINT('Ctrl Pts',(150.,-21.1486749637962,-19.9885854245792));
#63457=CARTESIAN_POINT('Ctrl Pts',(152.86059133337,-21.2703340386193,-19.8598655489513));
#63458=CARTESIAN_POINT('Ctrl Pts',(157.882541867759,-21.2859684563718,-19.8416434222251));
#63459=CARTESIAN_POINT('Ctrl Pts',(162.894422761796,-21.025769987728,-20.122202678601));
#63460=CARTESIAN_POINT('Ctrl Pts',(165.000000000597,-20.7313296143061,-20.421115846667));
#63461=CARTESIAN_POINT('Ctrl Pts',(164.848300728804,-20.4572239432962,-21.1841969134672));
#63462=CARTESIAN_POINT('Ctrl Pts',(162.799367188007,-20.758461879727,-20.9617128623935));
#63463=CARTESIAN_POINT('Ctrl Pts',(157.868853335481,-21.0564796490984,-20.8051063645433));
#63464=CARTESIAN_POINT('Ctrl Pts',(152.873956928668,-21.0354627790605,-20.8103848369588));
#63465=CARTESIAN_POINT('Ctrl Pts',(150.052788176347,-20.8995478587445,-20.8872814137861));
#63466=CARTESIAN_POINT('Ctrl Pts',(150.052788176357,-20.8995478588044,-20.8872814140596));
#63467=CARTESIAN_POINT('Ctrl Pts',(146.270211473775,-20.7172956804374,-20.9902923738984));
#63468=CARTESIAN_POINT('Ctrl Pts',(137.492160038673,-19.2542660948047,-19.8572749795118));
#63469=CARTESIAN_POINT('Ctrl Pts',(130.307399870729,-15.561280155124,-15.830692140194));
#63470=CARTESIAN_POINT('Ctrl Pts',(127.223161057304,-13.0166384114775,-12.8506787793981));
#63471=CARTESIAN_POINT('Ctrl Pts',(150.041124530135,-20.8302785517541,-20.5710289665452));
#63472=CARTESIAN_POINT('Ctrl Pts',(146.296085686373,-20.679401422355,-20.6914734862849));
#63473=CARTESIAN_POINT('Ctrl Pts',(137.573606595474,-19.2852642849748,-19.6233996678116));
#63474=CARTESIAN_POINT('Ctrl Pts',(130.379397801599,-15.6240250623009,-15.670113965112));
#63475=CARTESIAN_POINT('Ctrl Pts',(127.284956078127,-13.0852837400994,-12.7235960532101));
#63476=CARTESIAN_POINT('Ctrl Pts',(150.020722457357,-20.9266043917347,-20.2235451151067));
#63477=CARTESIAN_POINT('Ctrl Pts',(146.304992405092,-20.7810198217955,-20.3784783619107));
#63478=CARTESIAN_POINT('Ctrl Pts',(137.620776912513,-19.3976728561088,-19.396560999606));
#63479=CARTESIAN_POINT('Ctrl Pts',(130.42098757313,-15.7288387641185,-15.5137933612467));
#63480=CARTESIAN_POINT('Ctrl Pts',(127.32129741028,-13.1815939383356,-12.5992378142346));
#63481=CARTESIAN_POINT('Ctrl Pts',(150.000022383365,-21.1486749640491,-19.9885854250535));
#63482=CARTESIAN_POINT('Ctrl Pts',(146.292010364484,-20.9855352202971,-20.1610725773935));
#63483=CARTESIAN_POINT('Ctrl Pts',(137.621314702796,-19.5648105010933,-19.2230426666669));
#63484=CARTESIAN_POINT('Ctrl Pts',(130.426320557845,-15.8608035608174,-15.383251806118));
#63485=CARTESIAN_POINT('Ctrl Pts',(127.328278974586,-13.2952172871523,-12.4909704719795));
#63486=CARTESIAN_POINT('',(127.849160658792,-13.516786884833,-13.433913805062));
#63487=CARTESIAN_POINT('Ctrl Pts',(150.052788176357,-20.8995478588044,-20.8872814140596));
#63488=CARTESIAN_POINT('Ctrl Pts',(146.270211473775,-20.7172956804374,-20.9902923738984));
#63489=CARTESIAN_POINT('Ctrl Pts',(137.824437948057,-19.3096465417837,-19.9001633874786));
#63490=CARTESIAN_POINT('Ctrl Pts',(130.853616114337,-15.8376680709596,-16.1313846545366));
#63491=CARTESIAN_POINT('Ctrl Pts',(127.849390477127,-13.516530575009,-13.4338784035537));
#63492=CARTESIAN_POINT('Ctrl Pts',(127.849390477127,-13.516530575009,-13.4338784035538));
#63493=CARTESIAN_POINT('Ctrl Pts',(127.719628570137,-13.4162733825632,-13.3173646667328));
#63494=CARTESIAN_POINT('Ctrl Pts',(127.591474039895,-13.3152779704518,-13.1997176167471));
#63495=CARTESIAN_POINT('Ctrl Pts',(127.464959760394,-13.2135636128087,-13.0809546870724));
#63496=CARTESIAN_POINT('Origin',(155.,-2.16262821021008E-15,-3.7457819379656E-15));
#63497=CARTESIAN_POINT('Ctrl Pts',(164.848300728132,-8.11744071666462,-28.3085740843029));
#63498=CARTESIAN_POINT('Ctrl Pts',(164.798270483275,-9.53646247647449,-29.2590518177106));
#63499=CARTESIAN_POINT('Ctrl Pts',(164.727958910501,-12.9591271555504,-30.29114537139));
#63500=CARTESIAN_POINT('Ctrl Pts',(164.710733726509,-17.1339693172545,-28.7318180524794));
#63501=CARTESIAN_POINT('Ctrl Pts',(164.745475165276,-19.9513569110563,-25.4855311280028));
#63502=CARTESIAN_POINT('Ctrl Pts',(164.798266641053,-20.5708596534599,-22.8884755501744));
#63503=CARTESIAN_POINT('Ctrl Pts',(164.848300728223,-20.4572239433816,-21.1841969134041));
#63504=CARTESIAN_POINT('Ctrl Pts',(164.848300728223,-8.11744071408905,-28.3085740825778));
#63505=CARTESIAN_POINT('Ctrl Pts',(164.798270483317,-9.53646247440374,-29.2590518170862));
#63506=CARTESIAN_POINT('Ctrl Pts',(164.727958910505,-12.95912715454,-30.2911453717673));
#63507=CARTESIAN_POINT('Ctrl Pts',(164.710733726509,-17.1339693172545,-28.7318180524794));
#63508=CARTESIAN_POINT('Ctrl Pts',(164.745475165276,-19.9513569110563,-25.4855311280028));
#63509=CARTESIAN_POINT('Ctrl Pts',(164.798266641053,-20.5708596534599,-22.8884755501744));
#63510=CARTESIAN_POINT('Ctrl Pts',(164.848300728223,-20.4572239433816,-21.1841969134041));
#63511=CARTESIAN_POINT('Ctrl Pts',(165.010504706333,-8.13120148533915,-28.2878287434741));
#63512=CARTESIAN_POINT('Ctrl Pts',(164.963972531947,-9.55105232178415,-29.2280958614887));
#63513=CARTESIAN_POINT('Ctrl Pts',(164.897254300082,-12.9604500480093,-30.2393200900593));
#63514=CARTESIAN_POINT('Ctrl Pts',(164.880672093334,-17.1037809754509,-28.687112584774));
#63515=CARTESIAN_POINT('Ctrl Pts',(164.913916111783,-19.9089143586708,-25.4667798289579));
#63516=CARTESIAN_POINT('Ctrl Pts',(164.96396895833,-20.5367553748823,-22.8856324139044));
#63517=CARTESIAN_POINT('Ctrl Pts',(165.010504706333,-20.4323775670826,-21.1857414213305));
#63518=CARTESIAN_POINT('Ctrl Pts',(165.346643666359,-8.11348434695071,-28.3145385867768));
#63519=CARTESIAN_POINT('Ctrl Pts',(165.311962910978,-9.54610539081284,-29.2469736164883));
#63520=CARTESIAN_POINT('Ctrl Pts',(165.260681297213,-12.9648019155867,-30.2346929762586));
#63521=CARTESIAN_POINT('Ctrl Pts',(165.247690226289,-17.0973292423592,-28.6790699558661));
#63522=CARTESIAN_POINT('Ctrl Pts',(165.273524009678,-19.9093316570144,-25.4698265063441));
#63523=CARTESIAN_POINT('Ctrl Pts',(165.311960247537,-20.5555764444854,-22.8907876721078));
#63524=CARTESIAN_POINT('Ctrl Pts',(165.346643666359,-20.4643675391081,-21.1837528510551));
#63525=CARTESIAN_POINT('Ctrl Pts',(165.84092593075,-7.9327106299154,-28.5870677926454));
#63526=CARTESIAN_POINT('Ctrl Pts',(165.831140815774,-9.4213375450583,-29.5517299089082));
#63527=CARTESIAN_POINT('Ctrl Pts',(165.816207582955,-12.9763247577425,-30.5712033734336));
#63528=CARTESIAN_POINT('Ctrl Pts',(165.8123218556,-17.2757086549243,-28.950182175098));
#63529=CARTESIAN_POINT('Ctrl Pts',(165.81996762758,-20.2049668175332,-25.6141311461017));
#63530=CARTESIAN_POINT('Ctrl Pts',(165.831140064289,-20.8818870513838,-22.9351186567562));
#63531=CARTESIAN_POINT('Ctrl Pts',(165.84092593075,-20.7907716131811,-21.1634628227003));
#63532=CARTESIAN_POINT('Ctrl Pts',(166.,-7.70713717218929,-28.9271357865293));
#63533=CARTESIAN_POINT('Ctrl Pts',(166.000188628472,-9.25627523009477,-29.9459525591832));
#63534=CARTESIAN_POINT('Ctrl Pts',(166.000322627528,-12.9864301063653,-31.0398000946721));
#63535=CARTESIAN_POINT('Ctrl Pts',(166.000449863218,-17.5294747323444,-29.3334367489045));
#63536=CARTESIAN_POINT('Ctrl Pts',(166.000254419659,-20.6107325371867,-25.8084991572215));
#63537=CARTESIAN_POINT('Ctrl Pts',(166.000188642958,-21.3058263169705,-22.9892879280155));
#63538=CARTESIAN_POINT('Ctrl Pts',(166.,-21.1980658637617,-21.1381444748319));
#63539=CARTESIAN_POINT('Ctrl Pts',(166.,-7.57107088371367,-29.1322653714706));
#63540=CARTESIAN_POINT('Ctrl Pts',(166.,-9.15667614620178,-30.1840269840918));
#63541=CARTESIAN_POINT('Ctrl Pts',(166.,-12.9924218634215,-31.3233822840624));
#63542=CARTESIAN_POINT('Ctrl Pts',(166.,-17.6831143810041,-29.5655630495408));
#63543=CARTESIAN_POINT('Ctrl Pts',(166.,-20.8562314642464,-25.9259586209163));
#63544=CARTESIAN_POINT('Ctrl Pts',(166.,-21.5618051497126,-23.0220734941118));
#63545=CARTESIAN_POINT('Ctrl Pts',(166.,-21.4437464396264,-21.122872404884));
#63546=CARTESIAN_POINT('Origin',(165.,0.,0.));
#63547=CARTESIAN_POINT('',(165.000000000362,-28.0508699039984,-7.74330017685971));
#63548=CARTESIAN_POINT('Origin',(165.,0.,0.));
#63549=CARTESIAN_POINT('Origin',(165.,-29.0148173233401,-8.00939296658655));
#63550=CARTESIAN_POINT('Ctrl Pts',(127.110025063046,-18.8932088282594,5.4495616554018));
#63551=CARTESIAN_POINT('Ctrl Pts',(126.561429499416,-19.2648380810405,1.85688406416326));
#63552=CARTESIAN_POINT('Ctrl Pts',(126.561429543121,-19.2648380514345,-1.85688435037533));
#63553=CARTESIAN_POINT('Ctrl Pts',(127.110025063046,-18.8932088282595,-5.44956165540083));
#63554=CARTESIAN_POINT('Ctrl Pts',(127.362931194533,-18.7218853198324,5.39322150128864));
#63555=CARTESIAN_POINT('Ctrl Pts',(126.820035975585,-19.0896530593933,1.83787357333263));
#63556=CARTESIAN_POINT('Ctrl Pts',(126.820036018835,-19.0896530300949,-1.83787385657082));
#63557=CARTESIAN_POINT('Ctrl Pts',(127.362931194533,-18.7218853198325,-5.39322150128768));
#63558=CARTESIAN_POINT('Ctrl Pts',(127.647218583474,-18.2006252760714,5.29589178770983));
#63559=CARTESIAN_POINT('Ctrl Pts',(127.114085169261,-18.5617797346977,1.80447224301269));
#63560=CARTESIAN_POINT('Ctrl Pts',(127.114085211734,-18.5617797059261,-1.80447252115799));
#63561=CARTESIAN_POINT('Ctrl Pts',(127.647218583474,-18.2006252760715,-5.29589178770889));
#63562=CARTESIAN_POINT('Ctrl Pts',(127.47007422846,-17.6499357469874,5.26597768375927));
#63563=CARTESIAN_POINT('Ctrl Pts',(126.939976558162,-18.0090331072237,1.79444248385371));
#63564=CARTESIAN_POINT('Ctrl Pts',(126.939976600392,-18.009033078616,-1.79444276041493));
#63565=CARTESIAN_POINT('Ctrl Pts',(127.47007422846,-17.6499357469875,-5.26597768375833));
#63566=CARTESIAN_POINT('Ctrl Pts',(127.328278974586,-17.4651063902315,5.26851068351907));
#63567=CARTESIAN_POINT('Ctrl Pts',(126.797908769232,-17.8243882174359,1.7951925082875));
#63568=CARTESIAN_POINT('Ctrl Pts',(126.797908811484,-17.8243881888135,-1.79519278499075));
#63569=CARTESIAN_POINT('Ctrl Pts',(127.328278974586,-17.4651063902316,-5.26851068351812));
#63570=CARTESIAN_POINT('',(127.464921070561,-17.9352463278168,4.90283862543943));
#63571=CARTESIAN_POINT('Ctrl Pts',(127.464921070561,-17.9352463278168,4.90283862543943));
#63572=CARTESIAN_POINT('Ctrl Pts',(127.45225052721,-17.7646936285507,5.01023372772395));
#63573=CARTESIAN_POINT('Ctrl Pts',(127.404564208319,-17.6055373983341,5.13497641413088));
#63574=CARTESIAN_POINT('Ctrl Pts',(127.329689952111,-17.4676849997957,5.26605170523372));
#63575=CARTESIAN_POINT('Ctrl Pts',(127.328985684036,-17.4663947479229,5.26728090519223));
#63576=CARTESIAN_POINT('Ctrl Pts',(127.328278974586,-17.4651063902315,5.26851068351907));
#63577=CARTESIAN_POINT('',(126.797085404885,-19.1052002095942,2.686671805445));
#63578=CARTESIAN_POINT('Ctrl Pts',(126.797085404885,-19.1052002095942,2.686671805445));
#63579=CARTESIAN_POINT('Ctrl Pts',(126.969476250118,-18.9884193144365,3.27478905818323));
#63580=CARTESIAN_POINT('Ctrl Pts',(127.153613966227,-18.8183199497808,3.75991394003008));
#63581=CARTESIAN_POINT('Ctrl Pts',(127.375160462415,-18.45472723487,4.40330386019511));
#63582=CARTESIAN_POINT('Ctrl Pts',(127.435582156023,-18.296521770801,4.60168517640041));
#63583=CARTESIAN_POINT('Ctrl Pts',(127.467448207429,-18.0691174618076,4.80945858879493));
#63584=CARTESIAN_POINT('Ctrl Pts',(127.46981770909,-18.0011578594189,4.86133488079864));
#63585=CARTESIAN_POINT('Ctrl Pts',(127.464921070561,-17.9352463278168,4.90283862543943));
#63586=CARTESIAN_POINT('',(126.797085404885,-19.1052002095942,-2.68667180544497));
#63587=CARTESIAN_POINT('Ctrl Pts',(126.797739723099,-19.1047569617717,2.68660115054945));
#63588=CARTESIAN_POINT('Ctrl Pts',(126.665524631948,-19.1943220235194,0.900309345114276));
#63589=CARTESIAN_POINT('Ctrl Pts',(126.665524637169,-19.194322019982,-0.900309413205682));
#63590=CARTESIAN_POINT('Ctrl Pts',(126.797739723252,-19.104756961668,-2.6866011505329));
#63591=CARTESIAN_POINT('',(127.464921070561,-17.9352463278168,-4.90283862543942));
#63592=CARTESIAN_POINT('Ctrl Pts',(126.797085404885,-19.1052002095942,-2.68667180544496));
#63593=CARTESIAN_POINT('Ctrl Pts',(126.913668909287,-19.0262242872571,-3.08440041006524));
#63594=CARTESIAN_POINT('Ctrl Pts',(127.036713649274,-18.9228672390262,-3.43736008037827));
#63595=CARTESIAN_POINT('Ctrl Pts',(127.242196284535,-18.6805750672327,-4.01847563389922));
#63596=CARTESIAN_POINT('Ctrl Pts',(127.322999453907,-18.5537833666996,-4.24389900151411));
#63597=CARTESIAN_POINT('Ctrl Pts',(127.427486245728,-18.3037870887744,-4.58633594588917));
#63598=CARTESIAN_POINT('Ctrl Pts',(127.456769006322,-18.1859058432983,-4.71065867863441));
#63599=CARTESIAN_POINT('Ctrl Pts',(127.468025474849,-18.0271746269583,-4.84035139772881));
#63600=CARTESIAN_POINT('Ctrl Pts',(127.468398492741,-17.9820544024906,-4.87336411117509));
#63601=CARTESIAN_POINT('Ctrl Pts',(127.464921070561,-17.9352463278168,-4.9028386254394));
#63602=CARTESIAN_POINT('Ctrl Pts',(127.464921070561,-17.9352463278168,-4.9028386254394));
#63603=CARTESIAN_POINT('Ctrl Pts',(127.452250527209,-17.7646936285422,-5.01023372772925));
#63604=CARTESIAN_POINT('Ctrl Pts',(127.404564208274,-17.6055373982726,-5.13497641414103));
#63605=CARTESIAN_POINT('Ctrl Pts',(127.329689952113,-17.4676849997994,-5.26605170523214));
#63606=CARTESIAN_POINT('Ctrl Pts',(127.328985684035,-17.4663947479204,-5.26728090519385));
#63607=CARTESIAN_POINT('Ctrl Pts',(127.328278974586,-17.4651063902316,-5.26851068351812));
#63608=CARTESIAN_POINT('Ctrl Pts',(127.223161057304,-17.6373334845709,-4.84740014651676));
#63609=CARTESIAN_POINT('Ctrl Pts',(129.536338172585,-20.5271471019329,-5.38268796975447));
#63610=CARTESIAN_POINT('Ctrl Pts',(136.26241135915,-26.2301344772096,-6.59347728317351));
#63611=CARTESIAN_POINT('Ctrl Pts',(145.009334196347,-28.5361317066637,-7.37677649702869));
#63612=CARTESIAN_POINT('Ctrl Pts',(150.052765342883,-28.5386902383978,-7.65589740262126));
#63613=CARTESIAN_POINT('Ctrl Pts',(127.284956078127,-17.5615992796209,-4.97039010804839));
#63614=CARTESIAN_POINT('Ctrl Pts',(129.605785369344,-20.4274443273705,-5.5144062809461));
#63615=CARTESIAN_POINT('Ctrl Pts',(136.344308957598,-26.0580483580822,-6.73748831160726));
#63616=CARTESIAN_POINT('Ctrl Pts',(145.047721141658,-28.2686618330951,-7.49952020698795));
#63617=CARTESIAN_POINT('Ctrl Pts',(150.04110192192,-28.2301731145178,-7.75403475399862));
#63618=CARTESIAN_POINT('Ctrl Pts',(127.321297410279,-17.5020569846164,-5.11597630585222));
#63619=CARTESIAN_POINT('Ctrl Pts',(129.646063027636,-20.350330696392,-5.67750153807653));
#63620=CARTESIAN_POINT('Ctrl Pts',(136.391076364772,-25.928670384798,-6.94240078228871));
#63621=CARTESIAN_POINT('Ctrl Pts',(145.066397533214,-28.0592476052024,-7.7398015222993));
#63622=CARTESIAN_POINT('Ctrl Pts',(150.020700025828,-27.9774063873195,-8.01119722834054));
#63623=CARTESIAN_POINT('Ctrl Pts',(127.328278974586,-17.4651063902316,-5.26851068351812));
#63624=CARTESIAN_POINT('Ctrl Pts',(129.651808158315,-20.3057906258596,-5.85030184794966));
#63625=CARTESIAN_POINT('Ctrl Pts',(136.392549868564,-25.8653195043127,-7.16627842991105));
#63626=CARTESIAN_POINT('Ctrl Pts',(145.055988199056,-27.9753679280975,-8.01762643934787));
#63627=CARTESIAN_POINT('Ctrl Pts',(150.,-27.884960655152,-8.32099568925641));
#63628=CARTESIAN_POINT('',(127.849160658777,-18.3925040698363,-4.98892391726873));
#63629=CARTESIAN_POINT('',(150.052765342883,-28.5386902383978,-7.65589740262126));
#63630=CARTESIAN_POINT('Ctrl Pts',(127.849242092298,-18.3924580623247,-4.98880236863075));
#63631=CARTESIAN_POINT('Ctrl Pts',(130.04841076249,-20.9540078969733,-5.47373470087007));
#63632=CARTESIAN_POINT('Ctrl Pts',(136.59349121896,-26.317418800355,-6.62312594919461));
#63633=CARTESIAN_POINT('Ctrl Pts',(145.009334196347,-28.5361317066637,-7.37677649702869));
#63634=CARTESIAN_POINT('Ctrl Pts',(150.052765342883,-28.5386902383978,-7.65589740262126));
#63635=CARTESIAN_POINT('Origin',(149.99997684747,-28.843206725519,-8.60694055822638));
#63636=CARTESIAN_POINT('Ctrl Pts',(127.849242092298,-18.3924580623247,-4.98880236863075));
#63637=CARTESIAN_POINT('Ctrl Pts',(127.71953388091,-18.2413764049986,-4.96020078553652));
#63638=CARTESIAN_POINT('Ctrl Pts',(127.591421464258,-18.0889606118247,-4.93153597887233));
#63639=CARTESIAN_POINT('Ctrl Pts',(127.464935664776,-17.9352383975751,-4.90281760981483));
#63640=CARTESIAN_POINT('Ctrl Pts',(150.052765342888,-28.5386902386737,-7.65589740253316));
#63641=CARTESIAN_POINT('Ctrl Pts',(152.168609613435,-28.5397124602787,-7.77301191157992));
#63642=CARTESIAN_POINT('Ctrl Pts',(155.727161730325,-28.5490204299122,-7.81897514648418));
#63643=CARTESIAN_POINT('Ctrl Pts',(160.688042943987,-28.5326149000753,-7.66254093649981));
#63644=CARTESIAN_POINT('Ctrl Pts',(163.482365784657,-28.5466265021039,-7.37245455461431));
#63645=CARTESIAN_POINT('Ctrl Pts',(164.848300728928,-28.5746646574851,-7.12437716904556));
#63646=CARTESIAN_POINT('Ctrl Pts',(150.041092860165,-28.2301728106309,-7.75403434833187));
#63647=CARTESIAN_POINT('Ctrl Pts',(152.163924563052,-28.2149433767642,-7.8621120542075));
#63648=CARTESIAN_POINT('Ctrl Pts',(155.727838713922,-28.2140248889323,-7.90031724868427));
#63649=CARTESIAN_POINT('Ctrl Pts',(160.700266431706,-28.2254189367548,-7.76236208985673));
#63650=CARTESIAN_POINT('Ctrl Pts',(163.509376829801,-28.2726767580587,-7.48711172241153));
#63651=CARTESIAN_POINT('Ctrl Pts',(164.886050421363,-28.3206281744881,-7.24424874047374));
#63652=CARTESIAN_POINT('Ctrl Pts',(150.020682003358,-27.9774059754965,-8.01119693236669));
#63653=CARTESIAN_POINT('Ctrl Pts',(152.154736119442,-27.9443244242393,-8.12601440166864));
#63654=CARTESIAN_POINT('Ctrl Pts',(155.729373272436,-27.9313763655993,-8.1678953539404));
#63655=CARTESIAN_POINT('Ctrl Pts',(160.722407435408,-27.9750435222419,-8.01929016029531));
#63656=CARTESIAN_POINT('Ctrl Pts',(163.552610130101,-28.0572412233664,-7.72922400951313));
#63657=CARTESIAN_POINT('Ctrl Pts',(164.942784455423,-28.1247340938326,-7.47571985163942));
#63658=CARTESIAN_POINT('Ctrl Pts',(149.999976847469,-27.8849606552027,-8.32099568908656));
#63659=CARTESIAN_POINT('Ctrl Pts',(152.145387697858,-27.8469771399051,-8.44828440178341));
#63660=CARTESIAN_POINT('Ctrl Pts',(155.730932513824,-27.8315707318698,-8.49824064588987));
#63661=CARTESIAN_POINT('Ctrl Pts',(160.744916186185,-27.8833260496286,-8.32821637329774));
#63662=CARTESIAN_POINT('Ctrl Pts',(163.596303164748,-27.9764402277335,-8.01292903254352));
#63663=CARTESIAN_POINT('Ctrl Pts',(165.000000000725,-28.0508699039984,-7.74330017685971));
#63664=CARTESIAN_POINT('',(164.848300728422,-28.5746646621997,-7.12437716678769));
#63665=CARTESIAN_POINT('Ctrl Pts',(150.052765342888,-28.5386902386737,-7.65589740253316));
#63666=CARTESIAN_POINT('Ctrl Pts',(152.168609613435,-28.5397124602787,-7.77301191157992));
#63667=CARTESIAN_POINT('Ctrl Pts',(155.727161730325,-28.5490204299122,-7.81897514648418));
#63668=CARTESIAN_POINT('Ctrl Pts',(160.688042943987,-28.5326149000753,-7.66254093649981));
#63669=CARTESIAN_POINT('Ctrl Pts',(163.482365784657,-28.5466265021039,-7.37245455461431));
#63670=CARTESIAN_POINT('Ctrl Pts',(164.848300728928,-28.5746646574851,-7.12437716904556));
#63671=CARTESIAN_POINT('Origin',(165.000000000725,-29.0148173233798,-8.00939296644252));
#63672=CARTESIAN_POINT('Ctrl Pts',(165.000000000725,-28.0508699039984,-7.74330017685971));
#63673=CARTESIAN_POINT('Ctrl Pts',(163.596303164748,-27.9764402277335,-8.01292903254352));
#63674=CARTESIAN_POINT('Ctrl Pts',(160.744916186185,-27.8833260496286,-8.32821637329774));
#63675=CARTESIAN_POINT('Ctrl Pts',(155.73094021419,-27.8315708113545,-8.49824038477032));
#63676=CARTESIAN_POINT('Ctrl Pts',(152.14540311634,-27.846977073655,-8.44828461660339));
#63677=CARTESIAN_POINT('Ctrl Pts',(149.999999911594,-27.8849602468641,-8.32099705749327));
#63678=CARTESIAN_POINT('Origin',(165.,-29.0148173233401,-8.00939296658655));
#63679=CARTESIAN_POINT('Origin',(165.,-29.0148173233401,-8.00939296658655));
#63680=CARTESIAN_POINT('Origin',(155.,-4.32525642042015E-15,5.29691143075908E-31));
#63681=CARTESIAN_POINT('Origin',(133.079689783217,-14.8492424049175,3.30061879420892E-15));
#63682=CARTESIAN_POINT('',(127.849160658792,-18.3925040698507,4.98892391727468));
#63683=CARTESIAN_POINT('Ctrl Pts',(127.849390961451,-18.3923448905527,4.98871937797864));
#63684=CARTESIAN_POINT('Ctrl Pts',(127.719628878169,-18.2413126033933,4.96015108108561));
#63685=CARTESIAN_POINT('Ctrl Pts',(127.591474210887,-18.0889296687244,4.93151009034686));
#63686=CARTESIAN_POINT('Ctrl Pts',(127.464959837483,-17.9352208155387,4.9028043775574));
#63687=CARTESIAN_POINT('',(150.052788176347,-28.5386902497055,7.65589866638835));
#63688=CARTESIAN_POINT('Ctrl Pts',(150.052788176357,-28.5386902499724,7.65589866630348));
#63689=CARTESIAN_POINT('Ctrl Pts',(146.270211473775,-28.5367742688775,7.44655817002323));
#63690=CARTESIAN_POINT('Ctrl Pts',(137.824484222578,-26.8887993049828,6.7725224664745));
#63691=CARTESIAN_POINT('Ctrl Pts',(130.853619732367,-21.8890176546244,5.65012752812033));
#63692=CARTESIAN_POINT('Ctrl Pts',(127.849390961451,-18.3923448905527,4.98871937797864));
#63693=CARTESIAN_POINT('',(164.848300728421,-28.5746646621985,7.12437716678831));
#63694=CARTESIAN_POINT('Ctrl Pts',(164.848300728928,-28.5746646574851,7.1243771690456));
#63695=CARTESIAN_POINT('Ctrl Pts',(163.482355675751,-28.5466262946013,7.37245639056625));
#63696=CARTESIAN_POINT('Ctrl Pts',(160.688253082504,-28.5326161304868,7.66251821259513));
#63697=CARTESIAN_POINT('Ctrl Pts',(155.727427789529,-28.5490205309232,7.81896441116671));
#63698=CARTESIAN_POINT('Ctrl Pts',(152.16864825808,-28.539712545113,7.77301330068813));
#63699=CARTESIAN_POINT('Ctrl Pts',(150.052788176347,-28.5386902497055,7.65589866638835));
#63700=CARTESIAN_POINT('Ctrl Pts',(164.848300728068,-28.5746646622143,-7.12437716684098));
#63701=CARTESIAN_POINT('Ctrl Pts',(164.823285605682,-29.3409890323895,-6.74754215431457));
#63702=CARTESIAN_POINT('Ctrl Pts',(164.75934847695,-31.4726749978279,-5.28746335751779));
#63703=CARTESIAN_POINT('Ctrl Pts',(164.707290739753,-33.6036646709717,-1.36230726043271));
#63704=CARTESIAN_POINT('Ctrl Pts',(164.727957523923,-32.7110845673847,3.92638356344943));
#63705=CARTESIAN_POINT('Ctrl Pts',(164.79826664098,-30.1074311097653,6.37064925997245));
#63706=CARTESIAN_POINT('Ctrl Pts',(164.848300728068,-28.5746646622131,7.12437716684159));
#63707=CARTESIAN_POINT('Origin',(133.079689783217,-14.8492424049175,2.86216733792408E-15));
#63708=CARTESIAN_POINT('Ctrl Pts',(164.848300728928,-28.5746646574851,7.1243771690456));
#63709=CARTESIAN_POINT('Ctrl Pts',(163.482355675751,-28.5466262946013,7.37245639056625));
#63710=CARTESIAN_POINT('Ctrl Pts',(160.688253082504,-28.5326161304868,7.66251821259513));
#63711=CARTESIAN_POINT('Ctrl Pts',(155.727427789529,-28.5490205309232,7.81896441116671));
#63712=CARTESIAN_POINT('Ctrl Pts',(152.16864825808,-28.539712545113,7.77301330068813));
#63713=CARTESIAN_POINT('Ctrl Pts',(150.052788176347,-28.5386902497055,7.65589866638835));
#63714=CARTESIAN_POINT('Ctrl Pts',(164.886050421363,-28.3206281744881,7.24424874047378));
#63715=CARTESIAN_POINT('Ctrl Pts',(163.509366641421,-28.2726764031836,7.48711351977311));
#63716=CARTESIAN_POINT('Ctrl Pts',(160.700477667292,-28.2254226634644,7.76234047582256));
#63717=CARTESIAN_POINT('Ctrl Pts',(155.728105525916,-28.2140263886644,7.90030725550932));
#63718=CARTESIAN_POINT('Ctrl Pts',(152.163963306891,-28.2149432403176,7.86211330798194));
#63719=CARTESIAN_POINT('Ctrl Pts',(150.041115769415,-28.2301726485455,7.75403551841943));
#63720=CARTESIAN_POINT('Ctrl Pts',(164.942784455423,-28.1247340938326,7.47571985163946));
#63721=CARTESIAN_POINT('Ctrl Pts',(163.552599841806,-28.0572407238704,7.72922588562709));
#63722=CARTESIAN_POINT('Ctrl Pts',(160.722620218241,-27.9750498693307,8.01926740597123));
#63723=CARTESIAN_POINT('Ctrl Pts',(155.729641322233,-27.9313793869812,8.16788476575447));
#63724=CARTESIAN_POINT('Ctrl Pts',(152.15477503479,-27.9443240352357,8.12601574303588));
#63725=CARTESIAN_POINT('Ctrl Pts',(150.020705033617,-27.9774056214107,8.01119817466016));
#63726=CARTESIAN_POINT('Ctrl Pts',(165.000000000725,-28.0508699039984,7.74330017685976));
#63727=CARTESIAN_POINT('Ctrl Pts',(163.596292776377,-27.9764396769001,8.01293102799189));
#63728=CARTESIAN_POINT('Ctrl Pts',(160.745130525767,-27.8833331905189,8.32819167527699));
#63729=CARTESIAN_POINT('Ctrl Pts',(155.731201818055,-27.8315741795666,8.49822897795261));
#63730=CARTESIAN_POINT('Ctrl Pts',(152.145426787195,-27.8469766825496,8.44828591156898));
#63731=CARTESIAN_POINT('Ctrl Pts',(150.,-27.884960245299,8.32099706273789));
#63732=CARTESIAN_POINT('Origin',(150.,-28.8432063018385,8.60694197898318));
#63733=CARTESIAN_POINT('',(165.000000000362,-28.0508699039984,7.74330017685976));
#63734=CARTESIAN_POINT('Ctrl Pts',(150.,-27.884960245299,8.32099706273789));
#63735=CARTESIAN_POINT('Ctrl Pts',(152.145426787195,-27.8469766825496,8.44828591156898));
#63736=CARTESIAN_POINT('Ctrl Pts',(155.731201818055,-27.8315741795666,8.49822897795261));
#63737=CARTESIAN_POINT('Ctrl Pts',(160.745130525767,-27.8833331905189,8.32819167527699));
#63738=CARTESIAN_POINT('Ctrl Pts',(163.596292776377,-27.9764396769001,8.01293102799189));
#63739=CARTESIAN_POINT('Ctrl Pts',(165.000000000725,-28.0508699039984,7.74330017685976));
#63740=CARTESIAN_POINT('Origin',(165.000000000725,-29.0148173233798,8.00939296644257));
#63741=CARTESIAN_POINT('Ctrl Pts',(150.052788176357,-28.5386902499724,7.65589866630348));
#63742=CARTESIAN_POINT('Ctrl Pts',(146.270211473775,-28.5367742688775,7.44655817002323));
#63743=CARTESIAN_POINT('Ctrl Pts',(137.492208058031,-26.8239638226157,6.74600420562121));
#63744=CARTESIAN_POINT('Ctrl Pts',(130.307399870729,-21.4904216304607,5.56111785964704));
#63745=CARTESIAN_POINT('Ctrl Pts',(127.223161057304,-17.6373334845711,4.84740014651678));
#63746=CARTESIAN_POINT('Ctrl Pts',(150.041124530135,-28.2301729428908,7.75403591045255));
#63747=CARTESIAN_POINT('Ctrl Pts',(146.296085686373,-28.2590423920324,7.56315022367304));
#63748=CARTESIAN_POINT('Ctrl Pts',(137.573659607326,-26.6369374495338,6.88981462960117));
#63749=CARTESIAN_POINT('Ctrl Pts',(130.379397801599,-21.3827293051347,5.6957456307613));
#63750=CARTESIAN_POINT('Ctrl Pts',(127.284956078127,-17.5615992796211,4.97039010804842));
#63751=CARTESIAN_POINT('Ctrl Pts',(150.020722457357,-27.9774060201304,8.01119846063587));
#63752=CARTESIAN_POINT('Ctrl Pts',(146.304992405092,-28.0387898627839,7.80765190126751));
#63753=CARTESIAN_POINT('Ctrl Pts',(137.620830225758,-26.4966944429774,7.10057757161996));
#63754=CARTESIAN_POINT('Ctrl Pts',(130.42098757313,-21.2997585419613,5.86467726113271));
#63755=CARTESIAN_POINT('Ctrl Pts',(127.32129741028,-17.5020569846165,5.11597630585226));
#63756=CARTESIAN_POINT('Ctrl Pts',(150.000022383365,-27.8849602458363,8.32099706271974));
#63757=CARTESIAN_POINT('Ctrl Pts',(146.292010364484,-27.9527686297132,8.09347032409363));
#63758=CARTESIAN_POINT('Ctrl Pts',(137.621356775365,-26.4299654718048,7.33205606928553));
#63759=CARTESIAN_POINT('Ctrl Pts',(130.426320557845,-21.2526886373198,6.04423290504359));
#63760=CARTESIAN_POINT('Ctrl Pts',(127.328278974586,-17.4651063902317,5.26851068351816));
#63761=CARTESIAN_POINT('Origin',(165.,-29.0148173233401,8.00939296658655));
#63762=CARTESIAN_POINT('Origin',(165.,-29.0148173233401,8.00939296658655));
#63763=CARTESIAN_POINT('Origin',(165.,-29.0148173233401,8.00939296658655));
#63764=CARTESIAN_POINT('Ctrl Pts',(164.848300728225,-20.4572239433766,21.1841969133291));
#63765=CARTESIAN_POINT('Ctrl Pts',(164.823285605772,-20.5140374352135,22.0362707934392));
#63766=CARTESIAN_POINT('Ctrl Pts',(164.75934857031,-20.3154311261898,24.6124011045219));
#63767=CARTESIAN_POINT('Ctrl Pts',(164.707290846802,-17.981646634823,28.4204658567131));
#63768=CARTESIAN_POINT('Ctrl Pts',(164.727957731471,-12.9552328630782,30.2918070911301));
#63769=CARTESIAN_POINT('Ctrl Pts',(164.798266641053,-9.53657145358806,29.2591248126568));
#63770=CARTESIAN_POINT('Ctrl Pts',(164.848300728224,-8.11744071405221,28.3085740825531));
#63771=CARTESIAN_POINT('Ctrl Pts',(165.010504706335,-20.432377567078,21.1857414212557));
#63772=CARTESIAN_POINT('Ctrl Pts',(164.987238619141,-20.4845624632464,22.0356216477377));
#63773=CARTESIAN_POINT('Ctrl Pts',(164.927238219583,-20.2738925189293,24.6009637976647));
#63774=CARTESIAN_POINT('Ctrl Pts',(164.877329245491,-17.9446387756026,28.3773780702397));
#63775=CARTESIAN_POINT('Ctrl Pts',(164.897259516307,-12.9567274422132,30.2398779726856));
#63776=CARTESIAN_POINT('Ctrl Pts',(164.96396895833,-9.55116136464066,29.2281680728961));
#63777=CARTESIAN_POINT('Ctrl Pts',(165.010504706334,-8.1312014853023,28.2878287434497));
#63778=CARTESIAN_POINT('Ctrl Pts',(165.34664366636,-20.4643675391043,21.18375285098));
#63779=CARTESIAN_POINT('Ctrl Pts',(165.32930328867,-20.5099684897007,22.0372047174037));
#63780=CARTESIAN_POINT('Ctrl Pts',(165.28395294769,-20.2790321640665,24.6075978058925));
#63781=CARTESIAN_POINT('Ctrl Pts',(165.245038300776,-17.9353899642793,28.3689599675179));
#63782=CARTESIAN_POINT('Ctrl Pts',(165.260697889921,-12.9613040247773,30.2350974286757));
#63783=CARTESIAN_POINT('Ctrl Pts',(165.311960247537,-9.54621541440615,29.2470452264008));
#63784=CARTESIAN_POINT('Ctrl Pts',(165.34664366636,-8.11348434691343,28.3145385867528));
#63785=CARTESIAN_POINT('Ctrl Pts',(165.840925930751,-20.7907716131773,21.1634628226223));
#63786=CARTESIAN_POINT('Ctrl Pts',(165.836033373262,-20.8363258337755,22.0492227143292));
#63787=CARTESIAN_POINT('Ctrl Pts',(165.823057804221,-20.5908898164831,24.7182659833224));
#63788=CARTESIAN_POINT('Ctrl Pts',(165.811521565886,-18.1475857625226,28.6271012887971));
#63789=CARTESIAN_POINT('Ctrl Pts',(165.816211733742,-12.9727034529209,30.5715985406078));
#63790=CARTESIAN_POINT('Ctrl Pts',(165.831140064289,-9.42145186983594,29.551803993823));
#63791=CARTESIAN_POINT('Ctrl Pts',(165.84092593075,-7.93271062987668,28.5870677926205));
#63792=CARTESIAN_POINT('Ctrl Pts',(166.,-21.1980658637569,21.1381444747505));
#63793=CARTESIAN_POINT('Ctrl Pts',(166.000094314236,-21.2519419527489,22.0636451239774));
#63794=CARTESIAN_POINT('Ctrl Pts',(166.000254963943,-21.012709323309,24.8616125503422));
#63795=CARTESIAN_POINT('Ctrl Pts',(166.000465818828,-18.4514877712921,28.9930318844327));
#63796=CARTESIAN_POINT('Ctrl Pts',(166.000340749714,-12.9823367813052,31.040380240574));
#63797=CARTESIAN_POINT('Ctrl Pts',(166.000188642958,-9.25639420205611,29.9460308031115));
#63798=CARTESIAN_POINT('Ctrl Pts',(166.,-7.70713717214908,28.9271357865028));
#63799=CARTESIAN_POINT('Ctrl Pts',(166.,-21.4437464396212,21.1228724048004));
#63800=CARTESIAN_POINT('Ctrl Pts',(166.,-21.5027712616354,22.072400026806));
#63801=CARTESIAN_POINT('Ctrl Pts',(166.,-21.2677585367956,24.9482212131187));
#63802=CARTESIAN_POINT('Ctrl Pts',(166.,-18.6355842566111,29.2146519968481));
#63803=CARTESIAN_POINT('Ctrl Pts',(166.,-12.9880322537693,31.3241061902636));
#63804=CARTESIAN_POINT('Ctrl Pts',(166.,-9.15679791880095,30.184107758145));
#63805=CARTESIAN_POINT('Ctrl Pts',(166.,-7.57107088367251,29.1322653714433));
#63806=CARTESIAN_POINT('Origin',(165.,0.,0.));
#63807=CARTESIAN_POINT('Origin',(165.,0.,0.));
#63808=CARTESIAN_POINT('Ctrl Pts',(164.848300728223,-28.5746646574706,-7.12437716917368));
#63809=CARTESIAN_POINT('Ctrl Pts',(164.82328560577,-29.3409890294572,-6.74754215632307));
#63810=CARTESIAN_POINT('Ctrl Pts',(164.759348476971,-31.4726749969484,-5.28746335913763));
#63811=CARTESIAN_POINT('Ctrl Pts',(164.707290739753,-33.6036646709717,-1.36230726043271));
#63812=CARTESIAN_POINT('Ctrl Pts',(164.72795752393,-32.7110845670778,3.9263835652676));
#63813=CARTESIAN_POINT('Ctrl Pts',(164.798266641053,-30.10743110708,6.37064926249336));
#63814=CARTESIAN_POINT('Ctrl Pts',(164.848300728223,-28.5746646574706,7.12437716917368));
#63815=CARTESIAN_POINT('Ctrl Pts',(165.010504706333,-28.5635790524218,-7.10208732214358));
#63816=CARTESIAN_POINT('Ctrl Pts',(164.98723861914,-29.3256893668049,-6.72234065467426));
#63817=CARTESIAN_POINT('Ctrl Pts',(164.92723828344,-31.4420024657291,-5.25720937154396));
#63818=CARTESIAN_POINT('Ctrl Pts',(164.877329365366,-33.5478480428371,-1.35180246430346));
#63819=CARTESIAN_POINT('Ctrl Pts',(164.897259539862,-32.6668631380086,3.89912337054254));
#63820=CARTESIAN_POINT('Ctrl Pts',(164.96396895833,-30.0879167395549,6.34253565900248));
#63821=CARTESIAN_POINT('Ctrl Pts',(165.010504706333,-28.5635790524218,7.10208732214357));
#63822=CARTESIAN_POINT('Ctrl Pts',(165.346644572269,-28.5778515481473,-7.13078505628244));
#63823=CARTESIAN_POINT('Ctrl Pts',(165.329304194579,-29.3397630206672,-6.74355070471993));
#63824=CARTESIAN_POINT('Ctrl Pts',(165.283952952209,-31.4503181523986,-5.2583438798508));
#63825=CARTESIAN_POINT('Ctrl Pts',(165.245037936716,-33.5359341822839,-1.34800299949518));
#63826=CARTESIAN_POINT('Ctrl Pts',(165.260697253294,-32.6650132027678,3.89276739165126));
#63827=CARTESIAN_POINT('Ctrl Pts',(165.311961153447,-30.1017915210122,6.35625687486414));
#63828=CARTESIAN_POINT('Ctrl Pts',(165.346644572269,-28.5778515481473,7.13078505628243));
#63829=CARTESIAN_POINT('Ctrl Pts',(165.840927381346,-28.7234819145522,-7.42360430934041));
#63830=CARTESIAN_POINT('Ctrl Pts',(165.836034823858,-29.513349592714,-7.02017547577061));
#63831=CARTESIAN_POINT('Ctrl Pts',(165.823059613978,-31.7020874460943,-5.47308574876475));
#63832=CARTESIAN_POINT('Ctrl Pts',(165.811523533138,-33.8655876024517,-1.40269845885163));
#63833=CARTESIAN_POINT('Ctrl Pts',(165.816213733456,-32.9621300679948,4.05114677465934));
#63834=CARTESIAN_POINT('Ctrl Pts',(165.831141514884,-30.3033385927089,6.61668467647285));
#63835=CARTESIAN_POINT('Ctrl Pts',(165.840927381346,-28.7234819145522,7.4236043093404));
#63836=CARTESIAN_POINT('Ctrl Pts',(166.,-28.9052030359509,-7.78899131169736));
#63837=CARTESIAN_POINT('Ctrl Pts',(166.000094314236,-29.7336481538873,-7.37289904880312));
#63838=CARTESIAN_POINT('Ctrl Pts',(166.000251426188,-32.037140331791,-5.76671793879459));
#63839=CARTESIAN_POINT('Ctrl Pts',(166.000460788112,-34.3344462999043,-1.48291769243432));
#63840=CARTESIAN_POINT('Ctrl Pts',(166.000335048298,-33.3729252031548,4.27720053179844));
#63841=CARTESIAN_POINT('Ctrl Pts',(166.000188642958,-30.5622205190616,6.95674287510774));
#63842=CARTESIAN_POINT('Ctrl Pts',(166.,-28.9052030359509,7.78899131169735));
#63843=CARTESIAN_POINT('Ctrl Pts',(166.,-29.01481732334,-8.00939296658655));
#63844=CARTESIAN_POINT('Ctrl Pts',(166.,-29.8666447765897,-7.58574615089736));
#63845=CARTESIAN_POINT('Ctrl Pts',(166.,-32.2396668677417,-5.94429110561436));
#63846=CARTESIAN_POINT('Ctrl Pts',(166.,-34.6184184465404,-1.53153797601441));
#63847=CARTESIAN_POINT('Ctrl Pts',(166.,-33.621480950174,4.41413307648097));
#63848=CARTESIAN_POINT('Ctrl Pts',(166.,-30.7186030685495,7.16203426404533));
#63849=CARTESIAN_POINT('Ctrl Pts',(166.,-29.0148173233401,8.00939296658655));
#63850=CARTESIAN_POINT('Origin',(165.,7.57107088371364,-29.1322653714706));
#63851=CARTESIAN_POINT('Origin',(165.,7.57107088371364,-29.1322653714706));
#63852=CARTESIAN_POINT('',(164.948224876262,7.57107088371364,-28.1336066026402));
#63853=CARTESIAN_POINT('Origin',(165.,7.57107088371364,-29.1322653714706));
#63854=CARTESIAN_POINT('',(165.,7.57107088371364,-28.1322653714706));
#63855=CARTESIAN_POINT('Origin',(165.,7.57107088371364,-29.1322653714706));
#63856=CARTESIAN_POINT('Origin',(165.,7.57107088371364,-29.1322653714706));
#63857=CARTESIAN_POINT('Origin',(165.,0.,0.));
#63858=CARTESIAN_POINT('Origin',(158.5,0.,0.));
#63859=CARTESIAN_POINT('Origin',(158.5,0.,0.));
#63860=CARTESIAN_POINT('Ctrl Pts',(164.848300728223,8.11744071408902,-28.3085740825778));
#63861=CARTESIAN_POINT('Ctrl Pts',(162.799301172598,7.77413384506594,-28.4582165837515));
#63862=CARTESIAN_POINT('Ctrl Pts',(157.868889593112,7.48952269386188,-28.6379920043751));
#63863=CARTESIAN_POINT('Ctrl Pts',(152.874056267715,7.50458580396434,-28.6224403563239));
#63864=CARTESIAN_POINT('Ctrl Pts',(150.052788176347,7.63914239096103,-28.5431800801744));
#63865=CARTESIAN_POINT('Ctrl Pts',(164.886050420652,7.8866106465393,-28.1485078205183));
#63866=CARTESIAN_POINT('Ctrl Pts',(162.820942130408,7.53514215381986,-28.2683700222318));
#63867=CARTESIAN_POINT('Ctrl Pts',(157.870887029429,7.25093547801219,-28.3876377102898));
#63868=CARTESIAN_POINT('Ctrl Pts',(152.871700869076,7.26493835968652,-28.3795332220805));
#63869=CARTESIAN_POINT('Ctrl Pts',(150.041115769415,7.39989458347467,-28.3250644260708));
#63870=CARTESIAN_POINT('Ctrl Pts',(164.942784454705,7.58820374369006,-28.0945941257965));
#63871=CARTESIAN_POINT('Ctrl Pts',(162.857424103711,7.20825451719726,-28.1970512908879));
#63872=CARTESIAN_POINT('Ctrl Pts',(157.876641728405,6.87710112890612,-28.2763308833792));
#63873=CARTESIAN_POINT('Ctrl Pts',(152.866254061663,6.89616072826954,-28.2730904566236));
#63874=CARTESIAN_POINT('Ctrl Pts',(150.020705033617,7.05080167669808,-28.2347430874533));
#63875=CARTESIAN_POINT('Ctrl Pts',(165.,7.31954028957033,-28.1644160235812));
#63876=CARTESIAN_POINT('Ctrl Pts',(162.894354921365,6.91344062208961,-28.2699556831011));
#63877=CARTESIAN_POINT('Ctrl Pts',(157.882579751756,6.54039874786384,-28.3550078873843));
#63878=CARTESIAN_POINT('Ctrl Pts',(152.860692060566,6.56397499464613,-28.3505838425905));
#63879=CARTESIAN_POINT('Ctrl Pts',(150.,6.73628528150279,-28.3095824873171));
#63880=CARTESIAN_POINT('',(150.052788176347,7.63914239096103,-28.5431800801744));
#63881=CARTESIAN_POINT('Ctrl Pts',(164.848300728223,8.11744071408902,-28.3085740825778));
#63882=CARTESIAN_POINT('Ctrl Pts',(162.799301172598,7.77413384506594,-28.4582165837515));
#63883=CARTESIAN_POINT('Ctrl Pts',(157.868889593112,7.48952269386188,-28.6379920043751));
#63884=CARTESIAN_POINT('Ctrl Pts',(152.874056267715,7.50458580396434,-28.6224403563239));
#63885=CARTESIAN_POINT('Ctrl Pts',(150.052788176347,7.63914239096103,-28.5431800801744));
#63886=CARTESIAN_POINT('Origin',(150.,6.9677727482211,-29.2824203734792));
#63887=CARTESIAN_POINT('Origin',(165.,0.,0.));
#63888=CARTESIAN_POINT('',(165.,-4.89858719658941E-15,40.));
#63889=CARTESIAN_POINT('Origin',(165.,-4.77612251667468E-15,39.));
#63890=CARTESIAN_POINT('',(165.,-40.,-4.89858719658941E-15));
#63891=CARTESIAN_POINT('Origin',(165.,0.,0.));
#63892=CARTESIAN_POINT('Origin',(165.,0.,0.));
#63893=CARTESIAN_POINT('Origin',(158.,0.,0.));
#63894=CARTESIAN_POINT('',(158.,-40.,-4.89858719658941E-15));
#63895=CARTESIAN_POINT('Ctrl Pts',(127.110025063046,4.72714558106216,-19.086779631978));
#63896=CARTESIAN_POINT('Ctrl Pts',(126.561429494173,8.02431030058917,-17.6122811959622));
#63897=CARTESIAN_POINT('Ctrl Pts',(126.561429494173,11.2405277840037,-15.7553971661405));
#63898=CARTESIAN_POINT('Ctrl Pts',(127.110025063046,14.1660632471972,-13.6372179765762));
#63899=CARTESIAN_POINT('Ctrl Pts',(127.362931194533,4.69027583156377,-18.9102390443581));
#63900=CARTESIAN_POINT('Ctrl Pts',(126.820035970396,7.95318135743582,-17.4510612715844));
#63901=CARTESIAN_POINT('Ctrl Pts',(126.820035970396,11.1364717054729,-15.6131877322364));
#63902=CARTESIAN_POINT('Ctrl Pts',(127.362931194533,14.0316094882686,-13.5170175430695));
#63903=CARTESIAN_POINT('Ctrl Pts',(127.647216190801,4.5139354253642,-18.4101497684479));
#63904=CARTESIAN_POINT('Ctrl Pts',(127.114082771492,7.71817070628305,-16.9772089182626));
#63905=CARTESIAN_POINT('Ctrl Pts',(127.114082771492,10.8436088554295,-15.1727363615173));
#63906=CARTESIAN_POINT('Ctrl Pts',(127.647216190801,13.68668967427,-13.1142576336319));
#63907=CARTESIAN_POINT('Ctrl Pts',(127.47007422846,4.26449742359621,-17.9182815739338));
#63908=CARTESIAN_POINT('Ctrl Pts',(126.939976553095,7.45048380741851,-16.4935013967584));
#63909=CARTESIAN_POINT('Ctrl Pts',(126.939976553095,10.5585493032376,-14.6990589460883));
#63910=CARTESIAN_POINT('Ctrl Pts',(127.47007422846,13.3854383233911,-12.6523038901745));
#63911=CARTESIAN_POINT('Ctrl Pts',(127.328278974586,4.16988910307852,-17.759481155498));
#63912=CARTESIAN_POINT('Ctrl Pts',(126.797908764162,7.35751182232714,-16.3339692437331));
#63913=CARTESIAN_POINT('Ctrl Pts',(126.797908764162,10.466876398543,-14.5387767686462));
#63914=CARTESIAN_POINT('Ctrl Pts',(127.328278974586,13.295217287153,-12.4909704719789));
#63915=CARTESIAN_POINT('',(126.797085404885,7.22587406965037,-17.8889246286188));
#63916=CARTESIAN_POINT('',(126.797085404885,11.8793261399439,-15.2022528231738));
#63917=CARTESIAN_POINT('Ctrl Pts',(126.797739711515,7.22571363751863,-17.8885054447156));
#63918=CARTESIAN_POINT('Ctrl Pts',(126.66552461135,8.81747024270326,-17.0729251722985));
#63919=CARTESIAN_POINT('Ctrl Pts',(126.66552461135,10.3768517947697,-16.1726158134436));
#63920=CARTESIAN_POINT('Ctrl Pts',(126.797739711515,11.8790433321007,-15.2019042929206));
#63921=CARTESIAN_POINT('Ctrl Pts',(127.464921070561,13.2136059641945,-13.0809596303012));
#63922=CARTESIAN_POINT('Ctrl Pts',(127.468398487984,13.2114843263169,-13.1362337935814));
#63923=CARTESIAN_POINT('Ctrl Pts',(127.468025475828,13.2054546036853,-13.1918153340334));
#63924=CARTESIAN_POINT('Ctrl Pts',(127.456769054766,13.1725031106176,-13.3941266074234));
#63925=CARTESIAN_POINT('Ctrl Pts',(127.42748640474,13.1237772459311,-13.5583757980013));
#63926=CARTESIAN_POINT('Ctrl Pts',(127.322999545003,12.9522161781223,-13.9460981797133));
#63927=CARTESIAN_POINT('Ctrl Pts',(127.242195860578,12.8203888695307,-14.1686159650804));
#63928=CARTESIAN_POINT('Ctrl Pts',(127.036712854442,12.4382731297879,-14.6690054235001));
#63929=CARTESIAN_POINT('Ctrl Pts',(126.913668527289,12.1842802549694,-14.9349942415373));
#63930=CARTESIAN_POINT('Ctrl Pts',(126.797085404885,11.8793261399438,-15.2022528231739));
#63931=CARTESIAN_POINT('',(127.464921070561,4.72164036362224,-17.9837982557406));
#63932=CARTESIAN_POINT('Ctrl Pts',(127.328278974586,4.16988910307852,-17.759481155498));
#63933=CARTESIAN_POINT('Ctrl Pts',(127.328985683083,4.17159829889053,-17.7599820161488));
#63934=CARTESIAN_POINT('Ctrl Pts',(127.32968995021,4.17330794090804,-17.760484806387));
#63935=CARTESIAN_POINT('Ctrl Pts',(127.404564207119,4.35574867194381,-17.8143308393859));
#63936=CARTESIAN_POINT('Ctrl Pts',(127.45225052705,4.54335712491858,-17.8897928354479));
#63937=CARTESIAN_POINT('Ctrl Pts',(127.464921070561,4.72164036362224,-17.9837982557406));
#63938=CARTESIAN_POINT('Ctrl Pts',(127.464921070561,4.72164036362224,-17.9837982557406));
#63939=CARTESIAN_POINT('Ctrl Pts',(127.468732665988,4.77527212588831,-18.0120772817978));
#63940=CARTESIAN_POINT('Ctrl Pts',(127.468147721065,4.8349505944349,-18.0382766644184));
#63941=CARTESIAN_POINT('Ctrl Pts',(127.449453154144,5.08072944985862,-18.1261937520205));
#63942=CARTESIAN_POINT('Ctrl Pts',(127.402571734862,5.30241833367094,-18.1693636982815));
#63943=CARTESIAN_POINT('Ctrl Pts',(127.213728487718,5.97308976443218,-18.1944930288535));
#63944=CARTESIAN_POINT('Ctrl Pts',(127.043341092093,6.44608398123035,-18.1278551006546));
#63945=CARTESIAN_POINT('Ctrl Pts',(126.8466194568,7.06489842961485,-17.9421164691797));
#63946=CARTESIAN_POINT('Ctrl Pts',(126.821482537214,7.14552980179911,-17.9162275739827));
#63947=CARTESIAN_POINT('Ctrl Pts',(126.797085404885,7.22587406965033,-17.8889246286188));
#63948=CARTESIAN_POINT('Ctrl Pts',(150.052788176357,7.63914239116794,-28.5431800803631));
#63949=CARTESIAN_POINT('Ctrl Pts',(146.270211476078,7.81947858833029,-28.4368505439864));
#63950=CARTESIAN_POINT('Ctrl Pts',(137.492178857757,7.56977128370464,-26.6032877746526));
#63951=CARTESIAN_POINT('Ctrl Pts',(130.307399857943,5.92914146991218,-21.3918099845279));
#63952=CARTESIAN_POINT('Ctrl Pts',(127.223161057304,4.62069507309358,-17.6980789259149));
#63953=CARTESIAN_POINT('Ctrl Pts',(150.041124530135,7.39989439113665,-28.3250648769978));
#63954=CARTESIAN_POINT('Ctrl Pts',(146.296085688653,7.57964096956798,-28.2546237100009));
#63955=CARTESIAN_POINT('Ctrl Pts',(137.573627372765,7.35172410465697,-26.5132063436706));
#63956=CARTESIAN_POINT('Ctrl Pts',(130.379397788771,5.7587042375174,-21.3658595806507));
#63957=CARTESIAN_POINT('Ctrl Pts',(127.284956078127,4.47631553952171,-17.6939861612586));
#63958=CARTESIAN_POINT('Ctrl Pts',(150.020722457357,7.05080162839574,-28.2347435757426));
#63959=CARTESIAN_POINT('Ctrl Pts',(146.304992407354,7.25777004086244,-28.1861302632078));
#63960=CARTESIAN_POINT('Ctrl Pts',(137.620797808064,7.09907364066923,-26.4971349507024));
#63961=CARTESIAN_POINT('Ctrl Pts',(130.420987560279,5.57091977265869,-21.3784706071926));
#63962=CARTESIAN_POINT('Ctrl Pts',(127.32129741028,4.32046304628092,-17.7152141200869));
#63963=CARTESIAN_POINT('Ctrl Pts',(150.000022383365,6.73628528178713,-28.3095824877733));
#63964=CARTESIAN_POINT('Ctrl Pts',(146.292010366741,6.96723340927544,-28.2545429015207));
#63965=CARTESIAN_POINT('Ctrl Pts',(137.621331189602,6.86523720578075,-26.5551071049148));
#63966=CARTESIAN_POINT('Ctrl Pts',(130.426320545001,5.39188507143624,-21.4274846959551));
#63967=CARTESIAN_POINT('Ctrl Pts',(127.328278974586,4.16988910307942,-17.7594811554977));
#63968=CARTESIAN_POINT('',(127.849160658792,4.87571718501768,-18.4228377223367));
#63969=CARTESIAN_POINT('Ctrl Pts',(150.052788176357,7.63914239116794,-28.5431800803631));
#63970=CARTESIAN_POINT('Ctrl Pts',(146.270211476078,7.81947858833029,-28.4368505439864));
#63971=CARTESIAN_POINT('Ctrl Pts',(137.824456084703,7.57922352139125,-26.6726941187524));
#63972=CARTESIAN_POINT('Ctrl Pts',(130.853617522557,6.05135486105244,-21.7815128093462));
#63973=CARTESIAN_POINT('Ctrl Pts',(127.84939066713,4.87581470102322,-18.4225978736884));
#63974=CARTESIAN_POINT('Ctrl Pts',(127.464959790637,4.72165726174929,-17.9837590795911));
#63975=CARTESIAN_POINT('Ctrl Pts',(127.59147410695,4.77365180283685,-18.1312277406873));
#63976=CARTESIAN_POINT('Ctrl Pts',(127.719628690953,4.8250394361776,-18.2775158073745));
#63977=CARTESIAN_POINT('Ctrl Pts',(127.84939066713,4.87581470102322,-18.4225978736884));
#63978=CARTESIAN_POINT('Origin',(43.,10.6623800874337,1.24625349616492));
#63979=CARTESIAN_POINT('',(43.,11.5,0.7));
#63980=CARTESIAN_POINT('',(43.,11.5,0.7));
#63981=CARTESIAN_POINT('',(43.,11.3514471211877,1.97095110413219));
#63982=CARTESIAN_POINT('Origin',(43.,10.6623800874337,1.24625349616492));
#63983=CARTESIAN_POINT('',(43.,11.3514471211877,1.97095110413219));
#63984=CARTESIAN_POINT('Origin',(43.,12.7,0.));
#63985=CARTESIAN_POINT('',(43.,11.5,-0.7));
#63986=CARTESIAN_POINT('',(43.,11.5,0.35));
#63987=CARTESIAN_POINT('',(43.,11.3514471211877,-1.97095110413219));
#63988=CARTESIAN_POINT('Origin',(43.,10.6623800874337,-1.24625349616493));
#63989=CARTESIAN_POINT('',(43.,11.0285849021483,-3.33321392294394));
#63990=CARTESIAN_POINT('',(43.,11.608447933401,-0.886579411698658));
#63991=CARTESIAN_POINT('',(43.,10.5909347898596,-4.53564772407893));
#63992=CARTESIAN_POINT('Origin',(43.,10.0875684170659,-3.67157463993583));
#63993=CARTESIAN_POINT('',(43.,9.96261593757892,-5.78673342053171));
#63994=CARTESIAN_POINT('',(43.,11.7128765481331,-2.30167801119486));
#63995=CARTESIAN_POINT('',(43.,9.25946242264882,-6.85582640121192));
#63996=CARTESIAN_POINT('Origin',(43.,8.96893332226436,-5.89896024451612));
#63997=CARTESIAN_POINT('',(43.,8.35955976908767,-7.92828862157849));
#63998=CARTESIAN_POINT('',(43.,11.658153795166,-3.9971773404898));
#63999=CARTESIAN_POINT('',(43.,7.42881003951057,-8.80640570249106));
#64000=CARTESIAN_POINT('Origin',(43.,7.36678071053767,-7.8083313754256));
#64001=CARTESIAN_POINT('',(43.,6.30583756965351,-9.64242773087496));
#64002=CARTESIAN_POINT('',(43.,11.233667185904,-5.97379450798535));
#64003=CARTESIAN_POINT('',(43.,5.19766858426649,-10.2822293928957));
#64004=CARTESIAN_POINT('Origin',(43.,5.36748304388578,-9.29675334077463));
#64005=CARTESIAN_POINT('',(43.,3.91216603463411,-10.8367410653506));
#64006=CARTESIAN_POINT('',(43.,10.2301101470916,-8.11144599901502));
#64007=CARTESIAN_POINT('',(43.,2.68631947027824,-11.2037354352735));
#64008=CARTESIAN_POINT('Origin',(43.,3.07882297701681,-10.2839849271476));
#64009=CARTESIAN_POINT('',(43.,1.30758861606115,-11.4468428840072));
#64010=CARTESIAN_POINT('',(43.,8.50016082771923,-10.178598342398));
#64011=CARTESIAN_POINT('',(43.,0.0301501783194109,-11.5212452003569));
#64012=CARTESIAN_POINT('Origin',(43.,0.624182766533234,-10.7168042241878));
#64013=CARTESIAN_POINT('',(43.,-1.36748124326036,-11.4398424398823));
#64014=CARTESIAN_POINT('',(43.,6.00927410875514,-11.8694895125859));
#64015=CARTESIAN_POINT('',(43.,-2.6276445175567,-11.2176416545259));
#64016=CARTESIAN_POINT('Origin',(43.,-1.86410729845783,-10.5718778315606));
#64017=CARTESIAN_POINT('',(43.,-3.96882983479838,-10.8161171287304));
#64018=CARTESIAN_POINT('',(43.,2.86473295436895,-12.8619515284518));
#64019=CARTESIAN_POINT('',(43.,-5.1437822173509,-10.309292143521));
#64020=CARTESIAN_POINT('Origin',(43.,-4.25190285648285,-9.85701876860538));
#64021=CARTESIAN_POINT('',(43.,-6.35621778264911,-9.60929214352104));
#64022=CARTESIAN_POINT('',(43.,-0.684391108675454,-12.8839228005366));
#64023=CARTESIAN_POINT('',(43.,-7.3826172863893,-8.84516602459817));
#64024=CARTESIAN_POINT('Origin',(43.,-6.41047723095084,-8.61076527244045));
#64025=CARTESIAN_POINT('',(43.,-8.40094038459157,-7.88442773158195));
#64026=CARTESIAN_POINT('',(43.,-4.27758822914911,-11.7746098538554));
#64027=CARTESIAN_POINT('',(43.,-9.22345354659921,-6.90419471580332));
#64028=CARTESIAN_POINT('Origin',(43.,-8.22346111860809,-6.90030319162475));
#64029=CARTESIAN_POINT('',(43.,-9.99276611589833,-5.73451177982521));
#64030=CARTESIAN_POINT('',(43.,-7.49833494609831,-9.52711012115367));
#64031=CARTESIAN_POINT('',(43.,-10.56705103871,-4.59101648279533));
#64032=CARTESIAN_POINT('Origin',(43.,-9.5931160887976,-4.81784397967164));
#64033=CARTESIAN_POINT('',(43.,-11.0458792393659,-3.27544681369505));
#64034=CARTESIAN_POINT('',(43.,-9.94394919577672,-6.30297472627502));
#64035=CARTESIAN_POINT('',(43.,-11.3409760741447,-2.03033536285951));
#64036=CARTESIAN_POINT('Origin',(43.,-10.4456036875545,-2.47565355172201));
#64037=CARTESIAN_POINT('',(43.,-11.50350615392,-0.639801662020786));
#64038=CARTESIAN_POINT('',(43.,-11.2960260581795,-2.41490732725707));
#64039=CARTESIAN_POINT('',(43.,-11.50350615392,0.639801662020789));
#64040=CARTESIAN_POINT('Origin',(43.,-10.7349660877716,1.38777878078145E-15));
#64041=CARTESIAN_POINT('',(43.,-11.3409760741447,2.03033536285951));
#64042=CARTESIAN_POINT('',(43.,-11.3772910980671,1.71964047683772));
#64043=CARTESIAN_POINT('',(43.,-11.0458792393659,3.27544681369506));
#64044=CARTESIAN_POINT('Origin',(43.,-10.4456036875545,2.47565355172201));
#64045=CARTESIAN_POINT('',(43.,-10.56705103871,4.59101648279533));
#64046=CARTESIAN_POINT('',(43.,-10.1833632961047,5.64518989172489));
#64047=CARTESIAN_POINT('',(43.,-9.99276611589833,5.73451177982522));
#64048=CARTESIAN_POINT('Origin',(43.,-9.5931160887976,4.81784397967164));
#64049=CARTESIAN_POINT('',(43.,-9.2234535465992,6.90419471580333));
#64050=CARTESIAN_POINT('',(43.,-7.88299123074787,8.94226865316461));
#64051=CARTESIAN_POINT('',(43.,-8.40094038459157,7.88442773158195));
#64052=CARTESIAN_POINT('Origin',(43.,-8.22346111860809,6.90030319162475));
#64053=CARTESIAN_POINT('',(43.,-7.3826172863893,8.84516602459817));
#64054=CARTESIAN_POINT('',(43.,-4.78674977825024,11.2942407073473));
#64055=CARTESIAN_POINT('',(43.,-6.3562177826491,9.60929214352105));
#64056=CARTESIAN_POINT('Origin',(43.,-6.41047723095084,8.61076527244046));
#64057=CARTESIAN_POINT('',(43.,-5.14378221735089,10.309292143521));
#64058=CARTESIAN_POINT('',(43.,-1.29060889132455,12.5339228005366));
#64059=CARTESIAN_POINT('',(43.,-3.96882983479838,10.8161171287304));
#64060=CARTESIAN_POINT('Origin',(43.,-4.25190285648284,9.85701876860538));
#64061=CARTESIAN_POINT('',(43.,-2.62764451755669,11.2176416545259));
#64062=CARTESIAN_POINT('',(43.,2.19414029574811,12.6611892655541));
#64063=CARTESIAN_POINT('',(43.,-1.36748124326036,11.4398424398823));
#64064=CARTESIAN_POINT('Origin',(43.,-1.86410729845783,10.5718778315606));
#64065=CARTESIAN_POINT('',(43.,0.0301501783194164,11.5212452003569));
#64066=CARTESIAN_POINT('',(43.,5.31045839796525,11.8287881323485));
#64067=CARTESIAN_POINT('',(43.,1.30758861606115,11.4468428840072));
#64068=CARTESIAN_POINT('Origin',(43.,0.624182766533239,10.7168042241878));
#64069=CARTESIAN_POINT('',(43.,2.68631947027825,11.2037354352735));
#64070=CARTESIAN_POINT('',(43.,7.81079540061069,10.3001520667648));
#64071=CARTESIAN_POINT('',(43.,3.91216603463411,10.8367410653506));
#64072=CARTESIAN_POINT('Origin',(43.,3.07882297701681,10.2839849271476));
#64073=CARTESIAN_POINT('',(43.,5.1976685842665,10.2822293928957));
#64074=CARTESIAN_POINT('',(43.,9.58735887227544,8.38870183524243));
#64075=CARTESIAN_POINT('',(43.,6.30583756965351,9.64242773087495));
#64076=CARTESIAN_POINT('Origin',(43.,5.36748304388578,9.29675334077463));
#64077=CARTESIAN_POINT('',(43.,7.42881003951057,8.80640570249105));
#64078=CARTESIAN_POINT('',(43.,10.6721809509755,6.3918055221773));
#64079=CARTESIAN_POINT('',(43.,8.35955976908767,7.92828862157849));
#64080=CARTESIAN_POINT('Origin',(43.,7.36678071053768,7.80833137542559));
#64081=CARTESIAN_POINT('',(43.,9.25946242264883,6.85582640121192));
#64082=CARTESIAN_POINT('',(43.,11.2082024683855,4.53340845067308));
#64083=CARTESIAN_POINT('',(43.,9.96261593757892,5.7867334205317));
#64084=CARTESIAN_POINT('Origin',(43.,8.96893332226436,5.89896024451612));
#64085=CARTESIAN_POINT('',(43.,10.5909347898596,4.53564772407893));
#64086=CARTESIAN_POINT('',(43.,11.3987171219927,2.92722085942124));
#64087=CARTESIAN_POINT('',(43.,11.0285849021483,3.33321392294394));
#64088=CARTESIAN_POINT('Origin',(43.,10.0875684170659,3.67157463993582));
#64089=CARTESIAN_POINT('',(43.,11.4470168238813,1.56771082110453));
#64090=CARTESIAN_POINT('',(43.,-10.9193372788466,-0.35170782020184));
#64091=CARTESIAN_POINT('Origin',(43.,0.,0.));
#64092=CARTESIAN_POINT('Ctrl Pts',(43.,-10.9197403196571,-0.351952921252014));
#64093=CARTESIAN_POINT('Ctrl Pts',(43.,-10.9014607692317,-0.616218838015593));
#64094=CARTESIAN_POINT('Ctrl Pts',(43.,-10.8735485015388,-0.879472507464425));
#64095=CARTESIAN_POINT('Ctrl Pts',(43.,-10.8359390630765,-1.14119506822165));
#64096=CARTESIAN_POINT('Ctrl Pts',(43.,-10.8317883291396,-1.17007985776925));
#64097=CARTESIAN_POINT('Ctrl Pts',(43.,-10.8275194292063,-1.19894599289931));
#64098=CARTESIAN_POINT('Ctrl Pts',(43.,-10.8231322378448,-1.22779277132606));
#64099=CARTESIAN_POINT('Ctrl Pts',(43.,-10.7832837165566,-1.48980583834688));
#64100=CARTESIAN_POINT('Ctrl Pts',(43.,-10.733680401679,-1.75022311605247));
#64101=CARTESIAN_POINT('Ctrl Pts',(43.,-10.6745492794892,-2.00855052974716));
#64102=CARTESIAN_POINT('Ctrl Pts',(43.,-10.6320176199436,-2.19435951161089));
#64103=CARTESIAN_POINT('Ctrl Pts',(43.,-10.5845555537826,-2.37908709826241));
#64104=CARTESIAN_POINT('Ctrl Pts',(43.,-10.5322319524948,-2.5625435845543));
#64105=CARTESIAN_POINT('Ctrl Pts',(43.,-10.4850643149276,-2.72792228253783));
#64106=CARTESIAN_POINT('Ctrl Pts',(43.,-10.433945856036,-2.89226804048928));
#64107=CARTESIAN_POINT('Ctrl Pts',(43.,-10.3789185342256,-3.05543717466525));
#64108=CARTESIAN_POINT('Ctrl Pts',(43.,-10.3670683111114,-3.09057591269074));
#64109=CARTESIAN_POINT('Ctrl Pts',(43.,-10.3550363388042,-3.12566118761188));
#64110=CARTESIAN_POINT('Ctrl Pts',(43.,-10.3428289092764,-3.16067498608578));
#64111=CARTESIAN_POINT('Ctrl Pts',(43.,-10.2560596566836,-3.4095497485478));
#64112=CARTESIAN_POINT('Ctrl Pts',(43.,-10.1603659384729,-3.65500749223555));
#64113=CARTESIAN_POINT('Ctrl Pts',(43.,-10.0559781323561,-3.89656626265814));
#64114=CARTESIAN_POINT('Ctrl Pts',(43.,-9.9517959085899,-4.13764930491213));
#64115=CARTESIAN_POINT('Ctrl Pts',(43.,-9.83895351073254,-4.3748492901464));
#64116=CARTESIAN_POINT('Ctrl Pts',(43.,-9.71763349467765,-4.60766478312798));
#64117=CARTESIAN_POINT('Ctrl Pts',(43.,-9.59726776727907,-4.83864897744018));
#64118=CARTESIAN_POINT('Ctrl Pts',(43.,-9.46855694844644,-5.06531790864065));
#64119=CARTESIAN_POINT('Ctrl Pts',(43.,-9.33163817279928,-5.28715174611257));
#64120=CARTESIAN_POINT('Ctrl Pts',(43.,-9.28608468637509,-5.36095685177423));
#64121=CARTESIAN_POINT('Ctrl Pts',(43.,-9.23962232350255,-5.43422646696429));
#64122=CARTESIAN_POINT('Ctrl Pts',(43.,-9.19225520434974,-5.50694054568881));
#64123=CARTESIAN_POINT('Ctrl Pts',(43.,-9.1763218189465,-5.53140015947325));
#64124=CARTESIAN_POINT('Ctrl Pts',(43.,-9.16028605483618,-5.55579690911195));
#64125=CARTESIAN_POINT('Ctrl Pts',(43.,-9.14414805757597,-5.58013001893356));
#64126=CARTESIAN_POINT('Ctrl Pts',(43.,-9.12682372198913,-5.60625190714708));
#64127=CARTESIAN_POINT('Ctrl Pts',(43.,-9.10938647108694,-5.63229304613623));
#64128=CARTESIAN_POINT('Ctrl Pts',(43.,-9.09183870028264,-5.65824965886696));
#64129=CARTESIAN_POINT('Ctrl Pts',(43.,-8.98393008387962,-5.81786777774479));
#64130=CARTESIAN_POINT('Ctrl Pts',(43.,-8.87181893682748,-5.97432674016409));
#64131=CARTESIAN_POINT('Ctrl Pts',(43.,-8.75559238782109,-6.12744097842411));
#64132=CARTESIAN_POINT('Ctrl Pts',(43.,-8.59880957249742,-6.33398312861068));
#64133=CARTESIAN_POINT('Ctrl Pts',(43.,-8.43453971721519,-6.53444056558063));
#64134=CARTESIAN_POINT('Ctrl Pts',(43.,-8.26323653110453,-6.72852936150831));
#64135=CARTESIAN_POINT('Ctrl Pts',(43.,-8.0908916379292,-6.92379842544197));
#64136=CARTESIAN_POINT('Ctrl Pts',(43.,-7.9114271172275,-7.1126215757687));
#64137=CARTESIAN_POINT('Ctrl Pts',(43.,-7.72526608652512,-7.29467382738674));
#64138=CARTESIAN_POINT('Ctrl Pts',(43.,-7.53933348235205,-7.47650269410068));
#64139=CARTESIAN_POINT('Ctrl Pts',(43.,-7.34672025960377,-7.65157764909177));
#64140=CARTESIAN_POINT('Ctrl Pts',(43.,-7.1478170672538,-7.81953330954781));
#64141=CARTESIAN_POINT('Ctrl Pts',(43.,-6.96131195004891,-7.97701992285196));
#64142=CARTESIAN_POINT('Ctrl Pts',(43.,-6.76927594057254,-8.12824700157048));
#64143=CARTESIAN_POINT('Ctrl Pts',(43.,-6.57201255029189,-8.27287550401205));
#64144=CARTESIAN_POINT('Ctrl Pts',(43.,-6.49803877893665,-8.32711119242764));
#64145=CARTESIAN_POINT('Ctrl Pts',(43.,-6.42332975640829,-8.38041856443647));
#64146=CARTESIAN_POINT('Ctrl Pts',(43.,-6.34790100699426,-8.43277828285923));
#64147=CARTESIAN_POINT('Ctrl Pts',(43.,-6.31913166008323,-8.4527488499861));
#64148=CARTESIAN_POINT('Ctrl Pts',(43.,-6.29025760914184,-8.47258154931832));
#64149=CARTESIAN_POINT('Ctrl Pts',(43.,-6.26127970757771,-8.49227527579303));
#64150=CARTESIAN_POINT('Ctrl Pts',(43.,-6.24095851801632,-8.50608579785506));
#64151=CARTESIAN_POINT('Ctrl Pts',(43.,-6.22058756344042,-8.51982706261644));
#64152=CARTESIAN_POINT('Ctrl Pts',(43.,-6.20017500510534,-8.53349353441625));
#64153=CARTESIAN_POINT('Ctrl Pts',(43.,-5.98558578372535,-8.67716379340047));
#64154=CARTESIAN_POINT('Ctrl Pts',(43.,-5.76616234888234,-8.81273463764936));
#64155=CARTESIAN_POINT('Ctrl Pts',(43.,-5.54232609839399,-8.93991302101306));
#64156=CARTESIAN_POINT('Ctrl Pts',(43.,-5.31902082184162,-9.06678971773467));
#64157=CARTESIAN_POINT('Ctrl Pts',(43.,-5.09132310262944,-9.18531406818114));
#64158=CARTESIAN_POINT('Ctrl Pts',(43.,-4.8596233184157,-9.29515173524445));
#64159=CARTESIAN_POINT('Ctrl Pts',(43.,-4.79898194670169,-9.32389887810084));
#64160=CARTESIAN_POINT('Ctrl Pts',(43.,-4.73806631055322,-9.35205074173778));
#64161=CARTESIAN_POINT('Ctrl Pts',(43.,-4.67688316078947,-9.37960079431053));
#64162=CARTESIAN_POINT('Ctrl Pts',(43.,-4.44223905403518,-9.48525827520075));
#64163=CARTESIAN_POINT('Ctrl Pts',(43.,-4.20366139748706,-9.58206820829766));
#64164=CARTESIAN_POINT('Ctrl Pts',(43.,-3.9616792944636,-9.66993875920283));
#64165=CARTESIAN_POINT('Ctrl Pts',(43.,-3.72019372066151,-9.75762900629348));
#64166=CARTESIAN_POINT('Ctrl Pts',(43.,-3.47531699991253,-9.83641659993009));
#64167=CARTESIAN_POINT('Ctrl Pts',(43.,-3.22756696527006,-9.90615918028994));
#64168=CARTESIAN_POINT('Ctrl Pts',(43.,-3.08207686886982,-9.94711519773066));
#64169=CARTESIAN_POINT('Ctrl Pts',(43.,-2.93559578747511,-9.98495100860572));
#64170=CARTESIAN_POINT('Ctrl Pts',(43.,-2.78822868088063,-10.0196293646901));
#64171=CARTESIAN_POINT('Ctrl Pts',(43.,-2.71775606371211,-10.036212946799));
#64172=CARTESIAN_POINT('Ctrl Pts',(43.,-2.64708083229262,-10.0520743704123));
#64173=CARTESIAN_POINT('Ctrl Pts',(43.,-2.57621452869558,-10.0672090487995));
#64174=CARTESIAN_POINT('Ctrl Pts',(43.,-2.53796933999487,-10.0753769452675));
#64175=CARTESIAN_POINT('Ctrl Pts',(43.,-2.49966302806181,-10.0833342131057));
#64176=CARTESIAN_POINT('Ctrl Pts',(43.,-2.46132915360033,-10.0910738609485));
#64177=CARTESIAN_POINT('Ctrl Pts',(43.,-2.2110408156004,-10.1416073283451));
#64178=CARTESIAN_POINT('Ctrl Pts',(43.,-1.95936197263529,-10.1829167794131));
#64179=CARTESIAN_POINT('Ctrl Pts',(43.,-1.70681513844497,-10.2149618439869));
#64180=CARTESIAN_POINT('Ctrl Pts',(43.,-1.45414125122098,-10.2470230300166));
#64181=CARTESIAN_POINT('Ctrl Pts',(43.,-1.20059784362883,-10.2698105803062));
#64182=CARTESIAN_POINT('Ctrl Pts',(43.,-0.946698749354102,-10.2832327719403));
#64183=CARTESIAN_POINT('Ctrl Pts',(43.,-0.695269585796358,-10.2965243924769));
#64184=CARTESIAN_POINT('Ctrl Pts',(43.,-0.443490997686758,-10.3006319749984));
#64185=CARTESIAN_POINT('Ctrl Pts',(43.,-0.191862227924839,-10.2954157805661));
#64186=CARTESIAN_POINT('Ctrl Pts',(43.,-0.007494890391611,-10.291593896922));
#64187=CARTESIAN_POINT('Ctrl Pts',(43.,0.176792050471349,-10.2827655698261));
#64188=CARTESIAN_POINT('Ctrl Pts',(43.,0.360799239009517,-10.2688582725463));
#64189=CARTESIAN_POINT('Ctrl Pts',(43.,0.571063676741632,-10.2529664475251));
#64190=CARTESIAN_POINT('Ctrl Pts',(43.,0.780963176351545,-10.2304429873017));
#64191=CARTESIAN_POINT('Ctrl Pts',(43.,0.990204189978614,-10.2013572412664));
#64192=CARTESIAN_POINT('Ctrl Pts',(43.,1.08174713344046,-10.1886322273759));
#64193=CARTESIAN_POINT('Ctrl Pts',(43.,1.17316391573373,-10.1746508582186));
#64194=CARTESIAN_POINT('Ctrl Pts',(43.,1.26442930027015,-10.1594176036176));
#64195=CARTESIAN_POINT('Ctrl Pts',(43.,1.32370993252878,-10.1495229763316));
#64196=CARTESIAN_POINT('Ctrl Pts',(43.,1.38292668078725,-10.1391001574367));
#64197=CARTESIAN_POINT('Ctrl Pts',(43.,1.44207252185993,-10.1281501938123));
#64198=CARTESIAN_POINT('Ctrl Pts',(43.,1.4688141036338,-10.1231993918223));
#64199=CARTESIAN_POINT('Ctrl Pts',(43.,1.49554084490732,-10.1181408549116));
#64200=CARTESIAN_POINT('Ctrl Pts',(43.,1.52223858289392,-10.1129774033927));
#64201=CARTESIAN_POINT('Ctrl Pts',(43.,1.76830094160986,-10.0653879386793));
#64202=CARTESIAN_POINT('Ctrl Pts',(43.,2.0121949646504,-10.0088368898019));
#64203=CARTESIAN_POINT('Ctrl Pts',(43.,2.25345797839244,-9.94355576179654));
#64204=CARTESIAN_POINT('Ctrl Pts',(43.,2.50638158642547,-9.87511950140382));
#64205=CARTESIAN_POINT('Ctrl Pts',(43.,2.7564145141448,-9.79708905612276));
#64206=CARTESIAN_POINT('Ctrl Pts',(43.,3.00301114596651,-9.70967187635158));
#64207=CARTESIAN_POINT('Ctrl Pts',(43.,3.23921179421979,-9.62594001684527));
#64208=CARTESIAN_POINT('Ctrl Pts',(43.,3.47226026276032,-9.53359557848944));
#64209=CARTESIAN_POINT('Ctrl Pts',(43.,3.70165663824938,-9.43277251523916));
#64210=CARTESIAN_POINT('Ctrl Pts',(43.,3.92911185657958,-9.33280261896063));
#64211=CARTESIAN_POINT('Ctrl Pts',(43.,4.1529770703731,-9.2244967012555));
#64212=CARTESIAN_POINT('Ctrl Pts',(43.,4.37273672526662,-9.10794286268418));
#64213=CARTESIAN_POINT('Ctrl Pts',(43.,4.58858721508692,-8.99346232639901));
#64214=CARTESIAN_POINT('Ctrl Pts',(43.,4.80047734991067,-8.8710243849871));
#64215=CARTESIAN_POINT('Ctrl Pts',(43.,5.00788410116464,-8.74067580670551));
#64216=CARTESIAN_POINT('Ctrl Pts',(43.,5.04336450532171,-8.71837749572591));
#64217=CARTESIAN_POINT('Ctrl Pts',(43.,5.07871361634502,-8.69584760700039));
#64218=CARTESIAN_POINT('Ctrl Pts',(43.,5.1139286979658,-8.67308627433867));
#64219=CARTESIAN_POINT('Ctrl Pts',(43.,9.86762259782004,2.00332725038414));
#64220=CARTESIAN_POINT('Ctrl Pts',(43.,9.82706698336165,2.25743558012109));
#64221=CARTESIAN_POINT('Ctrl Pts',(43.,9.77677273737292,2.50964253586054));
#64222=CARTESIAN_POINT('Ctrl Pts',(43.,9.716775070148,2.75937815887491));
#64223=CARTESIAN_POINT('Ctrl Pts',(43.,9.65850508348496,3.00192244593501));
#64224=CARTESIAN_POINT('Ctrl Pts',(43.,9.59108241084547,3.24213639852568));
#64225=CARTESIAN_POINT('Ctrl Pts',(43.,9.51481538005978,3.479588668474));
#64226=CARTESIAN_POINT('Ctrl Pts',(43.,9.43805834492817,3.71856653399126));
#64227=CARTESIAN_POINT('Ctrl Pts',(43.,9.35234272165757,3.95474771094638));
#64228=CARTESIAN_POINT('Ctrl Pts',(43.,9.25793113430769,4.18768086760133));
#64229=CARTESIAN_POINT('Ctrl Pts',(43.,9.22821359814858,4.2610002524338));
#64230=CARTESIAN_POINT('Ctrl Pts',(43.,9.19763411850933,4.33399770935435));
#64231=CARTESIAN_POINT('Ctrl Pts',(43.,9.16619988905036,4.40665877998812));
#64232=CARTESIAN_POINT('Ctrl Pts',(43.,9.15308852625325,4.43696604931529));
#64233=CARTESIAN_POINT('Ctrl Pts',(43.,9.13982845171993,4.46721479283657));
#64234=CARTESIAN_POINT('Ctrl Pts',(43.,9.12642016387785,4.49740394982256));
#64235=CARTESIAN_POINT('Ctrl Pts',(43.,9.11247512762385,4.52880161174674));
#64236=CARTESIAN_POINT('Ctrl Pts',(43.,9.0983736369106,4.56012610296547));
#64237=CARTESIAN_POINT('Ctrl Pts',(43.,9.0841176102958,4.59137396666149));
#64238=CARTESIAN_POINT('Ctrl Pts',(43.,8.97497545680003,4.83060325740828));
#64239=CARTESIAN_POINT('Ctrl Pts',(43.,8.85676045078312,5.06538761272098));
#64240=CARTESIAN_POINT('Ctrl Pts',(43.,8.7298267363165,5.2952330977949));
#64241=CARTESIAN_POINT('Ctrl Pts',(43.,8.60727554449511,5.51714292095683));
#64242=CARTESIAN_POINT('Ctrl Pts',(43.,8.47659668546221,5.73444955597585));
#64243=CARTESIAN_POINT('Ctrl Pts',(43.,8.33805798760659,5.94669186954332));
#64244=CARTESIAN_POINT('Ctrl Pts',(43.,8.20001483954325,6.15817499715026));
#64245=CARTESIAN_POINT('Ctrl Pts',(43.,8.0541676735772,6.36463055093452));
#64246=CARTESIAN_POINT('Ctrl Pts',(43.,7.90073639000514,6.56557723205585));
#64247=CARTESIAN_POINT('Ctrl Pts',(43.,7.86221023371319,6.6160343687166));
#64248=CARTESIAN_POINT('Ctrl Pts',(43.,7.82320569071854,6.66614402388867));
#64249=CARTESIAN_POINT('Ctrl Pts',(43.,7.78372582885473,6.71589826069609));
#64250=CARTESIAN_POINT('Ctrl Pts',(43.,7.76082930694455,6.74475345216345));
#64251=CARTESIAN_POINT('Ctrl Pts',(43.,7.73777146386654,6.77349078468606));
#64252=CARTESIAN_POINT('Ctrl Pts',(43.,7.71456760228466,6.8020908181635));
#64253=CARTESIAN_POINT('Ctrl Pts',(43.,7.60014162299007,6.9431271205465));
#64254=CARTESIAN_POINT('Ctrl Pts',(43.,7.48209072299145,7.08092063769054));
#64255=CARTESIAN_POINT('Ctrl Pts',(43.,7.36052755954013,7.21531570044237));
#64256=CARTESIAN_POINT('Ctrl Pts',(43.,7.19168247597401,7.40198364290912));
#64257=CARTESIAN_POINT('Ctrl Pts',(43.,7.01606351231718,7.58209681141095));
#64258=CARTESIAN_POINT('Ctrl Pts',(43.,6.8341706909375,7.75545486785811));
#64259=CARTESIAN_POINT('Ctrl Pts',(43.,6.6502290329696,7.93076562549611));
#64260=CARTESIAN_POINT('Ctrl Pts',(43.,6.45987095725719,8.09916865102304));
#64261=CARTESIAN_POINT('Ctrl Pts',(43.,6.26356944027539,8.26042609800731));
#64262=CARTESIAN_POINT('Ctrl Pts',(43.,6.06626744215104,8.42250541859341));
#64263=CARTESIAN_POINT('Ctrl Pts',(43.,5.86296077545777,8.57736654972914));
#64264=CARTESIAN_POINT('Ctrl Pts',(43.,5.65409234725365,8.7247309754137));
#64265=CARTESIAN_POINT('Ctrl Pts',(43.,5.45601142315324,8.86448441670735));
#64266=CARTESIAN_POINT('Ctrl Pts',(43.,5.25292774258862,8.99749553175811));
#64267=CARTESIAN_POINT('Ctrl Pts',(43.,5.04519439225763,9.12349116326314));
#64268=CARTESIAN_POINT('Ctrl Pts',(43.,4.96729438588352,9.17073952507753));
#64269=CARTESIAN_POINT('Ctrl Pts',(43.,4.88874030973111,9.21700096120252));
#64270=CARTESIAN_POINT('Ctrl Pts',(43.,4.80955009420199,9.26225967137746));
#64271=CARTESIAN_POINT('Ctrl Pts',(43.,4.77331433726708,9.282969093749));
#64272=CARTESIAN_POINT('Ctrl Pts',(43.,4.73694538196408,9.30346855613007));
#64273=CARTESIAN_POINT('Ctrl Pts',(43.,4.70044492410173,9.32375648831331));
#64274=CARTESIAN_POINT('Ctrl Pts',(43.,4.67740974756973,9.33656005645134));
#64275=CARTESIAN_POINT('Ctrl Pts',(43.,4.65432571311928,9.34927739774407));
#64276=CARTESIAN_POINT('Ctrl Pts',(43.,4.63120049512196,9.36190432484467));
#64277=CARTESIAN_POINT('Ctrl Pts',(43.,4.40458184566217,9.48564357637074));
#64278=CARTESIAN_POINT('Ctrl Pts',(43.,4.17380615732999,9.6008173365724));
#64279=CARTESIAN_POINT('Ctrl Pts',(43.,3.939363930894,9.70720197086566));
#64280=CARTESIAN_POINT('Ctrl Pts',(43.,3.70373127349144,9.81412679608339));
#64281=CARTESIAN_POINT('Ctrl Pts',(43.,3.46439423219394,9.91217341639103));
#64282=CARTESIAN_POINT('Ctrl Pts',(43.,3.22181641041172,10.0010753306087));
#64283=CARTESIAN_POINT('Ctrl Pts',(43.,3.17239207733555,10.0191887664832));
#64284=CARTESIAN_POINT('Ctrl Pts',(43.,3.12283311254147,10.0369224403358));
#64285=CARTESIAN_POINT('Ctrl Pts',(43.,3.07314329332181,10.054273874917));
#64286=CARTESIAN_POINT('Ctrl Pts',(43.,2.83048404205589,10.1390092631713));
#64287=CARTESIAN_POINT('Ctrl Pts',(43.,2.58470581263651,10.2146327644165));
#64288=CARTESIAN_POINT('Ctrl Pts',(43.,2.33633929246782,10.2811548119466));
#64289=CARTESIAN_POINT('Ctrl Pts',(43.,2.0868961466204,10.3479652209859));
#64290=CARTESIAN_POINT('Ctrl Pts',(43.,1.83484159807047,10.4055952247248));
#64291=CARTESIAN_POINT('Ctrl Pts',(43.,1.58069736840436,10.4540051740405));
#64292=CARTESIAN_POINT('Ctrl Pts',(43.,1.4271016154715,10.4832624293571));
#64293=CARTESIAN_POINT('Ctrl Pts',(43.,1.27274232725865,10.5091510225733));
#64294=CARTESIAN_POINT('Ctrl Pts',(43.,1.11773335168316,10.5316530667177));
#64295=CARTESIAN_POINT('Ctrl Pts',(43.,1.04846171633564,10.5417089579379));
#64296=CARTESIAN_POINT('Ctrl Pts',(43.,0.979060326232052,10.5510884328026));
#64297=CARTESIAN_POINT('Ctrl Pts',(43.,0.909539329879307,10.5597894422334));
#64298=CARTESIAN_POINT('Ctrl Pts',(43.,0.881400338966954,10.5633112218129));
#64299=CARTESIAN_POINT('Ctrl Pts',(43.,0.853241753393424,10.5667218473265));
#64300=CARTESIAN_POINT('Ctrl Pts',(43.,0.825064246537586,10.5700211697436));
#64301=CARTESIAN_POINT('Ctrl Pts',(43.,0.794409772148462,10.5736105218836));
#64302=CARTESIAN_POINT('Ctrl Pts',(43.,0.763740334040977,10.5770672485921));
#64303=CARTESIAN_POINT('Ctrl Pts',(43.,0.733065052532173,10.5803905207605));
#64304=CARTESIAN_POINT('Ctrl Pts',(43.,0.473684069371478,10.6084911138097));
#64305=CARTESIAN_POINT('Ctrl Pts',(43.,0.213705062438641,10.6270752937871));
#64306=CARTESIAN_POINT('Ctrl Pts',(43.,-0.0463217365835306,10.6361971983038));
#64307=CARTESIAN_POINT('Ctrl Pts',(43.,-0.307829239757041,10.6453710468583));
#64308=CARTESIAN_POINT('Ctrl Pts',(43.,-0.569385716243544,10.644974661583));
#64309=CARTESIAN_POINT('Ctrl Pts',(43.,-0.830448282373223,10.6350128364797));
#64310=CARTESIAN_POINT('Ctrl Pts',(43.,-1.09101112025009,10.6250700803894));
#64311=CARTESIAN_POINT('Ctrl Pts',(43.,-1.35108258972456,10.6055985293602));
#64312=CARTESIAN_POINT('Ctrl Pts',(43.,-1.61012991025001,10.5765518130054));
#64313=CARTESIAN_POINT('Ctrl Pts',(43.,-1.79127941221719,10.5562397009526));
#64314=CARTESIAN_POINT('Ctrl Pts',(43.,-1.97192825321573,10.5312441942016));
#64315=CARTESIAN_POINT('Ctrl Pts',(43.,-2.1518936942779,10.5015342739645));
#64316=CARTESIAN_POINT('Ctrl Pts',(43.,-2.3735990345592,10.4649336469939));
#64317=CARTESIAN_POINT('Ctrl Pts',(43.,-2.5942675670509,10.4211788804489));
#64318=CARTESIAN_POINT('Ctrl Pts',(43.,-2.81360240330237,10.3704040738589));
#64319=CARTESIAN_POINT('Ctrl Pts',(43.,-2.90956139416238,10.3481900959757));
#64320=CARTESIAN_POINT('Ctrl Pts',(43.,-3.00526501584013,10.3246320793819));
#64321=CARTESIAN_POINT('Ctrl Pts',(43.,-3.10068788646092,10.2997396109821));
#64322=CARTESIAN_POINT('Ctrl Pts',(43.,-3.15953825260694,10.2843876217778));
#64323=CARTESIAN_POINT('Ctrl Pts',(43.,-3.21828182563309,10.2685280428291));
#64324=CARTESIAN_POINT('Ctrl Pts',(43.,-3.27691257491908,10.2521629392473));
#64325=CARTESIAN_POINT('Ctrl Pts',(43.,-3.30399262002573,10.2446043160237));
#64326=CARTESIAN_POINT('Ctrl Pts',(43.,-3.33104849368144,10.23693783807));
#64327=CARTESIAN_POINT('Ctrl Pts',(43.,-3.35806590898697,10.2291677543284));
#64328=CARTESIAN_POINT('Ctrl Pts',(43.,-3.60859648607806,10.1571163185484));
#64329=CARTESIAN_POINT('Ctrl Pts',(43.,-3.85611737951388,10.0760782973365));
#64330=CARTESIAN_POINT('Ctrl Pts',(43.,-4.10019229846966,9.98637712440751));
#64331=CARTESIAN_POINT('Ctrl Pts',(43.,-4.34718765047591,9.89560264877618));
#64332=CARTESIAN_POINT('Ctrl Pts',(43.,-4.59065464627726,9.79595632757706));
#64333=CARTESIAN_POINT('Ctrl Pts',(43.,-4.83013745544818,9.68772023928208));
#64334=CARTESIAN_POINT('Ctrl Pts',(43.,-5.07114944708197,9.57879302527063));
#64335=CARTESIAN_POINT('Ctrl Pts',(43.,-5.30812681600379,9.46116580706398));
#64336=CARTESIAN_POINT('Ctrl Pts',(43.,-5.54059227424405,9.33507519504236));
#64337=CARTESIAN_POINT('Ctrl Pts',(43.,-5.77228736148496,9.20940243671621));
#64338=CARTESIAN_POINT('Ctrl Pts',(43.,-5.99950098075074,9.07532202514378));
#64339=CARTESIAN_POINT('Ctrl Pts',(43.,-6.22173909702656,8.93302131478786));
#64340=CARTESIAN_POINT('Ctrl Pts',(43.,-6.44104496712845,8.79259814335498));
#64341=CARTESIAN_POINT('Ctrl Pts',(43.,-6.65550628069746,8.64416985306344));
#64342=CARTESIAN_POINT('Ctrl Pts',(43.,-6.86461922406877,8.48787505619828));
#64343=CARTESIAN_POINT('Ctrl Pts',(43.,-6.92523095564188,8.4425727515148));
#64344=CARTESIAN_POINT('Ctrl Pts',(43.,-6.98539313342641,8.39660929775948));
#64345=CARTESIAN_POINT('Ctrl Pts',(43.,-7.04509292776818,8.3499874634104));
#64346=CARTESIAN_POINT('Origin',(43.,10.0875684170659,3.67157463993582));
#64347=CARTESIAN_POINT('',(43.,11.0285849021483,3.33321392294394));
#64348=CARTESIAN_POINT('',(43.,10.5909347898596,4.53564772407893));
#64349=CARTESIAN_POINT('Origin',(43.,8.96893332226436,5.89896024451612));
#64350=CARTESIAN_POINT('',(43.,9.96261593757892,5.7867334205317));
#64351=CARTESIAN_POINT('',(43.,9.25946242264883,6.85582640121192));
#64352=CARTESIAN_POINT('Origin',(43.,7.36678071053768,7.80833137542559));
#64353=CARTESIAN_POINT('',(43.,8.35955976908767,7.92828862157849));
#64354=CARTESIAN_POINT('',(43.,7.42881003951057,8.80640570249105));
#64355=CARTESIAN_POINT('Origin',(43.,5.36748304388578,9.29675334077463));
#64356=CARTESIAN_POINT('',(43.,6.30583756965351,9.64242773087495));
#64357=CARTESIAN_POINT('',(43.,5.1976685842665,10.2822293928957));
#64358=CARTESIAN_POINT('Origin',(43.,3.07882297701681,10.2839849271476));
#64359=CARTESIAN_POINT('',(43.,3.91216603463411,10.8367410653506));
#64360=CARTESIAN_POINT('',(43.,2.68631947027825,11.2037354352735));
#64361=CARTESIAN_POINT('Origin',(43.,0.624182766533239,10.7168042241878));
#64362=CARTESIAN_POINT('',(43.,1.30758861606115,11.4468428840072));
#64363=CARTESIAN_POINT('',(43.,0.0301501783194164,11.5212452003569));
#64364=CARTESIAN_POINT('Origin',(43.,-1.86410729845783,10.5718778315606));
#64365=CARTESIAN_POINT('',(43.,-1.36748124326036,11.4398424398823));
#64366=CARTESIAN_POINT('',(43.,-2.62764451755669,11.2176416545259));
#64367=CARTESIAN_POINT('Origin',(43.,-4.25190285648284,9.85701876860538));
#64368=CARTESIAN_POINT('',(43.,-3.96882983479838,10.8161171287304));
#64369=CARTESIAN_POINT('',(43.,-5.14378221735089,10.309292143521));
#64370=CARTESIAN_POINT('Origin',(43.,-6.41047723095084,8.61076527244046));
#64371=CARTESIAN_POINT('',(43.,-6.3562177826491,9.60929214352105));
#64372=CARTESIAN_POINT('',(43.,-7.3826172863893,8.84516602459817));
#64373=CARTESIAN_POINT('Origin',(43.,-8.22346111860809,6.90030319162475));
#64374=CARTESIAN_POINT('',(43.,-8.40094038459157,7.88442773158195));
#64375=CARTESIAN_POINT('',(43.,-9.2234535465992,6.90419471580333));
#64376=CARTESIAN_POINT('Origin',(43.,-9.5931160887976,4.81784397967164));
#64377=CARTESIAN_POINT('',(43.,-9.99276611589833,5.73451177982522));
#64378=CARTESIAN_POINT('',(43.,-10.56705103871,4.59101648279533));
#64379=CARTESIAN_POINT('Origin',(43.,-10.4456036875545,2.47565355172201));
#64380=CARTESIAN_POINT('',(43.,-11.0458792393659,3.27544681369506));
#64381=CARTESIAN_POINT('',(43.,-11.3409760741447,2.03033536285951));
#64382=CARTESIAN_POINT('Origin',(43.,-10.7349660877716,1.38777878078145E-15));
#64383=CARTESIAN_POINT('',(43.,-11.50350615392,0.639801662020789));
#64384=CARTESIAN_POINT('',(43.,-11.50350615392,-0.639801662020786));
#64385=CARTESIAN_POINT('Origin',(43.,-10.4456036875545,-2.47565355172201));
#64386=CARTESIAN_POINT('',(43.,-11.3409760741447,-2.03033536285951));
#64387=CARTESIAN_POINT('',(43.,-11.0458792393659,-3.27544681369505));
#64388=CARTESIAN_POINT('Origin',(43.,-9.5931160887976,-4.81784397967164));
#64389=CARTESIAN_POINT('',(43.,-10.56705103871,-4.59101648279533));
#64390=CARTESIAN_POINT('',(43.,-9.99276611589833,-5.73451177982521));
#64391=CARTESIAN_POINT('Origin',(43.,-8.22346111860809,-6.90030319162475));
#64392=CARTESIAN_POINT('',(43.,-9.22345354659921,-6.90419471580332));
#64393=CARTESIAN_POINT('',(43.,-8.40094038459157,-7.88442773158195));
#64394=CARTESIAN_POINT('Origin',(43.,-6.41047723095084,-8.61076527244045));
#64395=CARTESIAN_POINT('',(43.,-7.3826172863893,-8.84516602459817));
#64396=CARTESIAN_POINT('',(43.,-6.35621778264911,-9.60929214352104));
#64397=CARTESIAN_POINT('Origin',(43.,-4.25190285648285,-9.85701876860538));
#64398=CARTESIAN_POINT('',(43.,-5.1437822173509,-10.309292143521));
#64399=CARTESIAN_POINT('',(43.,-3.96882983479838,-10.8161171287304));
#64400=CARTESIAN_POINT('Origin',(43.,-1.86410729845783,-10.5718778315606));
#64401=CARTESIAN_POINT('',(43.,-2.6276445175567,-11.2176416545259));
#64402=CARTESIAN_POINT('',(43.,-1.36748124326036,-11.4398424398823));
#64403=CARTESIAN_POINT('Origin',(43.,0.624182766533234,-10.7168042241878));
#64404=CARTESIAN_POINT('',(43.,0.0301501783194109,-11.5212452003569));
#64405=CARTESIAN_POINT('',(43.,1.30758861606115,-11.4468428840072));
#64406=CARTESIAN_POINT('Origin',(43.,3.07882297701681,-10.2839849271476));
#64407=CARTESIAN_POINT('',(43.,2.68631947027824,-11.2037354352735));
#64408=CARTESIAN_POINT('',(43.,3.91216603463411,-10.8367410653506));
#64409=CARTESIAN_POINT('Origin',(43.,5.36748304388578,-9.29675334077463));
#64410=CARTESIAN_POINT('',(43.,5.19766858426649,-10.2822293928957));
#64411=CARTESIAN_POINT('',(43.,6.30583756965351,-9.64242773087496));
#64412=CARTESIAN_POINT('Origin',(1.13921356237308,0.,0.));
#64413=CARTESIAN_POINT('',(0.7250000000004,-6.71403705763851,8.50428280207983));
#64414=CARTESIAN_POINT('Ctrl Pts',(0.724999999999708,-6.71335984205444,
8.50304879018103));
#64415=CARTESIAN_POINT('Ctrl Pts',(0.733026605239995,-6.92641633928169,
8.33946367811657));
#64416=CARTESIAN_POINT('Ctrl Pts',(0.740940929871476,-7.13307257448586,
8.16812285657541));
#64417=CARTESIAN_POINT('Ctrl Pts',(0.748756358915932,-7.33292193946551,
7.98945795695268));
#64418=CARTESIAN_POINT('Ctrl Pts',(0.756584638211413,-7.53309989990586,
7.81049929369949));
#64419=CARTESIAN_POINT('Ctrl Pts',(0.76431369644116,-7.72644915472315,7.62419206952429));
#64420=CARTESIAN_POINT('Ctrl Pts',(0.771956984759157,-7.91253600104634,
7.43092409212741));
#64421=CARTESIAN_POINT('Ctrl Pts',(0.779530442124436,-8.096922712398,7.23942185827309));
#64422=CARTESIAN_POINT('Ctrl Pts',(0.787019689648478,-8.27417961407399,
7.04108504419451));
#64423=CARTESIAN_POINT('Ctrl Pts',(0.79443781316425,-8.44385227796166,6.83625203349379));
#64424=CARTESIAN_POINT('Ctrl Pts',(0.800212214321066,-8.57592854017944,
6.67680632307532));
#64425=CARTESIAN_POINT('Ctrl Pts',(0.805943518977342,-8.70340868982644,
6.51342351738025));
#64426=CARTESIAN_POINT('Ctrl Pts',(0.811637899333878,-8.82606157077737,
6.34624917068448));
#64427=CARTESIAN_POINT('Ctrl Pts',(0.814239197455238,-8.88209167217916,
6.26988084142454));
#64428=CARTESIAN_POINT('Ctrl Pts',(0.816832790098731,-8.9371141781862,6.19272111954517));
#64429=CARTESIAN_POINT('Ctrl Pts',(0.819419265662117,-8.99111891717659,
6.11479294503839));
#64430=CARTESIAN_POINT('Ctrl Pts',(0.826604636584338,-9.14114704297707,
5.8983042037376));
#64431=CARTESIAN_POINT('Ctrl Pts',(0.833713812628948,-9.28289978709345,
5.67649524003392));
#64432=CARTESIAN_POINT('Ctrl Pts',(0.840755358224061,-9.41626049868725,
5.44992690374901));
#64433=CARTESIAN_POINT('Ctrl Pts',(0.84790890457536,-9.55174240659263,5.21975483804855));
#64434=CARTESIAN_POINT('Ctrl Pts',(0.8549926519471,-9.67856356222221,4.98467028977665));
#64435=CARTESIAN_POINT('Ctrl Pts',(0.862015579971874,-9.79656141681366,
4.74522601851525));
#64436=CARTESIAN_POINT('Ctrl Pts',(0.869056951950488,-9.91486916308786,
4.50515290710755));
#64437=CARTESIAN_POINT('Ctrl Pts',(0.876037184709222,-10.02430750059,4.26069654339065));
#64438=CARTESIAN_POINT('Ctrl Pts',(0.882965328814873,-10.1246675762525,
4.01238732779587));
#64439=CARTESIAN_POINT('Ctrl Pts',(0.88985287868436,-10.2244396097855,3.76553303617297));
#64440=CARTESIAN_POINT('Ctrl Pts',(0.89668894852099,-10.315239691526,3.51487029102214));
#64441=CARTESIAN_POINT('Ctrl Pts',(0.903482430731314,-10.3968142884726,
3.26090301038047));
#64442=CARTESIAN_POINT('Ctrl Pts',(0.904989246071567,-10.4149077860705,
3.2045722829942));
#64443=CARTESIAN_POINT('Ctrl Pts',(0.906493966244963,-10.4325472236707,
3.14807893692662));
#64444=CARTESIAN_POINT('Ctrl Pts',(0.907996688285087,-10.4497294915302,
3.09142840252523));
#64445=CARTESIAN_POINT('Ctrl Pts',(0.914798121173905,-10.5274977271745,
2.83502382632376));
#64446=CARTESIAN_POINT('Ctrl Pts',(0.92153920199599,-10.595686600671,2.57611633444297));
#64447=CARTESIAN_POINT('Ctrl Pts',(0.928226958834266,-10.6541321309661,
2.31524520296894));
#64448=CARTESIAN_POINT('Ctrl Pts',(0.934904048528506,-10.7124844391384,
2.05479016765412));
#64449=CARTESIAN_POINT('Ctrl Pts',(0.941527984209527,-10.7611247006838,
1.79237713010738));
#64450=CARTESIAN_POINT('Ctrl Pts',(0.948105760383946,-10.7998415598057,
1.5285239702178));
#64451=CARTESIAN_POINT('Ctrl Pts',(0.949439988481547,-10.8076948402946,
1.47500431703555));
#64452=CARTESIAN_POINT('Ctrl Pts',(0.950772317412216,-10.8151396711238,
1.42142536782279));
#64453=CARTESIAN_POINT('Ctrl Pts',(0.952102805548691,-10.8221740322919,
1.36779138536273));
#64454=CARTESIAN_POINT('Ctrl Pts',(0.958673983533257,-10.8569161979498,
1.10289729491273));
#64455=CARTESIAN_POINT('Ctrl Pts',(0.965200259104417,-10.8816499882616,
0.836661069242689));
#64456=CARTESIAN_POINT('Ctrl Pts',(0.971688664713417,-10.8964570290036,
0.569633878176683));
#64457=CARTESIAN_POINT('Ctrl Pts',(0.97707644134174,-10.9087523497421,0.347902539871251));
#64458=CARTESIAN_POINT('Ctrl Pts',(0.982438106095362,-10.9142020822907,
0.125625499710637));
#64459=CARTESIAN_POINT('Ctrl Pts',(0.987777685416798,-10.9128256696962,
-0.0968808233047792));
#64460=CARTESIAN_POINT('Ctrl Pts',(0.994189816422256,-10.9111727795822,
-0.364081590786523));
#64461=CARTESIAN_POINT('Ctrl Pts',(1.00055319720697,-10.8996813228307,-0.630917668696073));
#64462=CARTESIAN_POINT('Ctrl Pts',(1.00687375184277,-10.8784879568116,-0.896841028326388));
#64463=CARTESIAN_POINT('Ctrl Pts',(1.01321614470225,-10.8572213653409,-1.16368318292705));
#64464=CARTESIAN_POINT('Ctrl Pts',(1.01951541496329,-10.8261856600903,-1.42960695726622));
#64465=CARTESIAN_POINT('Ctrl Pts',(1.0257775483151,-10.7854663382832,-1.69406074261397));
#64466=CARTESIAN_POINT('Ctrl Pts',(1.03200494005034,-10.7449729227267,-1.95704736789066));
#64467=CARTESIAN_POINT('Ctrl Pts',(1.03819560579616,-10.6949029276176,-2.21858091129122));
#64468=CARTESIAN_POINT('Ctrl Pts',(1.04435543216967,-10.6352898291948,-2.47811128391209));
#64469=CARTESIAN_POINT('Ctrl Pts',(1.04850348743102,-10.5951460959847,-2.65288022419581));
#64470=CARTESIAN_POINT('Ctrl Pts',(1.05263755784743,-10.5506737759996,-2.8267406140342));
#64471=CARTESIAN_POINT('Ctrl Pts',(1.05675944102269,-10.5018704070006,-2.99952029639249));
#64472=CARTESIAN_POINT('Ctrl Pts',(1.0629007710959,-10.4291566533683,-3.25695045978844));
#64473=CARTESIAN_POINT('Ctrl Pts',(1.06900095568933,-10.3469954531024,-3.51139751252363));
#64474=CARTESIAN_POINT('Ctrl Pts',(1.07506533195419,-10.2554643254362,-3.76231651187138));
#64475=CARTESIAN_POINT('Ctrl Pts',(1.07674397561485,-10.2301281423731,-3.83177189676144));
#64476=CARTESIAN_POINT('Ctrl Pts',(1.07841987562493,-10.2040737300381,-3.90095690108396));
#64477=CARTESIAN_POINT('Ctrl Pts',(1.08009314517927,-10.1773020446965,-3.96985980070586));
#64478=CARTESIAN_POINT('Ctrl Pts',(1.08613676408953,-10.0806064086761,-4.21872757341254));
#64479=CARTESIAN_POINT('Ctrl Pts',(1.09214606726337,-9.97455728652671,-4.46391675270496));
#64480=CARTESIAN_POINT('Ctrl Pts',(1.09812638829685,-9.85950108128207,-4.70499072626318));
#64481=CARTESIAN_POINT('Ctrl Pts',(1.1027646420966,-9.77026508907132,-4.89196434651176));
#64482=CARTESIAN_POINT('Ctrl Pts',(1.10738546215988,-9.67560996452279,-5.07646226166185));
#64483=CARTESIAN_POINT('Ctrl Pts',(1.11199133682917,-9.57567838723778,-5.25827043391206));
#64484=CARTESIAN_POINT('Ctrl Pts',(1.11707662955477,-9.46534509345235,-5.45900272521038));
#64485=CARTESIAN_POINT('Ctrl Pts',(1.12213780964272,-9.34870474349792,-5.65622918144178));
#64486=CARTESIAN_POINT('Ctrl Pts',(1.127178060615,-9.2259690629308,-5.84967109060507));
#64487=CARTESIAN_POINT('Ctrl Pts',(1.13022993521894,-9.15165254405504,-5.96680026793372));
#64488=CARTESIAN_POINT('Ctrl Pts',(1.13327339817904,-9.07511873041999,-6.08251340265559));
#64489=CARTESIAN_POINT('Ctrl Pts',(1.136309144228,-8.99641356614057,-6.19674800058488));
#64490=CARTESIAN_POINT('Ctrl Pts',(1.1372781158142,-8.97129187722324,-6.23321023351521));
#64491=CARTESIAN_POINT('Ctrl Pts',(1.13824624770595,-8.94595032936056,-6.26951980831102));
#64492=CARTESIAN_POINT('Ctrl Pts',(1.13921356237309,-8.92039042199796,-6.30567469743334));
#64493=CARTESIAN_POINT('',(0.432106781186298,7.28849462691943,-7.74077132331895));
#64494=CARTESIAN_POINT('Ctrl Pts',(1.13921356237309,-10.477856724544,3.0906144932497));
#64495=CARTESIAN_POINT('Ctrl Pts',(1.13763308143963,-10.4574209463541,3.16000922715225));
#64496=CARTESIAN_POINT('Ctrl Pts',(1.13605477477627,-10.4362997195354,3.22920063924276));
#64497=CARTESIAN_POINT('Ctrl Pts',(1.13447854509856,-10.4144955096306,3.2981780152156));
#64498=CARTESIAN_POINT('Ctrl Pts',(1.13115766313255,-10.3685572758316,3.44350310785237));
#64499=CARTESIAN_POINT('Ctrl Pts',(1.12784665698753,-10.3195968367299,3.58784946507828));
#64500=CARTESIAN_POINT('Ctrl Pts',(1.12454462644006,-10.2676369503773,3.73111680051442));
#64501=CARTESIAN_POINT('Ctrl Pts',(1.11947030835345,-10.1877888122978,3.95127952189849));
#64502=CARTESIAN_POINT('Ctrl Pts',(1.11441935125481,-10.1008929441298,4.16880046250299));
#64503=CARTESIAN_POINT('Ctrl Pts',(1.10938854200519,-10.0070260356517,4.38331364872119));
#64504=CARTESIAN_POINT('Ctrl Pts',(1.10363613599139,-9.89969527790813,4.62859564635048));
#64505=CARTESIAN_POINT('Ctrl Pts',(1.09791905327103,-9.78342381018177,4.86955193565516));
#64506=CARTESIAN_POINT('Ctrl Pts',(1.09223274962076,-9.65836681837275,5.10565687499648));
#64507=CARTESIAN_POINT('Ctrl Pts',(1.09152947110833,-9.64289984710673,5.13485818761189));
#64508=CARTESIAN_POINT('Ctrl Pts',(1.09082666341069,-9.62729842486737,5.16398527146063));
#64509=CARTESIAN_POINT('Ctrl Pts',(1.09012431793074,-9.61156279278248,5.19303711398957));
#64510=CARTESIAN_POINT('Ctrl Pts',(1.08447046953009,-9.48489168741206,5.42690309321017));
#64511=CARTESIAN_POINT('Ctrl Pts',(1.07884657364517,-9.34952739565971,5.65589529942071));
#64512=CARTESIAN_POINT('Ctrl Pts',(1.07324814559379,-9.20588053275856,5.87964084721218));
#64513=CARTESIAN_POINT('Ctrl Pts',(1.06762104052026,-9.06149786255003,6.10453249458239));
#64514=CARTESIAN_POINT('Ctrl Pts',(1.06201966485802,-8.90874714934212,6.3241241042676));
#64515=CARTESIAN_POINT('Ctrl Pts',(1.05643946465514,-8.74800159464796,6.53800797753036));
#64516=CARTESIAN_POINT('Ctrl Pts',(1.0521954119542,-8.62574565744833,6.70067856227765));
#64517=CARTESIAN_POINT('Ctrl Pts',(1.04796360808913,-8.49886420561854,6.8600470011273));
#64518=CARTESIAN_POINT('Ctrl Pts',(1.04374204959655,-8.36750680337259,7.01592000534807));
#64519=CARTESIAN_POINT('Ctrl Pts',(1.03814630520578,-8.193390431872,7.22253220569441));
#64520=CARTESIAN_POINT('Ctrl Pts',(1.03258405359143,-8.01189492603689,7.42243050187484));
#64521=CARTESIAN_POINT('Ctrl Pts',(1.02705096687246,-7.82345724472851,7.61524123425328));
#64522=CARTESIAN_POINT('Ctrl Pts',(1.02156306555032,-7.63655842081408,7.80647739715551));
#64523=CARTESIAN_POINT('Ctrl Pts',(1.01610385472419,-7.44282982232682,7.99074172287405));
#64524=CARTESIAN_POINT('Ctrl Pts',(1.01066911167913,-7.24265586910669,8.16763781415122));
#64525=CARTESIAN_POINT('Ctrl Pts',(1.00516724706788,-7.04000967586757,8.34671865318915));
#64526=CARTESIAN_POINT('Ctrl Pts',(0.999690458346456,-6.83075754475374,
8.5182487185602));
#64527=CARTESIAN_POINT('Ctrl Pts',(0.994234364402248,-6.6152618682679,8.68177610532039));
#64528=CARTESIAN_POINT('Ctrl Pts',(0.98877827045804,-6.39976619178206,8.84530349208058));
#64529=CARTESIAN_POINT('Ctrl Pts',(0.983342871291044,-6.1780264993059,9.00082872467117));
#64530=CARTESIAN_POINT('Ctrl Pts',(0.977923785788639,-5.95037558631415,
9.1478512585176));
#64531=CARTESIAN_POINT('Ctrl Pts',(0.976644345775613,-5.89662746092396,
9.18256311396554));
#64532=CARTESIAN_POINT('Ctrl Pts',(0.975365815129984,-5.84254971516498,
9.21680077163412));
#64533=CARTESIAN_POINT('Ctrl Pts',(0.974088136192873,-5.78814923193305,
9.25056134875322));
#64534=CARTESIAN_POINT('Ctrl Pts',(0.968846505885174,-5.56497327326318,
9.38906286043428));
#64535=CARTESIAN_POINT('Ctrl Pts',(0.963635363001742,-5.33705940815049,
9.51910941319204));
#64536=CARTESIAN_POINT('Ctrl Pts',(0.958451011843141,-5.10495653633402,
9.64062895798397));
#64537=CARTESIAN_POINT('Ctrl Pts',(0.953028039799334,-4.86217063186076,
9.76774170054761));
#64538=CARTESIAN_POINT('Ctrl Pts',(0.947634382531812,-4.61480081436479,
9.88552498020093));
#64539=CARTESIAN_POINT('Ctrl Pts',(0.942265810185289,-4.36343962414311,
9.99384860346975));
#64540=CARTESIAN_POINT('Ctrl Pts',(0.937030389108632,-4.11831269128308,
10.0994855854746));
#64541=CARTESIAN_POINT('Ctrl Pts',(0.931818824071832,-3.86938916470361,
10.1961263377675));
#64542=CARTESIAN_POINT('Ctrl Pts',(0.926627192204765,-3.61719481498128,
10.2836023735669));
#64543=CARTESIAN_POINT('Ctrl Pts',(0.921237503954366,-3.3553794632154,10.3744155464597));
#64544=CARTESIAN_POINT('Ctrl Pts',(0.915869298750878,-3.09003835480785,
10.4553520081255));
#64545=CARTESIAN_POINT('Ctrl Pts',(0.910518187416254,-2.82174391269712,
10.5261658536988));
#64546=CARTESIAN_POINT('Ctrl Pts',(0.905444075780115,-2.56733770331453,
10.5933140282281));
#64547=CARTESIAN_POINT('Ctrl Pts',(0.900385334093099,-2.3102753383835,10.6513602100867));
#64548=CARTESIAN_POINT('Ctrl Pts',(0.895338220118187,-2.05104059707808,
10.7000429643343));
#64549=CARTESIAN_POINT('Ctrl Pts',(0.895062694243016,-2.0368887710389,10.7027005937313));
#64550=CARTESIAN_POINT('Ctrl Pts',(0.894787203020205,-2.02273047128043,
10.7053303057181));
#64551=CARTESIAN_POINT('Ctrl Pts',(0.894511745840935,-2.00856577669844,
10.7079320532379));
#64552=CARTESIAN_POINT('Ctrl Pts',(0.889401001454546,-1.74575856466006,
10.7562040444293));
#64553=CARTESIAN_POINT('Ctrl Pts',(0.884319779851196,-1.48166721548634,
10.794685434552));
#64554=CARTESIAN_POINT('Ctrl Pts',(0.879264451582565,-1.21682005225955,
10.8232520779441));
#64555=CARTESIAN_POINT('Ctrl Pts',(0.876921807049914,-1.09408959323652,
10.8364898910796));
#64556=CARTESIAN_POINT('Ctrl Pts',(0.874584722866263,-0.971196558317258,
10.8475979230759));
#64557=CARTESIAN_POINT('Ctrl Pts',(0.872252837861574,-0.848192386456712,
10.8565602006629));
#64558=CARTESIAN_POINT('Ctrl Pts',(0.867237085977621,-0.583617415777176,
10.8758375495036));
#64559=CARTESIAN_POINT('Ctrl Pts',(0.86224538838669,-0.318528561533122,
10.8851909660222));
#64560=CARTESIAN_POINT('Ctrl Pts',(0.85727415092005,-0.0534592325833127,
10.8847756706377));
#64561=CARTESIAN_POINT('Ctrl Pts',(0.85228141719438,0.21275628964214,10.8843585794634));
#64562=CARTESIAN_POINT('Ctrl Pts',(0.847309320919891,0.478952760788212,
10.8740880302371));
#64563=CARTESIAN_POINT('Ctrl Pts',(0.842354221101031,0.744590121269635,
10.8540684382892));
#64564=CARTESIAN_POINT('Ctrl Pts',(0.837420856891087,1.00906226006193,10.8341366625381));
#64565=CARTESIAN_POINT('Ctrl Pts',(0.832504340353467,1.2729808153636,10.8045410407433));
#64566=CARTESIAN_POINT('Ctrl Pts',(0.827601078196573,1.53580354714305,10.7653341716951));
#64567=CARTESIAN_POINT('Ctrl Pts',(0.823621521761986,1.74911416769346,10.7335133261012));
#64568=CARTESIAN_POINT('Ctrl Pts',(0.81965069621806,1.96170292216141,10.6953604214243));
#64569=CARTESIAN_POINT('Ctrl Pts',(0.815686680503933,2.17327106150822,10.6508799021689));
#64570=CARTESIAN_POINT('Ctrl Pts',(0.810804169986808,2.43386126597384,10.5960928834653));
#64571=CARTESIAN_POINT('Ctrl Pts',(0.805949363128693,2.69197493778206,10.531902823093));
#64572=CARTESIAN_POINT('Ctrl Pts',(0.801118889370196,2.94708953327321,10.4584732715955));
#64573=CARTESIAN_POINT('Ctrl Pts',(0.796282165955273,3.2025341954723,10.3849487171042));
#64574=CARTESIAN_POINT('Ctrl Pts',(0.791469838644924,3.45497265704967,10.3021606204436));
#64575=CARTESIAN_POINT('Ctrl Pts',(0.786678523780355,3.70387439973033,10.2102214489231));
#64576=CARTESIAN_POINT('Ctrl Pts',(0.781920863008356,3.95102786192312,10.1189280561661));
#64577=CARTESIAN_POINT('Ctrl Pts',(0.777183920536879,4.19469471906823,10.018611509716));
#64578=CARTESIAN_POINT('Ctrl Pts',(0.772464383507734,4.43434042015135,9.90933337288456));
#64579=CARTESIAN_POINT('Ctrl Pts',(0.767708844717327,4.67581419616309,9.79922163619598));
#64580=CARTESIAN_POINT('Ctrl Pts',(0.762970977927859,4.91320579000226,9.68001076338069));
#64581=CARTESIAN_POINT('Ctrl Pts',(0.75824739388751,5.1460893524394,9.55204235649902));
#64582=CARTESIAN_POINT('Ctrl Pts',(0.753532396346061,5.37854958072274,9.42430656971588));
#64583=CARTESIAN_POINT('Ctrl Pts',(0.748831629674759,5.60651865825446,9.28784464607474));
#64584=CARTESIAN_POINT('Ctrl Pts',(0.744141723071082,5.82954096950498,9.1429558285772));
#64585=CARTESIAN_POINT('Ctrl Pts',(0.74259451225051,5.90311653557811,9.09515667922181));
#64586=CARTESIAN_POINT('Ctrl Pts',(0.741048483390892,5.97615342524599,9.04644008343829));
#64587=CARTESIAN_POINT('Ctrl Pts',(0.739503515463292,6.04863436578528,8.99681593334812));
#64588=CARTESIAN_POINT('Ctrl Pts',(0.734863767385957,6.26630445362522,8.84778788502619));
#64589=CARTESIAN_POINT('Ctrl Pts',(0.730250109530775,6.47818691206417,8.69110907842344));
#64590=CARTESIAN_POINT('Ctrl Pts',(0.725659455047584,6.68391467027405,8.52718411802919));
#64591=CARTESIAN_POINT('Ctrl Pts',(0.721023486450231,6.89167315659813,8.36164106278674));
#64592=CARTESIAN_POINT('Ctrl Pts',(0.716410977596418,7.09315537397336,8.18870774038521));
#64593=CARTESIAN_POINT('Ctrl Pts',(0.711818749320292,7.28795751414488,8.00875466870083));
#64594=CARTESIAN_POINT('Ctrl Pts',(0.707233935345279,7.48244513995915,7.82909213707225));
#64595=CARTESIAN_POINT('Ctrl Pts',(0.702669336513519,7.67027473342892,7.64243207354529));
#64596=CARTESIAN_POINT('Ctrl Pts',(0.698121789032906,7.8510112305555,7.44910343525155));
#64597=CARTESIAN_POINT('Ctrl Pts',(0.693627981702904,8.02961189367095,7.25805943723556));
#64598=CARTESIAN_POINT('Ctrl Pts',(0.689150825100288,8.20128652139586,7.06050308523023));
#64599=CARTESIAN_POINT('Ctrl Pts',(0.684687266276008,8.3655762529813,6.85671964793019));
#64600=CARTESIAN_POINT('Ctrl Pts',(0.682517979460545,8.44542096046125,6.75768102400976));
#64601=CARTESIAN_POINT('Ctrl Pts',(0.680351904377722,8.52352076099609,6.65717114719464));
#64602=CARTESIAN_POINT('Ctrl Pts',(0.678188690577029,8.59981914949716,6.55522045519679));
#64603=CARTESIAN_POINT('Ctrl Pts',(0.674235981436656,8.73923455888814,6.36893215026916));
#64604=CARTESIAN_POINT('Ctrl Pts',(0.670292825554322,8.87263707984504,6.17783375356159));
#64605=CARTESIAN_POINT('Ctrl Pts',(0.666357084904245,8.99985180806314,5.98224795015969));
#64606=CARTESIAN_POINT('Ctrl Pts',(0.661946851434784,9.14240354154305,5.76308232594674));
#64607=CARTESIAN_POINT('Ctrl Pts',(0.65756160146588,9.27667903776863,5.53906302224739));
#64608=CARTESIAN_POINT('Ctrl Pts',(0.653198503486205,9.40256457256295,5.31072696629792));
#64609=CARTESIAN_POINT('Ctrl Pts',(0.648785999809938,9.52987557672935,5.07980533882245));
#64610=CARTESIAN_POINT('Ctrl Pts',(0.644396152640973,9.64860583657575,4.84446810109741));
#64611=CARTESIAN_POINT('Ctrl Pts',(0.640026033186523,9.75859577899607,4.60523793181333));
#64612=CARTESIAN_POINT('Ctrl Pts',(0.635637277637013,9.86905476649487,4.36498758076484));
#64613=CARTESIAN_POINT('Ctrl Pts',(0.63126841841593,9.97069900244601,4.12081043065888));
#64614=CARTESIAN_POINT('Ctrl Pts',(0.626916489101524,10.0633205597902,3.8732117373834));
#64615=CARTESIAN_POINT('Ctrl Pts',(0.622585543652824,10.155495520193,3.62680690029298));
#64616=CARTESIAN_POINT('Ctrl Pts',(0.618271365241239,10.2387348064874,3.37701282505353));
#64617=CARTESIAN_POINT('Ctrl Pts',(0.613971030148381,10.3127842830142,3.1243127112796));
#64618=CARTESIAN_POINT('Ctrl Pts',(0.609736671809157,10.385697675035,2.8754895821568));
#64619=CARTESIAN_POINT('Ctrl Pts',(0.605515735272247,10.4497011890361,2.62384832323812));
#64620=CARTESIAN_POINT('Ctrl Pts',(0.601305429334362,10.5045021989228,2.36984467960267));
#64621=CARTESIAN_POINT('Ctrl Pts',(0.599660718535591,10.525909624909,2.27062088404535));
#64622=CARTESIAN_POINT('Ctrl Pts',(0.59801762995594,10.5459122037102,2.17103657634585));
#64623=CARTESIAN_POINT('Ctrl Pts',(0.596375997208508,10.5644903125394,2.07111897731654));
#64624=CARTESIAN_POINT('Ctrl Pts',(0.59399579910307,10.5914266535127,1.92624876789767));
#64625=CARTESIAN_POINT('Ctrl Pts',(0.591623455770162,10.6153143629136,1.78097002630818));
#64626=CARTESIAN_POINT('Ctrl Pts',(0.58925849196569,10.6361258834378,1.6353707827831));
#64627=CARTESIAN_POINT('Ctrl Pts',(0.585077565471064,10.6729177520442,1.37797160665187));
#64628=CARTESIAN_POINT('Ctrl Pts',(0.58091970244798,10.7000985484984,1.11957140021379));
#64629=CARTESIAN_POINT('Ctrl Pts',(0.576782277101345,10.717814348248,0.860696065758531));
#64630=CARTESIAN_POINT('Ctrl Pts',(0.572582995972931,10.735795004654,0.597950465412193));
#64631=CARTESIAN_POINT('Ctrl Pts',(0.568404768188129,10.7440255795964,0.334714802351492));
#64632=CARTESIAN_POINT('Ctrl Pts',(0.564244848413053,10.7426058460084,0.0715303853695533));
#64633=CARTESIAN_POINT('Ctrl Pts',(0.560079949701344,10.7411844131656,-0.19196903252724));
#64634=CARTESIAN_POINT('Ctrl Pts',(0.555933402850673,10.7300894871931,-0.455417737004014));
#64635=CARTESIAN_POINT('Ctrl Pts',(0.551802452657825,10.7093689218361,-0.718271289950675));
#64636=CARTESIAN_POINT('Ctrl Pts',(0.547709928256149,10.6888410976355,-0.978679798715508));
#64637=CARTESIAN_POINT('Ctrl Pts',(0.54363271170391,10.6588657301226,-1.2385047963445));
#64638=CARTESIAN_POINT('Ctrl Pts',(0.539568123971003,10.6194398119681,-1.49720624911382));
#64639=CARTESIAN_POINT('Ctrl Pts',(0.536254598413142,10.5872990892106,-1.70810436029658));
#64640=CARTESIAN_POINT('Ctrl Pts',(0.532949465723335,10.5488767859629,-1.91825573707104));
#64641=CARTESIAN_POINT('Ctrl Pts',(0.529651274461671,10.5041474612957,-2.12735818519859));
#64642=CARTESIAN_POINT('Ctrl Pts',(0.525586067873786,10.4490160480808,-2.38508873574351));
#64643=CARTESIAN_POINT('Ctrl Pts',(0.521546127062304,10.3845045620134,-2.64029043501042));
#64644=CARTESIAN_POINT('Ctrl Pts',(0.517528930083677,10.310723224817,-2.89243634239262));
#64645=CARTESIAN_POINT('Ctrl Pts',(0.513559586306218,10.2378207773514,-3.14157866571008));
#64646=CARTESIAN_POINT('Ctrl Pts',(0.509612447735869,10.1558678136205,-3.38773817416334));
#64647=CARTESIAN_POINT('Ctrl Pts',(0.505685081484604,10.0649211552357,-3.63039966339775));
#64648=CARTESIAN_POINT('Ctrl Pts',(0.501716199920375,9.97301312000337,-3.87562627312913));
#64649=CARTESIAN_POINT('Ctrl Pts',(0.497767510902168,9.87192019985151,-4.11728116306982));
#64650=CARTESIAN_POINT('Ctrl Pts',(0.493836503570971,9.76198307580139,-4.35493572935158));
#64651=CARTESIAN_POINT('Ctrl Pts',(0.489895930395532,9.65177842708991,-4.59316861217486));
#64652=CARTESIAN_POINT('Ctrl Pts',(0.48597312506622,9.53268611470959,-4.82738222749505));
#64653=CARTESIAN_POINT('Ctrl Pts',(0.482065558349359,9.40500349653363,-5.05711947107752));
#64654=CARTESIAN_POINT('Ctrl Pts',(0.478182290677156,9.27811486752434,-5.28542810295709));
#64655=CARTESIAN_POINT('Ctrl Pts',(0.474314072685286,9.14274202900883,-5.50931636425508));
#64656=CARTESIAN_POINT('Ctrl Pts',(0.47045842203108,8.99913749852263,-5.72830281597816));
#64657=CARTESIAN_POINT('Ctrl Pts',(0.46907137261899,8.94747654750597,-5.80708200433299));
#64658=CARTESIAN_POINT('Ctrl Pts',(0.467685949623486,8.89474994107878,-5.88522647316663));
#64659=CARTESIAN_POINT('Ctrl Pts',(0.466302037474734,8.84096833393254,-5.96271256723553));
#64660=CARTESIAN_POINT('Ctrl Pts',(0.462459974638316,8.69165805127795,-6.1778320331854));
#64661=CARTESIAN_POINT('Ctrl Pts',(0.458643579556667,8.53476065639516,-6.38709923307584));
#64662=CARTESIAN_POINT('Ctrl Pts',(0.454850535787384,8.3706405761198,-6.59011266902282));
#64663=CARTESIAN_POINT('Ctrl Pts',(0.451015356700307,8.20469735533795,-6.79538129530248));
#64664=CARTESIAN_POINT('Ctrl Pts',(0.447204050606851,8.03136976050665,-6.99425703384597));
#64665=CARTESIAN_POINT('Ctrl Pts',(0.443414223006749,7.8509882461713,-7.18629733565622));
#64666=CARTESIAN_POINT('Ctrl Pts',(0.439624395406647,7.67060673183595,-7.37833763746647));
#64667=CARTESIAN_POINT('Ctrl Pts',(0.4358560462999,7.48317089012288,-7.56354305099811));
#64668=CARTESIAN_POINT('Ctrl Pts',(0.432106781186244,7.28897086323717,-7.74143516723144));
#64669=CARTESIAN_POINT('',(0.43210678118657,-6.57359493970369,8.35640737250497));
#64670=CARTESIAN_POINT('Origin',(0.432106781186538,-5.29372197986008E-16,
0.));
#64671=CARTESIAN_POINT('Ctrl Pts',(0.432106087019021,-6.57359491695503,
8.3564057487116));
#64672=CARTESIAN_POINT('Ctrl Pts',(0.432499680727653,-6.57386187415739,
8.35669653072526));
#64673=CARTESIAN_POINT('Ctrl Pts',(0.432893603877904,-6.57412862767405,
8.35698705347474));
#64674=CARTESIAN_POINT('Ctrl Pts',(0.43328785602668,-6.57439517729756,8.35727731668458));
#64675=CARTESIAN_POINT('Ctrl Pts',(0.464650193048242,-6.59559891493411,
8.38036744476688));
#64676=CARTESIAN_POINT('Ctrl Pts',(0.498045118005864,-6.6154829834037,8.40178361965518));
#64677=CARTESIAN_POINT('Ctrl Pts',(0.533242338208013,-6.63392272005744,
8.42139302969376));
#64678=CARTESIAN_POINT('Ctrl Pts',(0.545197310570806,-6.64018590052473,
8.42805349758626));
#64679=CARTESIAN_POINT('Ctrl Pts',(0.55736051028647,-6.64628225417658,8.43450526928213));
#64680=CARTESIAN_POINT('Ctrl Pts',(0.569723755782689,-6.65220622141807,
8.44074229613904));
#64681=CARTESIAN_POINT('Ctrl Pts',(0.606101769892647,-6.66963709456251,
8.45909432603881));
#64682=CARTESIAN_POINT('Ctrl Pts',(0.644102912062366,-6.68552633914734,
8.47553577160341));
#64683=CARTESIAN_POINT('Ctrl Pts',(0.683468556086442,-6.69977718424115,
8.4899682337961));
#64684=CARTESIAN_POINT('Ctrl Pts',(0.697150677552244,-6.70473027972321,
8.49498445303159));
#64685=CARTESIAN_POINT('Ctrl Pts',(0.710997883259307,-6.70948520674752,
8.4997576858588));
#64686=CARTESIAN_POINT('Ctrl Pts',(0.724999999999994,-6.71403705768202,
8.50428280204387));
#64687=CARTESIAN_POINT('Ctrl Pts',(0.230187047118035,-4.37735375204676,
9.06716418619638));
#64688=CARTESIAN_POINT('Ctrl Pts',(0.269788725778111,-5.88144327003121,
8.34103507242267));
#64689=CARTESIAN_POINT('Ctrl Pts',(0.348992083098263,-8.5198365510072,6.12665932563764));
#64690=CARTESIAN_POINT('Ctrl Pts',(0.467797119078491,-10.4108209426255,
1.31555314620701));
#64691=CARTESIAN_POINT('Ctrl Pts',(0.586602155058718,-9.77617122600883,
-3.8132732942528));
#64692=CARTESIAN_POINT('Ctrl Pts',(0.705407191038946,-6.77002375276244,
-8.01775424432509));
#64693=CARTESIAN_POINT('Ctrl Pts',(0.824212227019173,-2.12153173002185,
-10.2768823633875));
#64694=CARTESIAN_POINT('Ctrl Pts',(0.943017262999401,3.04159683638712,-10.0431701202702));
#64695=CARTESIAN_POINT('Ctrl Pts',(1.06182229897963,7.46688591750615,-7.37303115014316));
#64696=CARTESIAN_POINT('Ctrl Pts',(1.18062733495986,10.0808097748896,-2.91434903386085));
#64697=CARTESIAN_POINT('Ctrl Pts',(1.29943237094008,10.249274439043,2.25133856122268));
#64698=CARTESIAN_POINT('Ctrl Pts',(1.41823740692031,7.93140919765733,6.87087002708225));
#64699=CARTESIAN_POINT('Ctrl Pts',(1.53704244290054,3.68949714972476,9.82363271220668));
#64700=CARTESIAN_POINT('Ctrl Pts',(1.65584747888077,-1.44743493143616,10.3933177948697));
#64701=CARTESIAN_POINT('Ctrl Pts',(1.774652514861,-6.23323964791348,8.44173315899732));
#64702=CARTESIAN_POINT('Ctrl Pts',(1.89345755084122,-9.50694887448361,4.44230277254114));
#64703=CARTESIAN_POINT('Ctrl Pts',(2.01226258682145,-10.4744070276475,-0.634766799185825));
#64704=CARTESIAN_POINT('Ctrl Pts',(2.13106762280168,-8.90092254260253,-5.55785119946268));
#64705=CARTESIAN_POINT('Ctrl Pts',(2.2498726587819,-5.16820041446581,-9.13267955350996));
#64706=CARTESIAN_POINT('Ctrl Pts',(2.36867769476214,-0.181746135518434,
-10.4920493795623));
#64707=CARTESIAN_POINT('Ctrl Pts',(2.48748273074236,4.84879718275033,-9.30619672407481));
#64708=CARTESIAN_POINT('Ctrl Pts',(2.60628776672259,8.70309103847143,-5.86279268462035));
#64709=CARTESIAN_POINT('Ctrl Pts',(2.72509280270281,10.4461383825637,-0.997158240267306));
#64710=CARTESIAN_POINT('Ctrl Pts',(2.84389783868305,9.65510063715378,4.11037265272831));
#64711=CARTESIAN_POINT('Ctrl Pts',(2.96270287466327,6.52187234635328,8.22078541060934));
#64712=CARTESIAN_POINT('Ctrl Pts',(3.0815079106435,1.80653027708299,10.3369521629193));
#64713=CARTESIAN_POINT('Ctrl Pts',(3.20031294662373,-3.3470504283007,9.94552085593946));
#64714=CARTESIAN_POINT('Ctrl Pts',(3.31911798260395,-7.68868414698893,7.14144717485069));
#64715=CARTESIAN_POINT('Ctrl Pts',(3.43792301858418,-10.1651520849887,2.60495964518155));
#64716=CARTESIAN_POINT('Ctrl Pts',(3.55672805456441,-10.1756982265257,-2.56345416706898));
#64717=CARTESIAN_POINT('Ctrl Pts',(3.67553309054464,-7.71776422714997,-7.11001033739966));
#64718=CARTESIAN_POINT('Ctrl Pts',(3.79433812652486,-3.38761003189172,-9.93177879011561));
#64719=CARTESIAN_POINT('Ctrl Pts',(3.9131431625051,1.76433033496111,-10.3442384994258));
#64720=CARTESIAN_POINT('Ctrl Pts',(4.03194819848532,6.48826917337762,-8.24733258682529));
#64721=CARTESIAN_POINT('Ctrl Pts',(4.15075323446555,9.63824588685654,-4.14974070134389));
#64722=CARTESIAN_POINT('Ctrl Pts',(4.26955827044577,10.4501207782042,0.954519452312438));
#64723=CARTESIAN_POINT('Ctrl Pts',(4.38836330642601,8.72694450777083,5.82722671793283));
#64724=CARTESIAN_POINT('Ctrl Pts',(4.50716834240623,4.88673521132993,9.28633138748812));
#64725=CARTESIAN_POINT('Ctrl Pts',(4.62597337838646,-0.138926773910176,
10.4927037037835));
#64726=CARTESIAN_POINT('Ctrl Pts',(4.74477841436669,-5.13088709320036,9.15369484419977));
#64727=CARTESIAN_POINT('Ctrl Pts',(4.86358345034691,-8.87816693820219,5.59412937652621));
#64728=CARTESIAN_POINT('Ctrl Pts',(4.98238848632714,-10.4717293392756,0.677507423467737));
#64729=CARTESIAN_POINT('Ctrl Pts',(5.10119352230737,-9.52499864797096,-4.403468226302));
#64730=CARTESIAN_POINT('Ctrl Pts',(5.21999855828759,-6.26763830931662,-8.41622490713541));
#64731=CARTESIAN_POINT('Ctrl Pts',(5.33880359426783,-1.48983776572259,-10.387324732371));
#64732=CARTESIAN_POINT('Ctrl Pts',(5.45760863024804,3.64937630016661,-9.83860682635921));
#64733=CARTESIAN_POINT('Ctrl Pts',(5.57641366622829,7.90330340852995,-6.90318237457325));
#64734=CARTESIAN_POINT('Ctrl Pts',(5.6952187022085,10.2400011457753,-2.29314373697339));
#64735=CARTESIAN_POINT('Ctrl Pts',(5.81402373818874,10.092619765449,2.87317906402775));
#64736=CARTESIAN_POINT('Ctrl Pts',(5.93282877416896,7.49691190116663,7.34250935375952));
#64737=CARTESIAN_POINT('Ctrl Pts',(6.05163381014919,3.08255948452053,10.0306509603461));
#64738=CARTESIAN_POINT('Ctrl Pts',(6.17043884612943,-2.07957816526778,10.285498836636));
#64739=CARTESIAN_POINT('Ctrl Pts',(6.28924388210963,-6.73723963188388,8.0452305005185));
#64740=CARTESIAN_POINT('Ctrl Pts',(6.40804891808988,-9.76054226968837,3.85330329269919));
#64741=CARTESIAN_POINT('Ctrl Pts',(6.52685395407009,-10.4160757165381,-1.27338067020242));
#64742=CARTESIAN_POINT('Ctrl Pts',(6.64565899005034,-8.54481685095021,-6.09116053372568));
#64743=CARTESIAN_POINT('Ctrl Pts',(6.76446402603055,-4.60070654709105,-9.43131119895073));
#64744=CARTESIAN_POINT('Ctrl Pts',(6.88326906201079,0.459469946313315,-10.4835594638622));
#64745=CARTESIAN_POINT('Ctrl Pts',(7.00207409799101,5.40818554410445,-8.99264481587256));
#64746=CARTESIAN_POINT('Ctrl Pts',(7.12087913397124,9.04495199435029,-5.32024201364924));
#64747=CARTESIAN_POINT('Ctrl Pts',(7.23968416995146,10.4875413103608,-0.357223917697587));
#64748=CARTESIAN_POINT('Ctrl Pts',(7.3584892059317,9.38600177395559,4.69245163674624));
#64749=CARTESIAN_POINT('Ctrl Pts',(7.47729424191192,6.00755126144244,8.6038049434562));
#64750=CARTESIAN_POINT('Ctrl Pts',(7.59609927789215,1.17175397485717,10.4279971368574));
#64751=CARTESIAN_POINT('Ctrl Pts',(7.71490431387238,-3.94829421545725,9.72250505024742));
#64752=CARTESIAN_POINT('Ctrl Pts',(7.83370934985261,-8.11054219940231,6.65847106291035));
#64753=CARTESIAN_POINT('Ctrl Pts',(7.95251438583283,-10.3052876193431,1.97918638498572));
#64754=CARTESIAN_POINT('Ctrl Pts',(8.07131942181306,-10.000116348714,-3.18022085335027));
#64755=CARTESIAN_POINT('Ctrl Pts',(8.19012445779329,-7.26905861171694,-7.56815159489579));
#64756=CARTESIAN_POINT('Ctrl Pts',(8.30892949377352,-2.77463030036995,-10.1201560442598));
#64757=CARTESIAN_POINT('Ctrl Pts',(8.42773452975374,2.39288398919242,-10.2171540987775));
#64758=CARTESIAN_POINT('Ctrl Pts',(8.54653956573398,6.97991854406481,-7.83561540544965));
#64759=CARTESIAN_POINT('Ctrl Pts',(8.66534460171419,9.87372380620264,-3.55326749101827));
#64760=CARTESIAN_POINT('Ctrl Pts',(8.78414963769443,10.3723036410682,1.59105274626059));
#64761=CARTESIAN_POINT('Ctrl Pts',(8.90295467367466,8.35470964850016,6.34940614177092));
#64762=CARTESIAN_POINT('Ctrl Pts',(9.02175970965488,4.31038153005013,9.56748361531403));
#64763=CARTESIAN_POINT('Ctrl Pts',(9.14056474563511,-0.779584044405554,
10.4646251906893));
#64764=CARTESIAN_POINT('Ctrl Pts',(9.25936978161534,-5.68043358093007,8.82319703942633));
#64765=CARTESIAN_POINT('Ctrl Pts',(9.37817481759556,-9.20329045551407,5.0413863624348));
#64766=CARTESIAN_POINT('Ctrl Pts',(9.4969798535758,-10.4935595297617,0.036606819692515));
#64767=CARTESIAN_POINT('Ctrl Pts',(9.61578488955601,-9.23823981688005,-4.97705301857555));
#64768=CARTESIAN_POINT('Ctrl Pts',(9.73458992553625,-5.7418540840304,-8.78335034833538));
#64769=CARTESIAN_POINT('Ctrl Pts',(9.85339496151647,-0.85257594587396,-10.4589313947658));
#64770=CARTESIAN_POINT('Ctrl Pts',(9.97219999749669,4.24352503079001,-9.5973239487348));
#64771=CARTESIAN_POINT('Ctrl Pts',(10.0910050334769,8.31020699042318,-6.40754176265919));
#64772=CARTESIAN_POINT('Ctrl Pts',(10.2098100694571,10.3609505381623,-1.66338077710884));
#64773=CARTESIAN_POINT('Ctrl Pts',(10.3286151054374,9.89827436029318,3.48429280518479));
#64774=CARTESIAN_POINT('Ctrl Pts',(10.4474201414176,7.03441713875368,7.78672634564157));
#64775=CARTESIAN_POINT('Ctrl Pts',(10.5662251773978,2.46411003797023,10.2002104578618));
#64776=CARTESIAN_POINT('Ctrl Pts',(10.6850302133781,-2.70395522724915,10.1392681093327));
#64777=CARTESIAN_POINT('Ctrl Pts',(10.8038352493583,-7.21607928511531,7.61868304989973));
#64778=CARTESIAN_POINT('Ctrl Pts',(10.9226402853385,-9.97768480223973,3.24991348362604));
#64779=CARTESIAN_POINT('Ctrl Pts',(11.0414453213188,-10.3188454281855,-1.90723902359301));
#64780=CARTESIAN_POINT('Ctrl Pts',(11.160250357299,-8.15680043132904,-6.60172238036183));
#64781=CARTESIAN_POINT('Ctrl Pts',(11.2790553932792,-4.01603127915127,-9.69472147247038));
#64782=CARTESIAN_POINT('Ctrl Pts',(11.3978604292594,1.09897013081975,-10.4359185659656));
#64783=CARTESIAN_POINT('Ctrl Pts',(11.5166654652397,5.94737696585456,-8.64550975304073));
#64784=CARTESIAN_POINT('Ctrl Pts',(11.6354705012199,9.35303445790701,-4.75782283120169));
#64785=CARTESIAN_POINT('Ctrl Pts',(11.7542755372001,10.4897783773862,0.284044463455958));
#64786=CARTESIAN_POINT('Ctrl Pts',(11.8730805731804,9.08185076370161,5.25700659784181));
#64787=CARTESIAN_POINT('Ctrl Pts',(11.9918856091606,5.47079489740727,8.95469345396048));
#64788=CARTESIAN_POINT('Ctrl Pts',(12.1106906451408,0.532601741995187,10.4800986182537));
#64789=CARTESIAN_POINT('Ctrl Pts',(12.229495681121,-4.53479304595954,9.46318042173016));
#64790=CARTESIAN_POINT('Ctrl Pts',(12.3483007171013,-8.50211132536573,6.15062880321902));
#64791=CARTESIAN_POINT('Ctrl Pts',(12.4671057530815,-10.4069379216217,1.34602182724199));
#64792=CARTESIAN_POINT('Ctrl Pts',(12.5859107890617,-9.78718890495105,-3.7851109630634));
#64793=CARTESIAN_POINT('Ctrl Pts',(12.7047158250419,-6.79320660134877,-7.99802949077405));
#64794=CARTESIAN_POINT('Ctrl Pts',(12.8235208610222,-2.15128867552026,-10.270739442634));
#64795=CARTESIAN_POINT('Ctrl Pts',(12.9423258970024,3.01250138671254,-10.0519136018449));
#64796=CARTESIAN_POINT('Ctrl Pts',(13.0611309329826,7.44550131720053,-7.39463601534687));
#64797=CARTESIAN_POINT('Ctrl Pts',(13.1799359689628,10.0723281742079,-2.94352455654064));
#64798=CARTESIAN_POINT('Ctrl Pts',(13.2987410049431,10.2557509996443,2.2216442328137));
#64799=CARTESIAN_POINT('Ctrl Pts',(13.4175460409233,7.95127401622754,6.84787362491195));
#64800=CARTESIAN_POINT('Ctrl Pts',(13.5363510769035,3.71793067228796,9.81290594981732));
#64801=CARTESIAN_POINT('Ctrl Pts',(13.6551561128838,-1.41732994803981,10.3974663972667));
#64802=CARTESIAN_POINT('Ctrl Pts',(13.773961148864,-6.20876641478464,8.4597488893313));
#64803=CARTESIAN_POINT('Ctrl Pts',(13.8927661848442,-9.49404416364595,4.46981622470548));
#64804=CARTESIAN_POINT('Ctrl Pts',(14.0115712208244,-10.4762013842497,-0.60443049273222));
#64805=CARTESIAN_POINT('Ctrl Pts',(14.1303762568047,-8.91698065775955,-5.53205094092975));
#64806=CARTESIAN_POINT('Ctrl Pts',(14.2491812927849,-5.19462682919267,-9.11767425220551));
#64807=CARTESIAN_POINT('Ctrl Pts',(14.3679863287651,-0.212130169948613,
-10.4914790403879));
#64808=CARTESIAN_POINT('Ctrl Pts',(14.4867913647454,4.82182626140632,-9.32019973867041));
#64809=CARTESIAN_POINT('Ctrl Pts',(14.6055964007256,8.68607599507601,-5.88797210180758));
#64810=CARTESIAN_POINT('Ctrl Pts',(14.7244014367058,10.4432068245734,-1.02740589986761));
#64811=CARTESIAN_POINT('Ctrl Pts',(14.843206472686,9.66696371942952,4.08239440906108));
#64812=CARTESIAN_POINT('Ctrl Pts',(14.9620115086663,6.54565225307114,8.20186370563207));
#64813=CARTESIAN_POINT('Ctrl Pts',(15.0808165446465,1.83645834009328,10.3316771353446));
#64814=CARTESIAN_POINT('Ctrl Pts',(15.1996215806267,-3.31823433289184,9.95517215199806));
#64815=CARTESIAN_POINT('Ctrl Pts',(15.318426616607,-7.6679703954037,7.16368352728626));
#64816=CARTESIAN_POINT('Ctrl Pts',(15.4372316525872,-10.157565539744,2.63438682992933));
#64817=CARTESIAN_POINT('Ctrl Pts',(15.5560366885674,-10.1830792759437,-2.53397476778));
#64818=CARTESIAN_POINT('Ctrl Pts',(15.6748417245476,-7.73832233327883,-7.08763000799124));
#64819=CARTESIAN_POINT('Ctrl Pts',(15.7936467605279,-3.41635808961021,-9.92192668121746));
#64820=CARTESIAN_POINT('Ctrl Pts',(15.9124517965081,1.73436619692707,-10.349304593008));
#64821=CARTESIAN_POINT('Ctrl Pts',(16.0312568324883,6.46435783014953,-8.26608792039404));
#64822=CARTESIAN_POINT('Ctrl Pts',(16.1500618684685,9.62618789133837,-4.17763549685113));
#64823=CARTESIAN_POINT('Ctrl Pts',(16.2688669044488,10.4528412291769,0.924252076827058));
#64824=CARTESIAN_POINT('Ctrl Pts',(16.387671940429,8.74378346239289,5.80192919869627));
#64825=CARTESIAN_POINT('Ctrl Pts',(16.5064769764092,4.91360777791608,9.27214054405468));
#64826=CARTESIAN_POINT('Ctrl Pts',(16.6252820123894,-0.10853949907314,10.493062033603));
#64827=CARTESIAN_POINT('Ctrl Pts',(16.7440870483697,-5.10435663222344,9.16851542153781));
#64828=CARTESIAN_POINT('Ctrl Pts',(16.8628920843499,-8.86192920482737,5.61981693941426));
#64829=CARTESIAN_POINT('Ctrl Pts',(16.9816971203301,-10.4697233774365,0.707830533291434));
#64830=CARTESIAN_POINT('Ctrl Pts',(17.1005021563104,-9.53771107557352,-4.37586552613104));
#64831=CARTESIAN_POINT('Ctrl Pts',(17.2193071922906,-6.29198527163358,-8.39803864038776));
#64832=CARTESIAN_POINT('Ctrl Pts',(17.3381122282708,-1.51991303483393,-10.3829666295545));
#64833=CARTESIAN_POINT('Ctrl Pts',(17.4569172642511,3.62086855820574,-9.84913410143739));
#64834=CARTESIAN_POINT('Ctrl Pts',(17.5757223002313,7.88327876779868,-6.92604125984493));
#64835=CARTESIAN_POINT('Ctrl Pts',(17.6945273362115,10.2333173002494,-2.32278899091503));
#64836=CARTESIAN_POINT('Ctrl Pts',(17.8133323721917,10.1008981213041,2.8439389597766));
#64837=CARTESIAN_POINT('Ctrl Pts',(17.932137408172,7.51814424662471,7.32076763398781));
#64838=CARTESIAN_POINT('Ctrl Pts',(18.0509424441522,3.11159515355942,10.0216818580638));
#64839=CARTESIAN_POINT('Ctrl Pts',(18.1697474801324,-2.0497828143526,10.2914781289125));
#64840=CARTESIAN_POINT('Ctrl Pts',(18.2885525161126,-6.71391252885095,8.06470769580882));
#64841=CARTESIAN_POINT('Ctrl Pts',(18.4073575520929,-9.74934223905273,3.88155349953112));
#64842=CARTESIAN_POINT('Ctrl Pts',(18.5261625880731,-10.4197197269623,-1.24321055153653));
#64843=CARTESIAN_POINT('Ctrl Pts',(18.6449676240533,-8.56242091716224,-6.06638934632804));
#64844=CARTESIAN_POINT('Ctrl Pts',(18.7637726600336,-4.62800017217989,-9.41794808173218));
#64845=CARTESIAN_POINT('Ctrl Pts',(18.8825776960137,0.42910780888478,-10.4848461196268));
#64846=CARTESIAN_POINT('Ctrl Pts',(19.001382731994,5.38212031846822,-9.00826912017127));
#64847=CARTESIAN_POINT('Ctrl Pts',(19.1201877679742,9.02950673474984,-5.34641373174648));
#64848=CARTESIAN_POINT('Ctrl Pts',(19.2389928039545,10.486462817826,-0.387594161788445));
#64849=CARTESIAN_POINT('Ctrl Pts',(19.3577978399347,9.39955167548687,4.66525025735512));
#64850=CARTESIAN_POINT('Ctrl Pts',(19.4766028759149,6.03244254300923,8.58637109780332));
#64851=CARTESIAN_POINT('Ctrl Pts',(19.5954079118952,1.20194836440568,10.4245600287591));
#64852=CARTESIAN_POINT('Ctrl Pts',(19.7142129478754,-3.92012144880135,9.73389847340455));
#64853=CARTESIAN_POINT('Ctrl Pts',(19.8330179838556,-8.09122536945768,6.68193113437607));
#64854=CARTESIAN_POINT('Ctrl Pts',(19.9518230198358,-10.2995127152225,2.00902202398816));
#64855=CARTESIAN_POINT('Ctrl Pts',(20.0706280558161,-10.009284280293,-3.15124734988852));
#64856=CARTESIAN_POINT('Ctrl Pts',(20.1894330917963,-7.29094536875751,-7.54706878819144));
#64857=CARTESIAN_POINT('Ctrl Pts',(20.3082381277765,-2.80392646587668,-10.1120783243533));
#64858=CARTESIAN_POINT('Ctrl Pts',(20.4270431637567,2.36328524967433,-10.2240410060099));
#64859=CARTESIAN_POINT('Ctrl Pts',(20.545848199737,6.95719746515613,-7.85579627375385));
#64860=CARTESIAN_POINT('Ctrl Pts',(20.6646532357172,9.86339219955671,-3.58184672782404));
#64861=CARTESIAN_POINT('Ctrl Pts',(20.7834582716974,10.3768678079984,1.56100805866827));
#64862=CARTESIAN_POINT('Ctrl Pts',(20.9022633076776,8.37306238680994,6.32518441869393));
#64863=CARTESIAN_POINT('Ctrl Pts',(21.0210683436579,4.33807072559066,9.55496070340811));
#64864=CARTESIAN_POINT('Ctrl Pts',(21.1398733796381,-0.74927539795548,10.4668389708602));
#64865=CARTESIAN_POINT('Ctrl Pts',(21.2586784156183,-5.65485793154934,8.83961047998685));
#64866=CARTESIAN_POINT('Ctrl Pts',(21.3774834515986,-9.18865209318669,5.06801779537876));
#64867=CARTESIAN_POINT('Ctrl Pts',(21.4962884875788,-10.4934095136775,0.0669958369101187));
#64868=CARTESIAN_POINT('Ctrl Pts',(21.615093523559,-9.25261453881444,-4.95027836187213));
#64869=CARTESIAN_POINT('Ctrl Pts',(21.7338985595392,-5.76726644021558,-8.76668520430974));
#64870=CARTESIAN_POINT('Ctrl Pts',(21.8527035955195,-0.882861258940293,
-10.4564184911165));
#64871=CARTESIAN_POINT('Ctrl Pts',(21.9715086314997,4.21571354847328,-9.6095728802647));
#64872=CARTESIAN_POINT('Ctrl Pts',(22.0903136674799,8.29161601021562,-6.43158111221775));
#64873=CARTESIAN_POINT('Ctrl Pts',(22.2091187034601,10.3560899683198,-1.69337893927062));
#64874=CARTESIAN_POINT('Ctrl Pts',(22.3279237394404,9.90832330615713,3.45561295931176));
#64875=CARTESIAN_POINT('Ctrl Pts',(22.4467287754206,7.05693786850942,7.7663221401058));
#64876=CARTESIAN_POINT('Ctrl Pts',(22.5655338114008,2.4936393418288,10.19303166368));
#64877=CARTESIAN_POINT('Ctrl Pts',(22.6843388473811,-2.67458073980179,10.1470562002081));
#64878=CARTESIAN_POINT('Ctrl Pts',(22.8031438833613,-7.19398544832653,7.63954874538845));
#64879=CARTESIAN_POINT('Ctrl Pts',(22.9219489193415,-9.96823126771623,3.27879506179086));
#64880=CARTESIAN_POINT('Ctrl Pts',(23.0407539553217,-10.3243254893911,-1.87734782419486));
#64881=CARTESIAN_POINT('Ctrl Pts',(23.159558991302,-8.17588470309968,-6.5780727409721));
#64882=CARTESIAN_POINT('Ctrl Pts',(23.2783640272822,-4.04409018769059,-9.68305046035207));
#64883=CARTESIAN_POINT('Ctrl Pts',(23.3971690632624,1.06874327896542,-10.4390574032125));
#64884=CARTESIAN_POINT('Ctrl Pts',(23.5159740992426,5.92231477645477,-8.66269700223236));
#64885=CARTESIAN_POINT('Ctrl Pts',(23.6347791352229,9.33921666283309,-4.78488910932746));
#64886=CARTESIAN_POINT('Ctrl Pts',(23.7535841712031,10.4905569778446,0.253665051782705));
#64887=CARTESIAN_POINT('Ctrl Pts',(23.8723892071833,9.09703688225833,5.23068366724002));
#64888=CARTESIAN_POINT('Ctrl Pts',(23.9911942431636,5.49670459697617,8.93881257424503));
#64889=CARTESIAN_POINT('Ctrl Pts',(24.1099992791438,0.562949696752003,10.4785122657192));
#64890=CARTESIAN_POINT('Ctrl Pts',(24.228804315124,-4.50736881963169,9.47627342301349));
#64891=CARTESIAN_POINT('Ctrl Pts',(24.3476093511042,-8.48426355601317,6.17522498181294));
#64892=CARTESIAN_POINT('Ctrl Pts',(24.4664143870845,-10.4029962250826,1.37615449889055));
#64893=CARTESIAN_POINT('Ctrl Pts',(24.5852194230647,-9.79810948092905,-3.75675155734687));
#64894=CARTESIAN_POINT('Ctrl Pts',(24.704024459045,-6.81634027291969,-7.97832294079858));
#64895=CARTESIAN_POINT('Ctrl Pts',(24.8228294950251,-2.18102354189972,-10.2644662780672));
#64896=CARTESIAN_POINT('Ctrl Pts',(24.9416345310054,2.98337858259214,-10.0605956034834));
#64897=CARTESIAN_POINT('Ctrl Pts',(25.0604395669856,7.42405535477923,-7.41616705266769));
#64898=CARTESIAN_POINT('Ctrl Pts',(25.1792446029658,10.063761539955,-2.9726815051098));
#64899=CARTESIAN_POINT('Ctrl Pts',(25.2980496389461,10.2621418375906,2.19193443539551));
#64900=CARTESIAN_POINT('Ctrl Pts',(25.4168546749263,7.97107199968254,6.82481815433765));
#64901=CARTESIAN_POINT('Ctrl Pts',(25.5356597109065,3.74633309111811,9.80209773641814));
#64902=CARTESIAN_POINT('Ctrl Pts',(25.6544647468867,-1.38721311801518,10.4015273603979));
#64903=CARTESIAN_POINT('Ctrl Pts',(25.773269782867,-6.18424108959879,8.47769389690486));
#64904=CARTESIAN_POINT('Ctrl Pts',(25.8920748188472,-9.48105983952243,4.49729207226914));
#64905=CARTESIAN_POINT('Ctrl Pts',(26.0108798548275,-10.4779078741575,-0.574089056304778));
#64906=CARTESIAN_POINT('Ctrl Pts',(26.1296848908076,-8.93296399143784,-5.50620431800117));
#64907=CARTESIAN_POINT('Ctrl Pts',(26.2484899267879,-5.22100967646791,-9.10259246710126));
#64908=CARTESIAN_POINT('Ctrl Pts',(26.3672949627681,-0.242512426070257,
-10.4908207203775));
#64909=CARTESIAN_POINT('Ctrl Pts',(26.4860999987483,4.79481490108,-9.33412458285624));
#64910=CARTESIAN_POINT('Ctrl Pts',(26.6049050347286,8.66898810365204,-5.91310214038614));
#64911=CARTESIAN_POINT('Ctrl Pts',(26.7237100707088,10.4401876822764,-1.05764494171864));
#64912=CARTESIAN_POINT('Ctrl Pts',(26.842515106689,9.67874572738195,4.05438192682752));
#64913=CARTESIAN_POINT('Ctrl Pts',(26.9613201426693,6.56937726316331,8.18287321410596));
#64914=CARTESIAN_POINT('Ctrl Pts',(27.0801251786495,1.86637100119828,10.3263154585644));
#64915=CARTESIAN_POINT('Ctrl Pts',(27.1989302146297,-3.28939040832167,9.96473995674454));
#64916=CARTESIAN_POINT('Ctrl Pts',(27.3177352506099,-7.64719233458281,7.18585979975938));
#64917=CARTESIAN_POINT('Ctrl Pts',(27.4365402865902,-10.1498938056816,2.66379192079387));
#64918=CARTESIAN_POINT('Ctrl Pts',(27.5553453225704,-10.1903749225702,-2.50447411672651));
#64919=CARTESIAN_POINT('Ctrl Pts',(27.6741503585506,-7.75881554014436,-7.06519023649855));
#64920=CARTESIAN_POINT('Ctrl Pts',(27.7929553945308,-3.44507749523718,-9.91199135974755));
#64921=CARTESIAN_POINT('Ctrl Pts',(27.9117604305111,1.70438751322266,-10.3542838897082));
#64922=CARTESIAN_POINT('Ctrl Pts',(28.0305654664913,6.44039227206198,-8.28477392847046));
#64923=CARTESIAN_POINT('Ctrl Pts',(28.1493705024715,9.61404916352834,-4.20549525563395));
#64924=CARTESIAN_POINT('Ctrl Pts',(28.2681755384518,10.4554740149348,0.893976949883643));
#64925=CARTESIAN_POINT('Ctrl Pts',(28.386980574432,8.7605490852157,5.77658302021413));
#64926=CARTESIAN_POINT('Ctrl Pts',(28.5057856104122,4.94043913537346,9.25787193763072));
#64927=CARTESIAN_POINT('Ctrl Pts',(28.6245906463924,-0.0781513139439594,
10.4933323608865));
#64928=CARTESIAN_POINT('Ctrl Pts',(28.7433956823727,-5.07778336235737,9.18325910496195));
#64929=CARTESIAN_POINT('Ctrl Pts',(28.8622007183529,-8.84561714879615,5.64545737038407));
#64930=CARTESIAN_POINT('Ctrl Pts',(28.9810057543331,-10.4676296087965,0.738147706727696));
#64931=CARTESIAN_POINT('Ctrl Pts',(29.0998107903134,-9.55034351291589,-4.34822612673321));
#64932=CARTESIAN_POINT('Ctrl Pts',(29.2186158262936,-6.31627946473417,-8.37978194151124));
#64933=CARTESIAN_POINT('Ctrl Pts',(29.3374208622738,-1.54997555683656,-10.378521447543));
#64934=CARTESIAN_POINT('Ctrl Pts',(29.456225898254,3.59233044897795,-9.85957877443276));
#64935=CARTESIAN_POINT('Ctrl Pts',(29.5750309342343,7.8631880120934,-6.94884205824041));
#64936=CARTESIAN_POINT('Ctrl Pts',(29.6938359702145,10.2265476305979,-2.35241476423973));
#64937=CARTESIAN_POINT('Ctrl Pts',(29.8126410061947,10.1090917635981,2.81467500416174));
#64938=CARTESIAN_POINT('Ctrl Pts',(29.9314460421749,7.53931353939529,7.29896451687431));
#64939=CARTESIAN_POINT('Ctrl Pts',(30.0502510781552,3.14060472647248,10.0126287065864));
#64940=CARTESIAN_POINT('Ctrl Pts',(30.1690561141354,-2.01997027245138,10.2973711092838));
#64941=CARTESIAN_POINT('Ctrl Pts',(30.2878611501157,-6.69052911800965,8.08411725452847));
#64942=CARTESIAN_POINT('Ctrl Pts',(30.4066661860958,-9.73806044326235,3.90977115280018));
#64943=CARTESIAN_POINT('Ctrl Pts',(30.5254712220761,-10.4232763499531,-1.21303000639279));
#64944=CARTESIAN_POINT('Ctrl Pts',(30.6442762580563,-8.57995317261452,-6.04156728172768));
#64945=CARTESIAN_POINT('Ctrl Pts',(30.7630812940366,-4.65525498345498,-9.40450597867413));
#64946=CARTESIAN_POINT('Ctrl Pts',(30.8818863300168,0.398742072642834,-10.4860448417601));
#64947=CARTESIAN_POINT('Ctrl Pts',(31.000691365997,5.35600995441259,-9.0238178744993));
#64948=CARTESIAN_POINT('Ctrl Pts',(31.1194964019772,9.01398574706474,-5.37254061088553));
#64949=CARTESIAN_POINT('Ctrl Pts',(31.2383014379574,10.4852963781011,-0.417961155229236));
#64950=CARTESIAN_POINT('Ctrl Pts',(31.3571064739377,9.4130227454641,4.63800975174425));
#64951=CARTESIAN_POINT('Ctrl Pts',(31.4759115099179,6.05728323207572,8.56886524052714));
#64952=CARTESIAN_POINT('Ctrl Pts',(31.5947165458981,1.23213267353085,10.4210354926331));
#64953=CARTESIAN_POINT('Ctrl Pts',(31.7135215818784,-3.89191580512397,9.74521026092953));
#64954=CARTESIAN_POINT('Ctrl Pts',(31.8323266178586,-8.07184068054606,6.70533516625238));
#64955=CARTESIAN_POINT('Ctrl Pts',(31.9511316538388,-10.2936514318129,2.03884081385401));
#64956=CARTESIAN_POINT('Ctrl Pts',(32.0699366898191,-10.018368266652,-3.122247417749));
#64957=CARTESIAN_POINT('Ctrl Pts',(32.1887417257993,-7.31277097856737,-7.52592268621747));
#64958=CARTESIAN_POINT('Ctrl Pts',(32.3075467617795,-2.83319911559344,-10.1039157971204));
#64959=CARTESIAN_POINT('Ctrl Pts',(32.4263517977597,2.33366668990814,-10.2308421669144));
#64960=CARTESIAN_POINT('Ctrl Pts',(32.5451568337399,6.93441803807263,-7.87591125757227));
#64961=CARTESIAN_POINT('Ctrl Pts',(32.6639618697202,9.85297787124923,-3.61039592462831));
#64962=CARTESIAN_POINT('Ctrl Pts',(32.7827669057004,10.3813449468827,1.53095027931453));
#64963=CARTESIAN_POINT('Ctrl Pts',(32.9015719416806,8.39134490245989,6.30090964796831));
#64964=CARTESIAN_POINT('Ctrl Pts',(33.0203769776609,4.36572353887912,9.54235765657405));
#64965=CARTESIAN_POINT('Ctrl Pts',(33.1391820136411,-0.71896046753108,10.4689649684211));
#64966=CARTESIAN_POINT('Ctrl Pts',(33.2579870496213,-5.6292348563709,8.85594978507207));
#64967=CARTESIAN_POINT('Ctrl Pts',(33.3767920856015,-9.17393666806451,5.09460672419782));
#64968=CARTESIAN_POINT('Ctrl Pts',(33.4955971215818,-10.493171492143,0.0973842922511994));
#64969=CARTESIAN_POINT('Ctrl Pts',(33.614402157562,-9.26691166151779,-4.92346218849354));
#64970=CARTESIAN_POINT('Ctrl Pts',(33.7332071935423,-5.79263042786231,-8.74994653641399));
#64971=CARTESIAN_POINT('Ctrl Pts',(33.8520122295224,-0.913139167682674,
-10.4538178922508));
#64972=CARTESIAN_POINT('Ctrl Pts',(33.9708172655027,4.18786671008217,-9.62174121884839));
#64973=CARTESIAN_POINT('Ctrl Pts',(34.0896223014829,8.27295549041769,-6.45556652180641));
#64974=CARTESIAN_POINT('Ctrl Pts',(34.2084273374631,10.3511425446899,-1.72336289951095));
#64975=CARTESIAN_POINT('Ctrl Pts',(34.3272323734434,9.91828915353406,3.42690413212689));
#64976=CARTESIAN_POINT('Ctrl Pts',(34.4460374094236,7.07939941359363,7.74585280048044));
#64977=CARTESIAN_POINT('Ctrl Pts',(34.5648424454038,2.52314773219355,10.1857673832376));
#64978=CARTESIAN_POINT('Ctrl Pts',(34.6836474813841,-2.64518382135331,10.1547591904067));
#64979=CARTESIAN_POINT('Ctrl Pts',(34.8024525173643,-7.17183127748453,7.6603503700023));
#64980=CARTESIAN_POINT('Ctrl Pts',(34.9212575533445,-9.95869413227364,3.30764914156855));
#64981=CARTESIAN_POINT('Ctrl Pts',(35.0400625893247,-10.3297189632094,-1.84744087997725));
#64982=CARTESIAN_POINT('Ctrl Pts',(35.158867625305,-8.19490040588757,-6.55436793302628));
#64983=CARTESIAN_POINT('Ctrl Pts',(35.2776726612852,-4.07211517951482,-9.67129823905069));
#64984=CARTESIAN_POINT('Ctrl Pts',(35.3964776972655,1.03850746384432,-10.4421086908459));
#64985=CARTESIAN_POINT('Ctrl Pts',(35.5152827332456,5.89720291816771,-8.67981159967508));
#64986=CARTESIAN_POINT('Ctrl Pts',(35.6340877692259,9.3253205422193,-4.81191525785339));
#64987=CARTESIAN_POINT('Ctrl Pts',(35.7528928052061,10.4912475967761,0.223283512688066));
#64988=CARTESIAN_POINT('Ctrl Pts',(35.8716978411863,9.11214670637266,5.20431686827785));
#64989=CARTESIAN_POINT('Ctrl Pts',(35.9905028771666,5.5225681971373,8.92285672707276));
#64990=CARTESIAN_POINT('Ctrl Pts',(36.1093079131468,0.593292930198467,10.4768380326736));
#64991=CARTESIAN_POINT('Ctrl Pts',(36.2281129491271,-4.47990679119387,9.48928694929787));
#64992=CARTESIAN_POINT('Ctrl Pts',(36.3469179851072,-8.46634463138618,6.19976937042805));
#64993=CARTESIAN_POINT('Ctrl Pts',(36.4657230210875,-10.3989672813656,1.4062756290952));
#64994=CARTESIAN_POINT('Ctrl Pts',(36.5845280570677,-9.80894788275425,-3.72836064474877));
#64995=CARTESIAN_POINT('Ctrl Pts',(36.7033330930479,-6.83941677764739,-7.9585494787389));
#64996=CARTESIAN_POINT('Ctrl Pts',(36.8221381290282,-2.21074011661143,-10.2581070281365));
#64997=CARTESIAN_POINT('Ctrl Pts',(36.9409431650084,2.95423075766473,-10.0691932295675));
#64998=CARTESIAN_POINT('Ctrl Pts',(37.0597482009886,7.40254712876932,-7.43763589255681));
#64999=CARTESIAN_POINT('Ctrl Pts',(37.1785532369688,10.0551105035959,-3.00181352258519));
#65000=CARTESIAN_POINT('Ctrl Pts',(37.2973582729491,10.2684466096674,2.16220625480307));
#65001=CARTESIAN_POINT('Ctrl Pts',(37.4161633089293,7.99080313186483,6.80170544581863));
#65002=CARTESIAN_POINT('Ctrl Pts',(37.5349683449095,3.77470409044336,9.79120731541779));
#65003=CARTESIAN_POINT('Ctrl Pts',(37.6537733808897,-1.35708465380123,10.4055010886702));
#65004=CARTESIAN_POINT('Ctrl Pts',(37.77257841687,-6.15966389881867,8.49556780430181));
#65005=CARTESIAN_POINT('Ctrl Pts',(37.8913834528501,-9.46799600025767,4.52473020223357));
#65006=CARTESIAN_POINT('Ctrl Pts',(38.0101884888305,-10.4795264886231,-0.5437428051444));
#65007=CARTESIAN_POINT('Ctrl Pts',(38.1289935248106,-8.94887240670967,-5.48031151599342));
#65008=CARTESIAN_POINT('Ctrl Pts',(38.2477985607909,-5.24734873651581,-9.08743434096145));
#65009=CARTESIAN_POINT('Ctrl Pts',(38.3666035967711,-0.27289264830437,-10.4900744166284));
#65010=CARTESIAN_POINT('Ctrl Pts',(38.4854086327514,4.76776332790926,-9.34797114420792));
#65011=CARTESIAN_POINT('Ctrl Pts',(38.6042136687316,8.65182750771774,-5.93818258734095));
#65012=CARTESIAN_POINT('Ctrl Pts',(38.7230187047118,10.4370809808865,-1.08787511338123));
#65013=CARTESIAN_POINT('Ctrl Pts',(38.841823740692,9.69044656225397,4.02633544156494));
#65014=CARTESIAN_POINT('Ctrl Pts',(38.9606287766723,6.59304717762569,8.16381409498656));
#65015=CARTESIAN_POINT('Ctrl Pts',(39.0794338126525,1.89626800954364,10.3208671777074));
#65016=CARTESIAN_POINT('Ctrl Pts',(39.1982388486327,-3.26051889650485,9.9742241898529));
#65017=CARTESIAN_POINT('Ctrl Pts',(39.3170438846129,-7.62635013878093,7.20797580632616));
#65018=CARTESIAN_POINT('Ctrl Pts',(39.4358489205933,-10.1421369471471,2.69317467114161));
#65019=CARTESIAN_POINT('Ctrl Pts',(39.5546539565733,-10.197585105212,-2.47495246131395));
#65020=CARTESIAN_POINT('Ctrl Pts',(39.6734589925537,-7.77924367588624,-7.04269121111839));
#65021=CARTESIAN_POINT('Ctrl Pts',(39.7922640285338,-3.47376800789063,-9.90197290903841));
#65022=CARTESIAN_POINT('Ctrl Pts',(39.9110690645141,1.67439453523271,-10.3591763477472));
#65023=CARTESIAN_POINT('Ctrl Pts',(40.0298741004943,6.41637270018189,-8.30339045437917));
#65024=CARTESIAN_POINT('Ctrl Pts',(40.1486791364745,9.60182980508796,-4.23331974396269));
#65025=CARTESIAN_POINT('Ctrl Pts',(40.2674841724548,10.4580191136734,0.863694325242524));
#65026=CARTESIAN_POINT('Ctrl Pts',(40.386289208435,8.77724123509683,5.75118839534756));
#65027=CARTESIAN_POINT('Ctrl Pts',(40.5050942444152,4.96722905970481,9.24352568732455));
#65028=CARTESIAN_POINT('Ctrl Pts',(40.6238992803954,-0.0477624753722201,
10.493514684447));
#65029=CARTESIAN_POINT('Ctrl Pts',(40.7427043163757,-5.0511675026172,9.19792576873352));
#65030=CARTESIAN_POINT('Ctrl Pts',(40.8615093523559,-8.82923091434941,5.67105045842888));
#65031=CARTESIAN_POINT('Ctrl Pts',(40.9803143883362,-10.4654480365472,0.76845868172124));
#65032=CARTESIAN_POINT('Ctrl Pts',(41.0991194243163,-9.56289588181645,-4.32055024485495));
#65033=CARTESIAN_POINT('Ctrl Pts',(41.2179244602966,-6.34052063122281,-8.36145499271618));
#65034=CARTESIAN_POINT('Ctrl Pts',(41.3367294962768,-1.58002518326458,-10.3739891673947));
#65035=CARTESIAN_POINT('Ctrl Pts',(41.4555345322571,3.56376241212563,-9.86994086638596));
#65036=CARTESIAN_POINT('Ctrl Pts',(41.5743395682372,7.84303092287294,-6.97158436861771));
#65037=CARTESIAN_POINT('Ctrl Pts',(41.6931446042175,10.2196929414599,-2.38202121410348));
#65038=CARTESIAN_POINT('Ctrl Pts',(41.8119496401977,10.1171991785312,2.78538822638215));
#65039=CARTESIAN_POINT('Ctrl Pts',(41.9307546761779,7.56042239424033,7.27709867081222));
#65040=CARTESIAN_POINT('Ctrl Pts',(42.0495597121582,3.16958256444921,10.0034945082114));
#65041=CARTESIAN_POINT('Ctrl Pts',(42.1683647481384,-1.99013036390094,10.3031720737214));
#65042=CARTESIAN_POINT('Ctrl Pts',(42.2871697841186,-6.6671097412949,8.10346994054641));
#65043=CARTESIAN_POINT('Ctrl Pts',(42.4059748200989,-9.72665804500086,3.93793489890507));
#65044=CARTESIAN_POINT('Ctrl Pts',(42.5247798560791,-10.4268208272698,-1.18279844917567));
#65045=CARTESIAN_POINT('Ctrl Pts',(42.6435848920593,-8.59726759665103,-6.01677379735012));
#65046=CARTESIAN_POINT('Ctrl Pts',(42.7623899280396,-4.68275676202098,-9.39082860495563));
#65047=CARTESIAN_POINT('Ctrl Pts',(42.8811949640197,0.368965693322309,-10.4874893880972));
#65048=CARTESIAN_POINT('Ctrl Pts',(42.9603983213399,3.6752100549675,-9.52140074095435));
#65049=CARTESIAN_POINT('Ctrl Pts',(43.,5.1139286979658,-8.67308627433867));
#65050=CARTESIAN_POINT('Ctrl Pts',(0.395021395315363,-4.50147759502411,
9.32427186527549));
#65051=CARTESIAN_POINT('Ctrl Pts',(0.434623073975439,-6.04821693793231,
8.57755270070747));
#65052=CARTESIAN_POINT('Ctrl Pts',(0.513826431295591,-8.76142425767936,
6.3003863176029));
#65053=CARTESIAN_POINT('Ctrl Pts',(0.632631467275819,-10.7060292299026,
1.35285685100163));
#65054=CARTESIAN_POINT('Ctrl Pts',(0.751436503256047,-10.0533834439177,
-3.9214021233163));
#65055=CARTESIAN_POINT('Ctrl Pts',(0.870241539236274,-6.96199392763067,
-8.24510495099076));
#65056=CARTESIAN_POINT('Ctrl Pts',(0.989046575216502,-2.18168968988639,
-10.5682927005514));
#65057=CARTESIAN_POINT('Ctrl Pts',(1.10785161119673,3.1278440783295,-10.3279533344256));
#65058=CARTESIAN_POINT('Ctrl Pts',(1.22665664717696,7.67861625223654,-7.58210014766689));
#65059=CARTESIAN_POINT('Ctrl Pts',(1.34546168315718,10.3666602956518,-2.99698804874303));
#65060=CARTESIAN_POINT('Ctrl Pts',(1.46426671913741,10.539901928427,2.31517731173066));
#65061=CARTESIAN_POINT('Ctrl Pts',(1.58307175511764,8.15631151207012,7.06569978968951));
#65062=CARTESIAN_POINT('Ctrl Pts',(1.70187679109787,3.79411619374502,10.102190743681));
#65063=CARTESIAN_POINT('Ctrl Pts',(1.8206818270781,-1.48847826408105,10.6880297644884));
#65064=CARTESIAN_POINT('Ctrl Pts',(1.93948686305832,-6.40998882175759,8.68110617302293));
#65065=CARTESIAN_POINT('Ctrl Pts',(2.05829189903855,-9.77652704799499,4.56826830400835));
#65066=CARTESIAN_POINT('Ctrl Pts',(2.17709693501878,-10.7714183561408,-0.652766188536676));
#65067=CARTESIAN_POINT('Ctrl Pts',(2.29590197099901,-9.15331628882757,-5.71544912018155));
#65068=CARTESIAN_POINT('Ctrl Pts',(2.41470700697923,-5.31474943313272,-9.39164498035765));
#65069=CARTESIAN_POINT('Ctrl Pts',(2.53351204295946,-0.186899712328668,
-10.7895609729742));
#65070=CARTESIAN_POINT('Ctrl Pts',(2.65231707893969,4.9862892325668,-9.57008238795448));
#65071=CARTESIAN_POINT('Ctrl Pts',(2.77112211491992,8.94987509264377,-6.02903749822585));
#65072=CARTESIAN_POINT('Ctrl Pts',(2.88992715090014,10.7423481279403,-1.02543356820498));
#65073=CARTESIAN_POINT('Ctrl Pts',(3.00873218688037,9.92887978850885,4.22692600405091));
#65074=CARTESIAN_POINT('Ctrl Pts',(3.1275372228606,6.70680596261819,8.45389325047258));
#65075=CARTESIAN_POINT('Ctrl Pts',(3.24634225884083,1.85775608453379,10.6300658338294));
#65076=CARTESIAN_POINT('Ctrl Pts',(3.36514729482105,-3.44195908438213,10.2275351364789));
#65077=CARTESIAN_POINT('Ctrl Pts',(3.48395233080128,-7.90670377204593,7.34394939833388));
#65078=CARTESIAN_POINT('Ctrl Pts',(3.60275736678151,-10.4533942085886,2.67882564283126));
#65079=CARTESIAN_POINT('Ctrl Pts',(3.72156240276174,-10.4642393955512,-2.63614323917428));
#65080=CARTESIAN_POINT('Ctrl Pts',(3.84036743874197,-7.93660844430258,-7.31162114079292));
#65081=CARTESIAN_POINT('Ctrl Pts',(3.95917247472219,-3.48366879238604,-10.2134034018924));
#65082=CARTESIAN_POINT('Ctrl Pts',(4.07797751070242,1.81435952470949,-10.637558781028));
#65083=CARTESIAN_POINT('Ctrl Pts',(4.19678254668265,6.67224994114044,-8.48119319599131));
#65084=CARTESIAN_POINT('Ctrl Pts',(4.31558758266288,9.91154710645243,-4.26741036945542));
#65085=CARTESIAN_POINT('Ctrl Pts',(4.4343926186431,10.7464434480276,0.981585718675386));
#65086=CARTESIAN_POINT('Ctrl Pts',(4.55319765462333,8.97440494873879,5.99246302623709));
#65087=CARTESIAN_POINT('Ctrl Pts',(4.67200269060357,5.02530302841786,9.54965375169893));
#65088=CARTESIAN_POINT('Ctrl Pts',(4.79080772658378,-0.142866168815652,
10.7902338511532));
#65089=CARTESIAN_POINT('Ctrl Pts',(4.90961276256402,-5.27637805873932,9.41325617870981));
#65090=CARTESIAN_POINT('Ctrl Pts',(5.02841779854423,-9.12991542858833,5.75275599791864));
#65091=CARTESIAN_POINT('Ctrl Pts',(5.14722283452447,-10.7686647394821,0.696718762054908));
#65092=CARTESIAN_POINT('Ctrl Pts',(5.2660278705047,-9.79508863920986,-4.52833256892492));
#65093=CARTESIAN_POINT('Ctrl Pts',(5.38483290648492,-6.44536288846001,-8.65487461150229));
#65094=CARTESIAN_POINT('Ctrl Pts',(5.50363794246515,-1.53208346926155,-10.6818667632572));
#65095=CARTESIAN_POINT('Ctrl Pts',(5.62244297844538,3.7528576810432,-10.117589462446));
#65096=CARTESIAN_POINT('Ctrl Pts',(5.74124801442561,8.12740875775467,-7.09892838315313));
#65097=CARTESIAN_POINT('Ctrl Pts',(5.86005305040583,10.5303656825029,-2.35816791122463));
#65098=CARTESIAN_POINT('Ctrl Pts',(5.97885808638606,10.3788051692242,2.95465066700763));
#65099=CARTESIAN_POINT('Ctrl Pts',(6.09766312236629,7.7094936499458,7.55071287801421));
#65100=CARTESIAN_POINT('Ctrl Pts',(6.21646815834651,3.16996825957003,10.3150791823467));
#65101=CARTESIAN_POINT('Ctrl Pts',(6.33527319432675,-2.13854649368404,10.577153501728));
#65102=CARTESIAN_POINT('Ctrl Pts',(6.45407823030696,-6.92828018321643,8.27336032139389));
#65103=CARTESIAN_POINT('Ctrl Pts',(6.57288326628721,-10.03731131434,3.96256720874054));
#65104=CARTESIAN_POINT('Ctrl Pts',(6.69168830226742,-10.711433007704,-1.30948853612137));
#65105=CARTESIAN_POINT('Ctrl Pts',(6.81049333824766,-8.78711289672475,-6.26388092519149));
#65106=CARTESIAN_POINT('Ctrl Pts',(6.92929837422788,-4.73116376151398,-9.69874459744669));
#65107=CARTESIAN_POINT('Ctrl Pts',(7.04810341020811,0.472498634123263,-10.7808303180004));
#65108=CARTESIAN_POINT('Ctrl Pts',(7.16690844618834,5.56153955917688,-9.24763943049658));
#65109=CARTESIAN_POINT('Ctrl Pts',(7.28571348216856,9.30142982654727,-5.47110231000858));
#65110=CARTESIAN_POINT('Ctrl Pts',(7.4045185181488,10.7849250733744,-0.367353326463599));
#65111=CARTESIAN_POINT('Ctrl Pts',(7.52332355412902,9.65215038253687,4.82551036654753));
#65112=CARTESIAN_POINT('Ctrl Pts',(7.64212859010925,6.17790083602382,8.84777365019136));
#65113=CARTESIAN_POINT('Ctrl Pts',(7.76093362608948,1.2049801234898,10.7236924707285));
#65114=CARTESIAN_POINT('Ctrl Pts',(7.8797386620697,-4.06025168542382,9.99819551498056));
#65115=CARTESIAN_POINT('Ctrl Pts',(7.99854369804993,-8.3405239928429,6.84727805989915));
#65116=CARTESIAN_POINT('Ctrl Pts',(8.11734873403016,-10.5975034133492,2.03530801325437));
#65117=CARTESIAN_POINT('Ctrl Pts',(8.23615377001038,-10.2836787340574,-3.27039890524978));
#65118=CARTESIAN_POINT('Ctrl Pts',(8.35495880599062,-7.4751793734424,-7.78275340992027));
#65119=CARTESIAN_POINT('Ctrl Pts',(8.47376384197084,-2.85330746361317,-10.4071222642407));
#65120=CARTESIAN_POINT('Ctrl Pts',(8.59256887795107,2.46073638892106,-10.5068707867283));
#65121=CARTESIAN_POINT('Ctrl Pts',(8.7113739139313,7.17784047645446,-8.05780139984454));
#65122=CARTESIAN_POINT('Ctrl Pts',(8.83017894991153,10.1537022161608,-3.65402361928531));
#65123=CARTESIAN_POINT('Ctrl Pts',(8.94898398589176,10.6664197352621,1.63616849253841));
#65124=CARTESIAN_POINT('Ctrl Pts',(9.06778902187198,8.59161503181458,6.52944932209922));
#65125=CARTESIAN_POINT('Ctrl Pts',(9.18659405785222,4.43260631482062,9.83877830640454));
#65126=CARTESIAN_POINT('Ctrl Pts',(9.30539909383243,-0.801689858328023,
10.7613591463076));
#65127=CARTESIAN_POINT('Ctrl Pts',(9.42420412981267,-5.84150743645588,9.07338680838609));
#65128=CARTESIAN_POINT('Ctrl Pts',(9.54300916579289,-9.46425811864636,5.18433945343097));
#65129=CARTESIAN_POINT('Ctrl Pts',(9.66181420177312,-10.7911139448546,0.0376448393264476));
#65130=CARTESIAN_POINT('Ctrl Pts',(9.78061923775334,-9.50019850090942,-5.11818187915227));
#65131=CARTESIAN_POINT('Ctrl Pts',(9.89942427373357,-5.9046695737293,-9.0324102281639));
#65132=CARTESIAN_POINT('Ctrl Pts',(10.0182293097138,-0.87675151148418,-10.7555038976272));
#65133=CARTESIAN_POINT('Ctrl Pts',(10.137034345694,4.36385403877705,-9.86946478959288));
#65134=CARTESIAN_POINT('Ctrl Pts',(10.2558393816743,8.54585046043201,-6.58923343134073));
#65135=CARTESIAN_POINT('Ctrl Pts',(10.3746444176545,10.6547447048076,-1.7105474504198));
#65136=CARTESIAN_POINT('Ctrl Pts',(10.4934494536347,10.1789489235196,3.58309309356351));
#65137=CARTESIAN_POINT('Ctrl Pts',(10.6122544896149,7.23388442831402,8.00752604632419));
#65138=CARTESIAN_POINT('Ctrl Pts',(10.7310595255952,2.53398211702912,10.4894466934792));
#65139=CARTESIAN_POINT('Ctrl Pts',(10.8498645615754,-2.78062833457752,10.4267762692842));
#65140=CARTESIAN_POINT('Ctrl Pts',(10.9686695975556,-7.42069776989709,7.83471773024457));
#65141=CARTESIAN_POINT('Ctrl Pts',(11.0874746335359,-10.2606111207013,3.34206773338088));
#65142=CARTESIAN_POINT('Ctrl Pts',(11.2062796695161,-10.61144566618,-1.96132051905682));
#65143=CARTESIAN_POINT('Ctrl Pts',(11.3250847054963,-8.38809391896691,-6.78892021689419));
#65144=CARTESIAN_POINT('Ctrl Pts',(11.4438897414765,-4.12990949510587,-9.96962410861105));
#65145=CARTESIAN_POINT('Ctrl Pts',(11.5626947774567,1.13013242742211,-10.7318385191566));
#65146=CARTESIAN_POINT('Ctrl Pts',(11.681499813437,6.11602024360922,-8.89066103754532));
#65147=CARTESIAN_POINT('Ctrl Pts',(11.8003048494172,9.61824824828708,-4.89273522061911));
#65148=CARTESIAN_POINT('Ctrl Pts',(11.9191098853974,10.787225574468,0.292098802304907));
#65149=CARTESIAN_POINT('Ctrl Pts',(12.0379149213777,9.33937489403034,5.40607379652921));
#65150=CARTESIAN_POINT('Ctrl Pts',(12.1567199573579,5.62592425758049,9.20861192323424));
#65151=CARTESIAN_POINT('Ctrl Pts',(12.2755249933381,0.547704148320422,10.7772713369701));
#65152=CARTESIAN_POINT('Ctrl Pts',(12.3943300293183,-4.66338122316779,9.73151750099492));
#65153=CARTESIAN_POINT('Ctrl Pts',(12.5131350652986,-8.7431964171594,6.32503547150017));
#65154=CARTESIAN_POINT('Ctrl Pts',(12.6319401012788,-10.70203610231,1.38418949917172));
#65155=CARTESIAN_POINT('Ctrl Pts',(12.750745137259,-10.0647135391572,-3.89244122363726));
#65156=CARTESIAN_POINT('Ctrl Pts',(12.8695501732393,-6.985834146953,-8.22482088413054));
#65157=CARTESIAN_POINT('Ctrl Pts',(12.9883552092195,-2.21229042061208,-10.5619755916984));
#65158=CARTESIAN_POINT('Ctrl Pts',(13.1071602451997,3.09792360074278,-10.3369447453648));
#65159=CARTESIAN_POINT('Ctrl Pts',(13.22596528118,7.65662527215884,-7.60431763845401));
#65160=CARTESIAN_POINT('Ctrl Pts',(13.3447703171602,10.3579381914762,-3.02699086987778));
#65161=CARTESIAN_POINT('Ctrl Pts',(13.4635753531404,10.5465621377889,2.28464097365887));
#65162=CARTESIAN_POINT('Ctrl Pts',(13.5823803891206,8.1767396156204,7.04205130364076));
#65163=CARTESIAN_POINT('Ctrl Pts',(13.7011854251009,3.82335597467568,10.0911598141976));
#65164=CARTESIAN_POINT('Ctrl Pts',(13.8199904610811,-1.45751962652659,10.6922960042759));
#65165=CARTESIAN_POINT('Ctrl Pts',(13.9387954970613,-6.3848216278666,8.69963275575993));
#65166=CARTESIAN_POINT('Ctrl Pts',(14.0576005330415,-9.76325641235606,4.59656192510799));
#65167=CARTESIAN_POINT('Ctrl Pts',(14.1764055690218,-10.7732635933548,-0.621569668549491));
#65168=CARTESIAN_POINT('Ctrl Pts',(14.295210605002,-9.16982974643052,-5.68891727187536));
#65169=CARTESIAN_POINT('Ctrl Pts',(14.4140156409822,-5.34192519286066,-9.37621419010065));
#65170=CARTESIAN_POINT('Ctrl Pts',(14.5328206769624,-0.218145313662554,
-10.7889744613143));
#65171=CARTESIAN_POINT('Ctrl Pts',(14.6516257129427,4.95855352624183,-9.58448247075233));
#65172=CARTESIAN_POINT('Ctrl Pts',(14.7704307489229,8.93237757223272,-6.05493090066587));
#65173=CARTESIAN_POINT('Ctrl Pts',(14.8892357849031,10.7393334429595,-1.0565389276768));
#65174=CARTESIAN_POINT('Ctrl Pts',(15.0080408208834,9.94107925926152,4.198154411863));
#65175=CARTESIAN_POINT('Ctrl Pts',(15.1268458568636,6.73126017019787,8.43443500335809));
#65176=CARTESIAN_POINT('Ctrl Pts',(15.2456508928438,1.88853278496387,10.6246412280548));
#65177=CARTESIAN_POINT('Ctrl Pts',(15.364455928824,-3.41232588240514,10.2374601038066));
#65178=CARTESIAN_POINT('Ctrl Pts',(15.4832609648043,-7.88540266321364,7.36681628274709));
#65179=CARTESIAN_POINT('Ctrl Pts',(15.6020660007845,-10.4455925399602,2.70908726214061));
#65180=CARTESIAN_POINT('Ctrl Pts',(15.7208710367647,-10.471829741332,-2.60582792473298));
#65181=CARTESIAN_POINT('Ctrl Pts',(15.8396760727449,-7.95774949421017,-7.28860619680897));
#65182=CARTESIAN_POINT('Ctrl Pts',(15.9584811087252,-3.51323202740212,-10.2032719274947));
#65183=CARTESIAN_POINT('Ctrl Pts',(16.0772861447054,1.78354572631557,-10.6427685282968));
#65184=CARTESIAN_POINT('Ctrl Pts',(16.1960911806856,6.64766057004887,-8.50048035408482));
#65185=CARTESIAN_POINT('Ctrl Pts',(16.3148962166659,9.89914719551524,-4.29609614723494));
#65186=CARTESIAN_POINT('Ctrl Pts',(16.4337012526461,10.7492410398595,0.950460084256655));
#65187=CARTESIAN_POINT('Ctrl Pts',(16.5525062886263,8.99172138721932,5.96644817285685));
#65188=CARTESIAN_POINT('Ctrl Pts',(16.6713113246065,5.05293759104645,9.53506051400588));
#65189=CARTESIAN_POINT('Ctrl Pts',(16.7901163605868,-0.111617235190228,
10.7906023417404));
#65190=CARTESIAN_POINT('Ctrl Pts',(16.908921396567,-5.24909530243537,9.42849700698447));
#65191=CARTESIAN_POINT('Ctrl Pts',(17.0277264325472,-9.1132172595298,5.77917195499255));
#65192=CARTESIAN_POINT('Ctrl Pts',(17.1465314685275,-10.7666018967724,0.727901711209732));
#65193=CARTESIAN_POINT('Ctrl Pts',(17.2653365045077,-9.80816153924783,-4.49994716911031));
#65194=CARTESIAN_POINT('Ctrl Pts',(17.3841415404879,-6.47040023101552,-8.63617265663666));
#65195=CARTESIAN_POINT('Ctrl Pts',(17.5029465764682,-1.56301154995544,-10.6773850824755));
#65196=CARTESIAN_POINT('Ctrl Pts',(17.6217516124484,3.72354157615641,-10.1284152479743));
#65197=CARTESIAN_POINT('Ctrl Pts',(17.7405566484286,8.10681630014075,-7.12243545288664));
#65198=CARTESIAN_POINT('Ctrl Pts',(17.8593616844088,10.5234923104641,-2.38865378327797));
#65199=CARTESIAN_POINT('Ctrl Pts',(17.978166720389,10.3873182653814,2.92458143303239));
#65200=CARTESIAN_POINT('Ctrl Pts',(18.0969717563693,7.73132805785142,7.52835465202347));
#65201=CARTESIAN_POINT('Ctrl Pts',(18.2157767923495,3.19982726138682,10.3058557530197));
#65202=CARTESIAN_POINT('Ctrl Pts',(18.3345818283297,-2.1079062685211,10.5833023422698));
#65203=CARTESIAN_POINT('Ctrl Pts',(18.4533868643099,-6.90429161898161,8.29338981025399));
#65204=CARTESIAN_POINT('Ctrl Pts',(18.5721919002902,-10.0257936966592,3.9916184758558));
#65205=CARTESIAN_POINT('Ctrl Pts',(18.6909969362704,-10.7151803473548,-1.27846291632762));
#65206=CARTESIAN_POINT('Ctrl Pts',(18.8098019722506,-8.80521614222957,-6.23840732826769));
#65207=CARTESIAN_POINT('Ctrl Pts',(18.9286070082309,-4.75923132214166,-9.68500255689744));
#65208=CARTESIAN_POINT('Ctrl Pts',(19.0474120442111,0.441275550700383,-10.7821534580583));
#65209=CARTESIAN_POINT('Ctrl Pts',(19.1662170801913,5.53473523038444,-9.26370677614018));
#65210=CARTESIAN_POINT('Ctrl Pts',(19.2850221161716,9.285546602577,-5.49801615095253));
#65211=CARTESIAN_POINT('Ctrl Pts',(19.4038271521518,10.7838159992039,-0.398584746420578));
#65212=CARTESIAN_POINT('Ctrl Pts',(19.522632188132,9.66608450383772,4.79753766732815));
#65213=CARTESIAN_POINT('Ctrl Pts',(19.6414372241122,6.2034979324961,8.82984545200429));
#65214=CARTESIAN_POINT('Ctrl Pts',(19.7602422600925,1.23603070238909,10.7201579003071));
#65215=CARTESIAN_POINT('Ctrl Pts',(19.8790472960727,-4.03128005437112,10.0099120090036));
#65216=CARTESIAN_POINT('Ctrl Pts',(19.9978523320529,-8.3206594166336,6.87140336300752));
#65217=CARTESIAN_POINT('Ctrl Pts',(20.1166573680331,-10.591564756575,2.06598966890988));
#65218=CARTESIAN_POINT('Ctrl Pts',(20.2354624040134,-10.2931066306666,-3.24060383177155));
#65219=CARTESIAN_POINT('Ctrl Pts',(20.3542674399936,-7.49768674936553,-7.76107278107562));
#65220=CARTESIAN_POINT('Ctrl Pts',(20.4730724759738,-2.88343434851185,-10.3988154932466));
#65221=CARTESIAN_POINT('Ctrl Pts',(20.5918775119541,2.43029835025003,-10.5139529784728));
#65222=CARTESIAN_POINT('Ctrl Pts',(20.7106825479343,7.15447512070854,-8.07855451500617));
#65223=CARTESIAN_POINT('Ctrl Pts',(20.8294875839145,10.143077647421,-3.68341324631829));
#65224=CARTESIAN_POINT('Ctrl Pts',(20.9482926198947,10.6711133232926,1.6052718605303));
#65225=CARTESIAN_POINT('Ctrl Pts',(21.067097655875,8.61048817869476,6.50454077005611));
#65226=CARTESIAN_POINT('Ctrl Pts',(21.1859026918552,4.46108066265957,9.82590029595299));
#65227=CARTESIAN_POINT('Ctrl Pts',(21.3047077278354,-0.770521782668894,
10.7636357002268));
#65228=CARTESIAN_POINT('Ctrl Pts',(21.4235127638156,-5.8152065662985,9.09026566696722));
#65229=CARTESIAN_POINT('Ctrl Pts',(21.5423177997959,-9.44920467225451,5.21172604485384));
#65230=CARTESIAN_POINT('Ctrl Pts',(21.6611228357761,-10.7909596749281,0.0688955647392342));
#65231=CARTESIAN_POINT('Ctrl Pts',(21.7799278717564,-9.51498083114538,-5.09064800273012));
#65232=CARTESIAN_POINT('Ctrl Pts',(21.8987329077365,-5.9308025203642,-9.01527252883716));
#65233=CARTESIAN_POINT('Ctrl Pts',(22.0175379437168,-0.907895592120268,
-10.7529197383117));
#65234=CARTESIAN_POINT('Ctrl Pts',(22.136342979697,4.33525393660926,-9.88206105070588));
#65235=CARTESIAN_POINT('Ctrl Pts',(22.2551480156772,8.52673231608858,-6.6139544384986));
#65236=CARTESIAN_POINT('Ctrl Pts',(22.3739530516575,10.6497463090909,-1.7413962377265));
#65237=CARTESIAN_POINT('Ctrl Pts',(22.4927580876377,10.1892828163742,3.55360000460175));
#65238=CARTESIAN_POINT('Ctrl Pts',(22.611563123618,7.25704375382471,7.98654326100085));
#65239=CARTESIAN_POINT('Ctrl Pts',(22.7303681595982,2.56434875112944,10.4820643380655));
#65240=CARTESIAN_POINT('Ctrl Pts',(22.8491731955784,-2.75042090684844,10.4347851985527));
#65241=CARTESIAN_POINT('Ctrl Pts',(22.9679782315586,-7.39797744229131,7.85617509148778));
#65242=CARTESIAN_POINT('Ctrl Pts',(23.0867832675389,-10.2508895226167,3.37176827493685));
#65243=CARTESIAN_POINT('Ctrl Pts',(23.2055883035191,-10.6170811195004,-1.93058172754009));
#65244=CARTESIAN_POINT('Ctrl Pts',(23.3243933394993,-8.4077193426039,-6.7645999704911));
#65245=CARTESIAN_POINT('Ctrl Pts',(23.4431983754796,-4.15876403949162,-9.95762215433964));
#65246=CARTESIAN_POINT('Ctrl Pts',(23.5620034114597,1.09904846571882,-10.7350663609856));
#65247=CARTESIAN_POINT('Ctrl Pts',(23.68080844744,6.09024739305704,-8.90833564680441));
#65248=CARTESIAN_POINT('Ctrl Pts',(23.7996134834202,9.60403863707877,-4.920568987654));
#65249=CARTESIAN_POINT('Ctrl Pts',(23.9184185194005,10.7880262528498,0.260857954810412));
#65250=CARTESIAN_POINT('Ctrl Pts',(24.0372235553806,9.35499162877712,5.37900445531273));
#65251=CARTESIAN_POINT('Ctrl Pts',(24.1560285913609,5.65256865022265,9.19228072674483));
#65252=CARTESIAN_POINT('Ctrl Pts',(24.2748336273411,0.578912646909042,10.775640001968));
#65253=CARTESIAN_POINT('Ctrl Pts',(24.3936386633213,-4.6351793579843,9.74498176622617));
#65254=CARTESIAN_POINT('Ctrl Pts',(24.5124436993016,-8.72484255809005,6.35032909708662));
#65255=CARTESIAN_POINT('Ctrl Pts',(24.6312487352818,-10.6979826353841,1.41517661010394));
#65256=CARTESIAN_POINT('Ctrl Pts',(24.750053771262,-10.0759437779896,-3.86327766120379));
#65257=CARTESIAN_POINT('Ctrl Pts',(24.8688588072422,-7.00962379480096,-8.20455553702481));
#65258=CARTESIAN_POINT('Ctrl Pts',(24.9876638432225,-2.24286844614533,-10.5555245458504));
#65259=CARTESIAN_POINT('Ctrl Pts',(25.1064688792027,3.06797499305006,-10.3458729330484));
#65260=CARTESIAN_POINT('Ctrl Pts',(25.225273915183,7.63457118998693,-7.62645920790152));
#65261=CARTESIAN_POINT('Ctrl Pts',(25.3440789511631,10.3491286425253,-3.05697459021611));
#65262=CARTESIAN_POINT('Ctrl Pts',(25.4628839871434,10.553134193752,2.25408872794007));
#65263=CARTESIAN_POINT('Ctrl Pts',(25.5816890231236,8.19709898888505,7.01834207424971));
#65264=CARTESIAN_POINT('Ctrl Pts',(25.7004940591039,3.85256376989868,10.0800451240869));
#65265=CARTESIAN_POINT('Ctrl Pts',(25.8192990950841,-1.42654880642194,10.6964721197066));
#65266=CARTESIAN_POINT('Ctrl Pts',(25.9381041310643,-6.35960086480098,8.71808661032838));
#65267=CARTESIAN_POINT('Ctrl Pts',(26.0569091670446,-9.74990390592425,4.62481687529434));
#65268=CARTESIAN_POINT('Ctrl Pts',(26.1757142030247,-10.7750184723344,-0.590367873123402));
#65269=CARTESIAN_POINT('Ctrl Pts',(26.294519239005,-9.186266302058,-5.66233774446897));
#65270=CARTESIAN_POINT('Ctrl Pts',(26.4133242749852,-5.36905614974228,-9.36070474727618));
#65271=CARTESIAN_POINT('Ctrl Pts',(26.5321293109654,-0.249389086262369,
-10.7882974740418));
#65272=CARTESIAN_POINT('Ctrl Pts',(26.6509343469457,4.93077623425049,-9.59880216654739));
#65273=CARTESIAN_POINT('Ctrl Pts',(26.7697393829259,8.91480513812109,-6.0807735243219));
#65274=CARTESIAN_POINT('Ctrl Pts',(26.8885444189061,10.7362286901394,-1.08763542503522));
#65275=CARTESIAN_POINT('Ctrl Pts',(27.0073494548864,9.95319535675478,4.16934761024307));
#65276=CARTESIAN_POINT('Ctrl Pts',(27.1261544908666,6.75565792450814,8.41490601918968));
#65277=CARTESIAN_POINT('Ctrl Pts',(27.2449595268468,1.91929364675366,10.6191275160578));
#65278=CARTESIAN_POINT('Ctrl Pts',(27.3637645628271,-3.3826640621457,10.2472992123502));
#65279=CARTESIAN_POINT('Ctrl Pts',(27.4825695988073,-7.86403542159889,7.3896213835759));
#65280=CARTESIAN_POINT('Ctrl Pts',(27.6013746347875,-10.4377032669078,2.73932616107459));
#65281=CARTESIAN_POINT('Ctrl Pts',(27.7201796707677,-10.4793322626475,-2.57549075591409));
#65282=CARTESIAN_POINT('Ctrl Pts',(27.8389847067479,-7.97882380457684,-7.26553012520643));
#65283=CARTESIAN_POINT('Ctrl Pts',(27.9577897427282,-3.54276579787058,-10.1930548809571));
#65284=CARTESIAN_POINT('Ctrl Pts',(28.0765947787084,1.75271696979558,-10.6478890174792));
#65285=CARTESIAN_POINT('Ctrl Pts',(28.1953998146886,6.62301544678623,-8.51969622089868));
#65286=CARTESIAN_POINT('Ctrl Pts',(28.3142048506688,9.88666426304871,-4.32474589479191));
#65287=CARTESIAN_POINT('Ctrl Pts',(28.4330098866491,10.7519484806497,0.919326478580275));
#65288=CARTESIAN_POINT('Ctrl Pts',(28.5518149226293,9.00896241451082,5.94038328045385));
#65289=CARTESIAN_POINT('Ctrl Pts',(28.6706199586096,5.08052977602393,9.52038730828209));
#65290=CARTESIAN_POINT('Ctrl Pts',(28.7894249945897,-0.080367365460473,
10.7908803343996));
#65291=CARTESIAN_POINT('Ctrl Pts',(28.90823003057,-5.22176852335733,9.44365876094848));
#65292=CARTESIAN_POINT('Ctrl Pts',(29.0270350665502,-9.09644266032839,5.80553944367983));
#65293=CARTESIAN_POINT('Ctrl Pts',(29.1458401025304,-10.7644487574201,0.759078555645491));
#65294=CARTESIAN_POINT('Ctrl Pts',(29.2646451385107,-9.82115218082908,-4.47152402942895));
#65295=CARTESIAN_POINT('Ctrl Pts',(29.3834501744909,-6.49538330803559,-8.61739827247514));
#65296=CARTESIAN_POINT('Ctrl Pts',(29.5022552104711,-1.59392652208477,-10.6728138532891));
#65297=CARTESIAN_POINT('Ctrl Pts',(29.6210602464513,3.69419424291127,-10.1391560891627));
#65298=CARTESIAN_POINT('Ctrl Pts',(29.7398652824316,8.08615585280263,-7.14588278863781));
#65299=CARTESIAN_POINT('Ctrl Pts',(29.8586703184118,10.5165306806785,-2.41911962232377));
#65300=CARTESIAN_POINT('Ctrl Pts',(29.9774753543921,10.3957442458476,2.89448767136634));
#65301=CARTESIAN_POINT('Ctrl Pts',(30.0962803903722,7.75309762515328,7.50593328771355));
#65302=CARTESIAN_POINT('Ctrl Pts',(30.2150854263525,3.22965942709844,10.2965458912063));
#65303=CARTESIAN_POINT('Ctrl Pts',(30.3338904623327,-2.0772483649061,10.589362423454));
#65304=CARTESIAN_POINT('Ctrl Pts',(30.452695498313,-6.88024515027933,8.31334974464697));
#65305=CARTESIAN_POINT('Ctrl Pts',(30.5715005342932,-10.0141919952983,4.02063626632234));
#65306=CARTESIAN_POINT('Ctrl Pts',(30.6903055702734,-10.7188378216221,-1.24742657440377));
#65307=CARTESIAN_POINT('Ctrl Pts',(30.8091106062536,-8.82324554071531,-6.21288141147184));
#65308=CARTESIAN_POINT('Ctrl Pts',(30.9279156422339,-4.78725896835465,-9.67117929079346));
#65309=CARTESIAN_POINT('Ctrl Pts',(31.0467206782141,0.410048766416475,-10.7833861710468));
#65310=CARTESIAN_POINT('Ctrl Pts',(31.1655257141943,5.50788448323168,-9.27969642952504));
#65311=CARTESIAN_POINT('Ctrl Pts',(31.2843307501746,9.26958550318347,-5.52488388148891));
#65312=CARTESIAN_POINT('Ctrl Pts',(31.4031357861548,10.7826164840207,-0.429812823552344));
#65313=CARTESIAN_POINT('Ctrl Pts',(31.521940822135,9.67993755824422,4.76952473242949));
#65314=CARTESIAN_POINT('Ctrl Pts',(31.6407458581152,6.22904300187173,8.81184320023894));
#65315=CARTESIAN_POINT('Ctrl Pts',(31.7595508940955,1.26707091502548,10.7165334227567));
#65316=CARTESIAN_POINT('Ctrl Pts',(31.8783559300757,-4.00227461403915,10.0215445525419));
#65317=CARTESIAN_POINT('Ctrl Pts',(31.9971609660559,-8.30072505725463,6.89547103747298));
#65318=CARTESIAN_POINT('Ctrl Pts',(32.1159660020362,-10.5855372711486,2.09665399765623));
#65319=CARTESIAN_POINT('Ctrl Pts',(32.2347710380164,-10.3024482017127,-3.21078158020638));
#65320=CARTESIAN_POINT('Ctrl Pts',(32.3535760739966,-7.52013124417266,-7.73932706216649));
#65321=CARTESIAN_POINT('Ctrl Pts',(32.4723811099768,-2.91353705080895,-10.3904215101375));
#65322=CARTESIAN_POINT('Ctrl Pts',(32.5911861459571,2.39983992930974,-10.5209469924743));
#65323=CARTESIAN_POINT('Ctrl Pts',(32.7099911819373,7.13104976227232,-8.09923987746757));
#65324=CARTESIAN_POINT('Ctrl Pts',(32.8287962179175,10.1323680113717,-3.71277198153824));
#65325=CARTESIAN_POINT('Ctrl Pts',(32.9476012538977,10.675717415518,1.57436176553197));
#65326=CARTESIAN_POINT('Ctrl Pts',(33.066406289878,8.62928911168777,6.4795776661501));
#65327=CARTESIAN_POINT('Ctrl Pts',(33.1852113258582,4.48951759659464,9.81293987827461));
#65328=CARTESIAN_POINT('Ctrl Pts',(33.3040163618384,-0.739347244847647,
10.7658219823802));
#65329=CARTESIAN_POINT('Ctrl Pts',(33.4228213978187,-5.78885692554182,9.10706828789432));
#65330=CARTESIAN_POINT('Ctrl Pts',(33.5416264337989,-9.43407197788229,5.23906892690871));
#65331=CARTESIAN_POINT('Ctrl Pts',(33.6604314697791,-10.7907149040768,0.100145712342985));
#65332=CARTESIAN_POINT('Ctrl Pts',(33.7792365057593,-9.52968336175359,-5.06307143238975));
#65333=CARTESIAN_POINT('Ctrl Pts',(33.8980415417396,-5.9568857269268,-8.99805922080419));
#65334=CARTESIAN_POINT('Ctrl Pts',(34.0168465777198,-0.939032058476067,
-10.7502453971023));
#65335=CARTESIAN_POINT('Ctrl Pts',(34.1356516137,4.30661747581347,-9.89457443358646));
#65336=CARTESIAN_POINT('Ctrl Pts',(34.2544566496803,8.5075426602965,-6.63861997616971));
#65337=CARTESIAN_POINT('Ctrl Pts',(34.3732616856605,10.6446585967686,-1.77223042040338));
#65338=CARTESIAN_POINT('Ctrl Pts',(34.4920667216407,10.1995312544087,3.52407711253673));
#65339=CARTESIAN_POINT('Ctrl Pts',(34.6108717576209,7.28014221642872,7.96549349465162));
#65340=CARTESIAN_POINT('Ctrl Pts',(34.7296767936012,2.5946938787148,10.4745940723507));
#65341=CARTESIAN_POINT('Ctrl Pts',(34.8484818295813,-2.7201904120668,10.4427066140376));
#65342=CARTESIAN_POINT('Ctrl Pts',(34.9672868655616,-7.37519506980545,7.87756656506827));
#65343=CARTESIAN_POINT('Ctrl Pts',(35.0860919015418,-10.2410819530331,3.40144053836394));
#65344=CARTESIAN_POINT('Ctrl Pts',(35.2048969375221,-10.6226275301695,-1.89982674474522));
#65345=CARTESIAN_POINT('Ctrl Pts',(35.3237019735023,-8.42727425292232,-6.74022299117739));
#65346=CARTESIAN_POINT('Ctrl Pts',(35.4425070094825,-4.18758370542302,-9.94553668812497));
#65347=CARTESIAN_POINT('Ctrl Pts',(35.5613120454627,1.06795528658719,-10.7382041706523));
#65348=CARTESIAN_POINT('Ctrl Pts',(35.680117081443,6.06442346521121,-8.92593554420823));
#65349=CARTESIAN_POINT('Ctrl Pts',(35.7989221174232,9.5897484793387,-4.94836148717781));
#65350=CARTESIAN_POINT('Ctrl Pts',(35.9177271534034,10.7887364549087,0.229614919569558));
#65351=CARTESIAN_POINT('Ctrl Pts',(36.0365321893837,9.37052990568324,5.35189000180867));
#65352=CARTESIAN_POINT('Ctrl Pts',(36.1553372253639,5.67916563626647,9.17587243702824));
#65353=CARTESIAN_POINT('Ctrl Pts',(36.2741422613441,0.610116290310253,10.7739182945233));
#65354=CARTESIAN_POINT('Ctrl Pts',(36.3929472973243,-4.60693861877766,9.75836430287265));
#65355=CARTESIAN_POINT('Ctrl Pts',(36.5117523333046,-8.70641552607383,6.37556946414236));
#65356=CARTESIAN_POINT('Ctrl Pts',(36.6305573692848,-10.6938394473072,1.44615185232411));
#65357=CARTESIAN_POINT('Ctrl Pts',(36.749362405265,-10.0870895125465,-3.83408169848251));
#65358=CARTESIAN_POINT('Ctrl Pts',(36.8681674412452,-7.03335465478792,-8.18422138048192));
#65359=CARTESIAN_POINT('Ctrl Pts',(36.9869724772255,-2.27342766133397,-10.5489849736098));
#65360=CARTESIAN_POINT('Ctrl Pts',(37.1057775132057,3.03800065506263,-10.354714352632));
#65361=CARTESIAN_POINT('Ctrl Pts',(37.2245825491859,7.61245307868578,-7.64853681625265));
#65362=CARTESIAN_POINT('Ctrl Pts',(37.3433875851662,10.3402322981697,-3.08693267251687));
#65363=CARTESIAN_POINT('Ctrl Pts',(37.4621926211464,10.5596177433697,2.2235175777754));
#65364=CARTESIAN_POINT('Ctrl Pts',(37.5809976571266,8.21738961524842,6.99457398388005));
#65365=CARTESIAN_POINT('Ctrl Pts',(37.6998026931069,3.88173925468816,10.0688458953039));
#65366=CARTESIAN_POINT('Ctrl Pts',(37.8186077290871,-1.39556602222997,10.7005585266546));
#65367=CARTESIAN_POINT('Ctrl Pts',(37.9374127650673,-6.33432676544503,8.7364673486101));
#65368=CARTESIAN_POINT('Ctrl Pts',(38.0562178010475,-9.73646962962712,4.65303303836466));
#65369=CARTESIAN_POINT('Ctrl Pts',(38.1750228370277,-10.776682984084,-0.559161126438245));
#65370=CARTESIAN_POINT('Ctrl Pts',(38.293827873008,-9.20262581489952,-5.63571072853365));
#65371=CARTESIAN_POINT('Ctrl Pts',(38.4126329089881,-5.39614207776996,-9.34511679869675));
#65372=CARTESIAN_POINT('Ctrl Pts',(38.5314379449685,-0.280630767301916,
-10.7875300081718));
#65373=CARTESIAN_POINT('Ctrl Pts',(38.6502429809486,4.90295758914298,-9.61304135972742));
#65374=CARTESIAN_POINT('Ctrl Pts',(38.7690480169289,8.89715793789664,-6.10656515013863));
#65375=CARTESIAN_POINT('Ctrl Pts',(38.8878530529091,10.7330338954088,-1.11872280068296));
#65376=CARTESIAN_POINT('Ctrl Pts',(39.0066580888894,9.96522797943113,4.14050584140738));
#65377=CARTESIAN_POINT('Ctrl Pts',(39.1254631248695,6.77999902090202,8.39530646143021));
#65378=CARTESIAN_POINT('Ctrl Pts',(39.2442681608499,1.95003841193557,10.6135247442467));
#65379=CARTESIAN_POINT('Ctrl Pts',(39.36307319683,-3.35297387237816,10.2570523795059));
#65380=CARTESIAN_POINT('Ctrl Pts',(39.4818782328103,-7.84260222639748,7.41236450960387));
#65381=CARTESIAN_POINT('Ctrl Pts',(39.6006832687904,-10.4297264556015,2.7695420860061));
#65382=CARTESIAN_POINT('Ctrl Pts',(39.7194883047708,-10.4867468965695,-2.54513198713841));
#65383=CARTESIAN_POINT('Ctrl Pts',(39.8382933407509,-7.99983119866904,-7.24239311951865));
#65384=CARTESIAN_POINT('Ctrl Pts',(39.9570983767312,-3.57226985607901,-10.1827523479751));
#65385=CARTESIAN_POINT('Ctrl Pts',(40.0759034127114,1.7218735136626,-10.6529202056113));
#65386=CARTESIAN_POINT('Ctrl Pts',(40.1947084486916,6.59831477812089,-8.53884063531481));
#65387=CARTESIAN_POINT('Ctrl Pts',(40.3135134846719,9.87409841359704,-4.35335937176901));
#65388=CARTESIAN_POINT('Ctrl Pts',(40.4323185206521,10.7545657479756,0.888185162602149));
#65389=CARTESIAN_POINT('Ctrl Pts',(40.5511235566323,9.02612788546858,5.91426856792521));
#65390=CARTESIAN_POINT('Ctrl Pts',(40.6699285926125,5.1080793530015,9.50563425701323));
#65391=CARTESIAN_POINT('Ctrl Pts',(40.7887336285928,-0.0491168237592284,
10.7910678279104));
#65392=CARTESIAN_POINT('Ctrl Pts',(40.907538664573,-5.1943979467306,9.45874131129767));
#65393=CARTESIAN_POINT('Ctrl Pts',(41.0263437005532,-9.07959177931511,5.83185824699045));
#65394=CARTESIAN_POINT('Ctrl Pts',(41.1451487365335,-10.7622053247075,0.790249025876052));
#65395=CARTESIAN_POINT('Ctrl Pts',(41.2639537725137,-9.83406048355512,-4.44306337277325));
#65396=CARTESIAN_POINT('Ctrl Pts',(41.3827588084939,-6.52031185482594,-8.59855164639482));
#65397=CARTESIAN_POINT('Ctrl Pts',(41.5015638444742,-1.62482823297377,-10.6681530562191));
#65398=CARTESIAN_POINT('Ctrl Pts',(41.6203688804544,3.66481613341659,-10.1498120076484));
#65399=CARTESIAN_POINT('Ctrl Pts',(41.7391739164346,8.06542719100225,-7.16926997788992));
#65400=CARTESIAN_POINT('Ctrl Pts',(41.8579789524149,10.5094816206018,-2.44956558997433));
#65401=CARTESIAN_POINT('Ctrl Pts',(41.976783988395,10.4040815538976,2.86437044039235));
#65402=CARTESIAN_POINT('Ctrl Pts',(42.0955890243753,7.77480504075731,7.48344741571868));
#65403=CARTESIAN_POINT('Ctrl Pts',(42.2143940603555,3.25945895800075,10.2871526843369));
#65404=CARTESIAN_POINT('Ctrl Pts',(42.3331990963358,-2.04656231863566,10.5953278795091));
#65405=CARTESIAN_POINT('Ctrl Pts',(42.4520041323159,-6.85616169585859,8.33325119366114));
#65406=CARTESIAN_POINT('Ctrl Pts',(42.5708091682962,-10.0024662716737,4.04959862103809));
#65407=CARTESIAN_POINT('Ctrl Pts',(42.6896142042764,-10.7224828058137,-1.21633777391285));
#65408=CARTESIAN_POINT('Ctrl Pts',(42.8084192402567,-8.84105093097755,-6.18738488531697));
#65409=CARTESIAN_POINT('Ctrl Pts',(42.9272242762368,-4.81554058484046,-9.65711408271567));
#65410=CARTESIAN_POINT('Ctrl Pts',(43.0460293122172,0.37942805080499,-10.7848716788079));
#65411=CARTESIAN_POINT('Ctrl Pts',(43.1252326695373,3.77942397543446,-9.79138871027069));
#65412=CARTESIAN_POINT('Ctrl Pts',(43.1648343481973,5.2589387927992,-8.91901951616117));
#65413=CARTESIAN_POINT('Ctrl Pts',(0.559855743512691,-4.62560143800145,
9.5813795443546));
#65414=CARTESIAN_POINT('Ctrl Pts',(0.599457422172767,-6.21499060583341,
8.81407032899227));
#65415=CARTESIAN_POINT('Ctrl Pts',(0.678660779492919,-9.00301196435153,
6.47411330956815));
#65416=CARTESIAN_POINT('Ctrl Pts',(0.797465815473146,-11.0012375171796,
1.39016055579626));
#65417=CARTESIAN_POINT('Ctrl Pts',(0.916270851453375,-10.3305956618265,
-4.02953095237981));
#65418=CARTESIAN_POINT('Ctrl Pts',(1.0350758874336,-7.15396410249891,-8.47245565765642));
#65419=CARTESIAN_POINT('Ctrl Pts',(1.15388092341383,-2.24184764975094,-10.8597030377153));
#65420=CARTESIAN_POINT('Ctrl Pts',(1.27268595939406,3.21409132027188,-10.6127365485809));
#65421=CARTESIAN_POINT('Ctrl Pts',(1.39149099537429,7.89034658696693,-7.79116914519064));
#65422=CARTESIAN_POINT('Ctrl Pts',(1.51029603135451,10.6525108164139,-3.07962706362521));
#65423=CARTESIAN_POINT('Ctrl Pts',(1.62910106733474,10.8305294178111,2.37901606223865));
#65424=CARTESIAN_POINT('Ctrl Pts',(1.74790610331497,8.38121382648292,7.26052955229675));
#65425=CARTESIAN_POINT('Ctrl Pts',(1.86671113929519,3.89873523776527,10.3807487751553));
#65426=CARTESIAN_POINT('Ctrl Pts',(1.98551617527542,-1.52952159672593,10.9827417341072));
#65427=CARTESIAN_POINT('Ctrl Pts',(2.10432121125565,-6.58673799560173,8.92047918704855));
#65428=CARTESIAN_POINT('Ctrl Pts',(2.22312624723588,-10.0461052215063,4.69423383547555));
#65429=CARTESIAN_POINT('Ctrl Pts',(2.34193128321611,-11.068429684634,-0.670765577887514));
#65430=CARTESIAN_POINT('Ctrl Pts',(2.46073631919634,-9.40571003505258,-5.87304704090043));
#65431=CARTESIAN_POINT('Ctrl Pts',(2.57954135517656,-5.46129845179964,-9.65061040720532));
#65432=CARTESIAN_POINT('Ctrl Pts',(2.69834639115679,-0.192053289138888,
-11.0870725663861));
#65433=CARTESIAN_POINT('Ctrl Pts',(2.81715142713702,5.12378128238326,-9.83396805183416));
#65434=CARTESIAN_POINT('Ctrl Pts',(2.93595646311724,9.19665914681612,-6.19528231183135));
#65435=CARTESIAN_POINT('Ctrl Pts',(3.05476149909747,11.0385578733168,-1.05370889614266));
#65436=CARTESIAN_POINT('Ctrl Pts',(3.1735665350777,10.2026589398639,4.34347935537351));
#65437=CARTESIAN_POINT('Ctrl Pts',(3.29237157105793,6.89173957888312,8.6870010903358));
#65438=CARTESIAN_POINT('Ctrl Pts',(3.41117660703815,1.90898189198456,10.9231795047394));
#65439=CARTESIAN_POINT('Ctrl Pts',(3.52998164301839,-3.53686774046353,10.5095494170184));
#65440=CARTESIAN_POINT('Ctrl Pts',(3.64878667899861,-8.12472339710296,7.54645162181705));
#65441=CARTESIAN_POINT('Ctrl Pts',(3.76759171497884,-10.7416363321884,2.75269164048099));
#65442=CARTESIAN_POINT('Ctrl Pts',(3.88639675095907,-10.7527805645767,-2.70883231127959));
#65443=CARTESIAN_POINT('Ctrl Pts',(4.00520178693929,-8.15545266145518,-7.51323194418617));
#65444=CARTESIAN_POINT('Ctrl Pts',(4.12400682291953,-3.57972755288038,-10.4950280136692));
#65445=CARTESIAN_POINT('Ctrl Pts',(4.24281185889974,1.86438871445788,-10.9308790626302));
#65446=CARTESIAN_POINT('Ctrl Pts',(4.36161689487998,6.85623070890327,-8.71505380515732));
#65447=CARTESIAN_POINT('Ctrl Pts',(4.4804219308602,10.1848483260483,-4.38508003756695));
#65448=CARTESIAN_POINT('Ctrl Pts',(4.59922696684043,11.042766117851,1.00865198503834));
#65449=CARTESIAN_POINT('Ctrl Pts',(4.71803200282065,9.22186538970676,6.15769933454135));
#65450=CARTESIAN_POINT('Ctrl Pts',(4.83683703880089,5.16387084550579,9.81297611590975));
#65451=CARTESIAN_POINT('Ctrl Pts',(4.95564207478112,-0.146805563721134,
11.087763998523));
#65452=CARTESIAN_POINT('Ctrl Pts',(5.07444711076134,-5.42186902427828,9.67281751321984));
#65453=CARTESIAN_POINT('Ctrl Pts',(5.19325214674157,-9.38166391897448,5.91138261931107));
#65454=CARTESIAN_POINT('Ctrl Pts',(5.3120571827218,-11.0656001396886,0.715930100642075));
#65455=CARTESIAN_POINT('Ctrl Pts',(5.43086221870202,-10.0651786304488,-4.65319691154783));
#65456=CARTESIAN_POINT('Ctrl Pts',(5.54966725468225,-6.62308746760338,-8.89352431586915));
#65457=CARTESIAN_POINT('Ctrl Pts',(5.66847229066248,-1.57432917280051,-10.9764087941435));
#65458=CARTESIAN_POINT('Ctrl Pts',(5.78727732664271,3.8563390619198,-10.3965720985329));
#65459=CARTESIAN_POINT('Ctrl Pts',(5.90608236262293,8.35151410697939,-7.29467439173299));
#65460=CARTESIAN_POINT('Ctrl Pts',(6.02488739860317,10.8207302192305,-2.42319208547587));
#65461=CARTESIAN_POINT('Ctrl Pts',(6.14369243458339,10.6649905729994,3.0361222699875));
#65462=CARTESIAN_POINT('Ctrl Pts',(6.26249747056362,7.92207539872496,7.75891640226891));
#65463=CARTESIAN_POINT('Ctrl Pts',(6.38130250654385,3.25737703461955,10.5995074043473));
#65464=CARTESIAN_POINT('Ctrl Pts',(6.50010754252407,-2.19751482210031,10.8688081668199));
#65465=CARTESIAN_POINT('Ctrl Pts',(6.6189125785043,-7.11932073454899,8.50149014226928));
#65466=CARTESIAN_POINT('Ctrl Pts',(6.73771761448453,-10.3140803589917,4.07183112478187));
#65467=CARTESIAN_POINT('Ctrl Pts',(6.85652265046476,-11.0067902988699,-1.34559640204031));
#65468=CARTESIAN_POINT('Ctrl Pts',(6.97532768644499,-9.02940894249928,-6.43660131665733));
#65469=CARTESIAN_POINT('Ctrl Pts',(7.09413272242521,-4.86162097593691,-9.96617799594263));
#65470=CARTESIAN_POINT('Ctrl Pts',(7.21293775840544,0.485527321933209,-11.0781011721386));
#65471=CARTESIAN_POINT('Ctrl Pts',(7.33174279438566,5.71489357424931,-9.50263404512058));
#65472=CARTESIAN_POINT('Ctrl Pts',(7.4505478303659,9.55790765874424,-5.62196260636793));
#65473=CARTESIAN_POINT('Ctrl Pts',(7.56935286634612,11.082308836388,-0.377482735229612));
#65474=CARTESIAN_POINT('Ctrl Pts',(7.68815790232635,9.91829899111815,4.95856909634882));
#65475=CARTESIAN_POINT('Ctrl Pts',(7.80696293830658,6.34825041060521,9.09174235692651));
#65476=CARTESIAN_POINT('Ctrl Pts',(7.92576797428681,1.23820627212243,11.0193878045996));
#65477=CARTESIAN_POINT('Ctrl Pts',(8.04457301026703,-4.17220915539039,10.2738859797137));
#65478=CARTESIAN_POINT('Ctrl Pts',(8.16337804624726,-8.57050578628349,7.03608505688796));
#65479=CARTESIAN_POINT('Ctrl Pts',(8.28218308222749,-10.8897192073552,2.09142964152301));
#65480=CARTESIAN_POINT('Ctrl Pts',(8.40098811820772,-10.5672411194009,-3.36057695714928));
#65481=CARTESIAN_POINT('Ctrl Pts',(8.51979315418794,-7.68130013516784,-7.99735522494477));
#65482=CARTESIAN_POINT('Ctrl Pts',(8.63859819016817,-2.93198462685639,-10.6940884842215));
#65483=CARTESIAN_POINT('Ctrl Pts',(8.75740322614839,2.52858878864971,-10.796587474679));
#65484=CARTESIAN_POINT('Ctrl Pts',(8.87620826212863,7.37576240884407,-8.2799873942394));
#65485=CARTESIAN_POINT('Ctrl Pts',(8.99501329810886,10.433680626119,-3.75477974755237));
#65486=CARTESIAN_POINT('Ctrl Pts',(9.11381833408908,10.960535829456,1.68128423881622));
#65487=CARTESIAN_POINT('Ctrl Pts',(9.2326233700693,8.82852041512902,6.70949250242752));
#65488=CARTESIAN_POINT('Ctrl Pts',(9.35142840604955,4.5548310995911,10.110072997495));
#65489=CARTESIAN_POINT('Ctrl Pts',(9.47023344202975,-0.82379567225048,11.0580931019259));
#65490=CARTESIAN_POINT('Ctrl Pts',(9.58903847801,-6.0025812919817,9.32357657734583));
#65491=CARTESIAN_POINT('Ctrl Pts',(9.70784351399022,-9.72522578177864,5.32729254442715));
#65492=CARTESIAN_POINT('Ctrl Pts',(9.82664854997045,-11.0886683599476,0.038682858960375));
#65493=CARTESIAN_POINT('Ctrl Pts',(9.94545358595068,-9.7621571849388,-5.25931073972898));
#65494=CARTESIAN_POINT('Ctrl Pts',(10.0642586219309,-6.0674850634282,-9.28147010799242));
#65495=CARTESIAN_POINT('Ctrl Pts',(10.1830636579111,-0.900927077094411,
-11.0520764004887));
#65496=CARTESIAN_POINT('Ctrl Pts',(10.3018686938914,4.48418304676412,-10.1416056304509));
#65497=CARTESIAN_POINT('Ctrl Pts',(10.4206737298716,8.78149393044081,-6.7709251000223));
#65498=CARTESIAN_POINT('Ctrl Pts',(10.5394787658518,10.948538871453,-1.75771412373074));
#65499=CARTESIAN_POINT('Ctrl Pts',(10.658283801832,10.4596234867461,3.68189338194223));
#65500=CARTESIAN_POINT('Ctrl Pts',(10.7770888378123,7.43335171787435,8.2283257470068));
#65501=CARTESIAN_POINT('Ctrl Pts',(10.8958938737925,2.60385419608802,10.7786829290965));
#65502=CARTESIAN_POINT('Ctrl Pts',(11.0146989097727,-2.85730144190588,10.7142844292357));
#65503=CARTESIAN_POINT('Ctrl Pts',(11.1335039457529,-7.62531625467886,8.0507524105894));
#65504=CARTESIAN_POINT('Ctrl Pts',(11.2523089817332,-10.5435374391628,3.43422198313571));
#65505=CARTESIAN_POINT('Ctrl Pts',(11.3711140177134,-10.9040459041746,-2.01540201452063));
#65506=CARTESIAN_POINT('Ctrl Pts',(11.4899190536936,-8.61938740660476,-6.97611805342656));
#65507=CARTESIAN_POINT('Ctrl Pts',(11.6087240896739,-4.24378771106049,-10.2445267447517));
#65508=CARTESIAN_POINT('Ctrl Pts',(11.7275291256541,1.16129472402448,-11.0277584723476));
#65509=CARTESIAN_POINT('Ctrl Pts',(11.8463341616343,6.28466352136386,-9.13581232204993));
#65510=CARTESIAN_POINT('Ctrl Pts',(11.9651391976145,9.88346203866717,-5.02764761003651));
#65511=CARTESIAN_POINT('Ctrl Pts',(12.0839442335948,11.0846727715497,0.30015314115385));
#65512=CARTESIAN_POINT('Ctrl Pts',(12.202749269575,9.5968990243591,5.5551409952166));
#65513=CARTESIAN_POINT('Ctrl Pts',(12.3215543055552,5.7810536177537,9.46253039250801));
#65514=CARTESIAN_POINT('Ctrl Pts',(12.4403593415355,0.562806554645667,11.0744440556864));
#65515=CARTESIAN_POINT('Ctrl Pts',(12.5591643775157,-4.79196940037605,9.99985458025968));
#65516=CARTESIAN_POINT('Ctrl Pts',(12.6779694134959,-8.98428150895305,6.49944213978132));
#65517=CARTESIAN_POINT('Ctrl Pts',(12.7967744494761,-10.9971342829983,1.42235717110146));
#65518=CARTESIAN_POINT('Ctrl Pts',(12.9155794854564,-10.3422381733633,-3.99977148421112));
#65519=CARTESIAN_POINT('Ctrl Pts',(13.0343845214366,-7.17846169255723,-8.45161227748701));
#65520=CARTESIAN_POINT('Ctrl Pts',(13.1531895574168,-2.2732921657039,-10.8532117407627));
#65521=CARTESIAN_POINT('Ctrl Pts',(13.2719945933971,3.18334581477301,-10.6219758888847));
#65522=CARTESIAN_POINT('Ctrl Pts',(13.3907996293773,7.86774922711715,-7.81399926156115));
#65523=CARTESIAN_POINT('Ctrl Pts',(13.5096046653575,10.6435482087445,-3.11045718321492));
#65524=CARTESIAN_POINT('Ctrl Pts',(13.6284097013377,10.8373732759336,2.34763771450406));
#65525=CARTESIAN_POINT('Ctrl Pts',(13.747214737318,8.40220521501328,7.23622898236953));
#65526=CARTESIAN_POINT('Ctrl Pts',(13.8660197732982,3.92878127706338,10.3694136785778));
#65527=CARTESIAN_POINT('Ctrl Pts',(13.9848248092784,-1.49770930501336,10.9871256112851));
#65528=CARTESIAN_POINT('Ctrl Pts',(14.1036298452586,-6.56087684094856,8.93951662218857));
#65529=CARTESIAN_POINT('Ctrl Pts',(14.2224348812389,-10.0324686610662,4.7233076255105));
#65530=CARTESIAN_POINT('Ctrl Pts',(14.3412399172191,-11.0703258024599,-0.63870884436676));
#65531=CARTESIAN_POINT('Ctrl Pts',(14.4600449531993,-9.42267883510151,-5.84578360282098));
#65532=CARTESIAN_POINT('Ctrl Pts',(14.5788499891796,-5.48922355652863,-9.63475412799578));
#65533=CARTESIAN_POINT('Ctrl Pts',(14.6976550251598,-0.224160457376507,
-11.0864698822407));
#65534=CARTESIAN_POINT('Ctrl Pts',(14.81646006114,5.09528079107735,-9.84876520283426));
#65535=CARTESIAN_POINT('Ctrl Pts',(14.9352650971202,9.17867914938943,-6.22188969952415));
#65536=CARTESIAN_POINT('Ctrl Pts',(15.0540701331005,11.0354600613455,-1.08567195548599));
#65537=CARTESIAN_POINT('Ctrl Pts',(15.1728751690807,10.2151947990935,4.31391441466492));
#65538=CARTESIAN_POINT('Ctrl Pts',(15.2916802050609,6.9168680873246,8.66700630108408));
#65539=CARTESIAN_POINT('Ctrl Pts',(15.4104852410412,1.94060722983446,10.917605320765));
#65540=CARTESIAN_POINT('Ctrl Pts',(15.5292902770214,-3.50641743191844,10.5197480556152));
#65541=CARTESIAN_POINT('Ctrl Pts',(15.6480953130016,-8.10283493102359,7.56994903820792));
#65542=CARTESIAN_POINT('Ctrl Pts',(15.7669003489818,-10.7336195401764,2.78378769435189));
#65543=CARTESIAN_POINT('Ctrl Pts',(15.8857053849621,-10.7605802067204,-2.67768108168596));
#65544=CARTESIAN_POINT('Ctrl Pts',(16.0045104209423,-8.17717665514151,-7.48958238562669));
#65545=CARTESIAN_POINT('Ctrl Pts',(16.1233154569225,-3.61010596519403,-10.4846171737718));
#65546=CARTESIAN_POINT('Ctrl Pts',(16.2421204929027,1.83272525570407,-10.9362324635857));
#65547=CARTESIAN_POINT('Ctrl Pts',(16.360925528883,6.83096330994821,-8.73487278777558));
#65548=CARTESIAN_POINT('Ctrl Pts',(16.4797305648632,10.1721064996921,-4.41455679761877));
#65549=CARTESIAN_POINT('Ctrl Pts',(16.5985356008434,11.045640850542,0.976668091686266));
#65550=CARTESIAN_POINT('Ctrl Pts',(16.7173406368236,9.23965931204577,6.13096714701741));
#65551=CARTESIAN_POINT('Ctrl Pts',(16.8361456728039,5.19226740417679,9.79798048395709));
#65552=CARTESIAN_POINT('Ctrl Pts',(16.9549507087841,-0.114694971307305,
11.0881426498777));
#65553=CARTESIAN_POINT('Ctrl Pts',(17.0737557447643,-5.3938339726473,9.68847859243116));
#65554=CARTESIAN_POINT('Ctrl Pts',(17.1925607807446,-9.36450531423223,5.93852697057082));
#65555=CARTESIAN_POINT('Ctrl Pts',(17.3113658167248,-11.0634804161082,0.747972889128046));
#65556=CARTESIAN_POINT('Ctrl Pts',(17.430170852705,-10.0786120029221,-4.62402881208958));
#65557=CARTESIAN_POINT('Ctrl Pts',(17.5489758886852,-6.64881519039745,-8.87430667288556));
#65558=CARTESIAN_POINT('Ctrl Pts',(17.6677809246655,-1.60611006507696,-10.9718035353965));
#65559=CARTESIAN_POINT('Ctrl Pts',(17.7865859606457,3.82621459410709,-10.4076963945113));
#65560=CARTESIAN_POINT('Ctrl Pts',(17.9053909966259,8.3303538324828,-7.31882964592835));
#65561=CARTESIAN_POINT('Ctrl Pts',(18.0241960326061,10.8136673206787,-2.45451857564091));
#65562=CARTESIAN_POINT('Ctrl Pts',(18.1430010685864,10.6737384094587,3.00522390628817));
#65563=CARTESIAN_POINT('Ctrl Pts',(18.2618061045666,7.94451186907812,7.73594167005914));
#65564=CARTESIAN_POINT('Ctrl Pts',(18.3806111405468,3.28805936921423,10.5900296479756));
#65565=CARTESIAN_POINT('Ctrl Pts',(18.4994161765271,-2.1660297226896,10.8751265556271));
#65566=CARTESIAN_POINT('Ctrl Pts',(18.6182212125073,-7.09467070911227,8.52207192469913));
#65567=CARTESIAN_POINT('Ctrl Pts',(18.7370262484875,-10.3022451542656,4.10168345218049));
#65568=CARTESIAN_POINT('Ctrl Pts',(18.8558312844677,-11.0106409677473,-1.31371528111871));
#65569=CARTESIAN_POINT('Ctrl Pts',(18.974636320448,-9.0480113672969,-6.41042531020733));
#65570=CARTESIAN_POINT('Ctrl Pts',(19.0934413564282,-4.89046247210343,-9.95205703206272));
#65571=CARTESIAN_POINT('Ctrl Pts',(19.2122463924084,0.453443292515987,-11.0794607964897));
#65572=CARTESIAN_POINT('Ctrl Pts',(19.3310514283887,5.68735014230065,-9.5191444321091));
#65573=CARTESIAN_POINT('Ctrl Pts',(19.4498564643689,9.54158647040418,-5.64961857015859));
#65574=CARTESIAN_POINT('Ctrl Pts',(19.5686615003491,11.0811691805817,-0.409575331052704));
#65575=CARTESIAN_POINT('Ctrl Pts',(19.6874665363294,9.93261733218861,4.92982507730117));
#65576=CARTESIAN_POINT('Ctrl Pts',(19.8062715723096,6.37455332198295,9.07331980620529));
#65577=CARTESIAN_POINT('Ctrl Pts',(19.9250766082898,1.2701130403725,11.015755771855));
#65578=CARTESIAN_POINT('Ctrl Pts',(20.04388164427,-4.1424386599409,10.2859255446026));
#65579=CARTESIAN_POINT('Ctrl Pts',(20.1626866802503,-8.55009346380952,7.06087559163894));
#65580=CARTESIAN_POINT('Ctrl Pts',(20.2814917162305,-10.8836167979275,2.12295731383161));
#65581=CARTESIAN_POINT('Ctrl Pts',(20.4002967522107,-10.5769289810401,-3.32996031365458));
#65582=CARTESIAN_POINT('Ctrl Pts',(20.519101788191,-7.70442812997353,-7.97507677395982));
#65583=CARTESIAN_POINT('Ctrl Pts',(20.6379068241712,-2.96294223114701,-10.68555266214));
#65584=CARTESIAN_POINT('Ctrl Pts',(20.7567118601514,2.49731145082573,-10.8038649509356));
#65585=CARTESIAN_POINT('Ctrl Pts',(20.8755168961316,7.35175277626096,-8.3013127562585));
#65586=CARTESIAN_POINT('Ctrl Pts',(20.9943219321119,10.4227630952853,-3.78497976481254));
#65587=CARTESIAN_POINT('Ctrl Pts',(21.113126968092,10.9653588385869,1.64953566239232));
#65588=CARTESIAN_POINT('Ctrl Pts',(21.2319320040723,8.84791397057959,6.68389712141829));
#65589=CARTESIAN_POINT('Ctrl Pts',(21.3507370400525,4.58409059972847,10.0968398884979));
#65590=CARTESIAN_POINT('Ctrl Pts',(21.4695420760328,-0.791768167382311,
11.0604324295934));
#65591=CARTESIAN_POINT('Ctrl Pts',(21.588347112013,-5.97555520104765,9.34092085394759));
#65592=CARTESIAN_POINT('Ctrl Pts',(21.7071521479932,-9.70975725132234,5.35543429432891));
#65593=CARTESIAN_POINT('Ctrl Pts',(21.8259571839734,-11.0885098361787,0.0707952925683478));
#65594=CARTESIAN_POINT('Ctrl Pts',(21.9447622199537,-9.77734712347633,-5.2310176435881));
#65595=CARTESIAN_POINT('Ctrl Pts',(22.0635672559339,-6.09433860051282,-9.2638598533646));
#65596=CARTESIAN_POINT('Ctrl Pts',(22.1823722919141,-0.932929925300243,
-11.0494209855069));
#65597=CARTESIAN_POINT('Ctrl Pts',(22.3011773278944,4.45479432474524,-10.1545492211471));
#65598=CARTESIAN_POINT('Ctrl Pts',(22.4199823638746,8.76184862196152,-6.79632776477945));
#65599=CARTESIAN_POINT('Ctrl Pts',(22.5387873998548,10.9434026498621,-1.78941353618239));
#65600=CARTESIAN_POINT('Ctrl Pts',(22.657592435835,10.4702423265913,3.65158704989175));
#65601=CARTESIAN_POINT('Ctrl Pts',(22.7763974718153,7.45714963914,8.20676438189589));
#65602=CARTESIAN_POINT('Ctrl Pts',(22.8952025077955,2.63505816043006,10.771097012451));
#65603=CARTESIAN_POINT('Ctrl Pts',(23.0140075437757,-2.82626107389507,10.7225141968974));
#65604=CARTESIAN_POINT('Ctrl Pts',(23.132812579756,-7.60196943625612,8.07280143758712));
#65605=CARTESIAN_POINT('Ctrl Pts',(23.2516176157362,-10.5335477775172,3.46474148808284));
#65606=CARTESIAN_POINT('Ctrl Pts',(23.3704226517164,-10.9098367496098,-1.98381563088531));
#65607=CARTESIAN_POINT('Ctrl Pts',(23.4892276876966,-8.63955398210809,-6.95112720001011));
#65608=CARTESIAN_POINT('Ctrl Pts',(23.6080327236768,-4.27343789129267,-10.2321938483272));
#65609=CARTESIAN_POINT('Ctrl Pts',(23.7268377596571,1.12935365247223,-11.0310753187588));
#65610=CARTESIAN_POINT('Ctrl Pts',(23.8456427956373,6.25818000965933,-9.15397429137645));
#65611=CARTESIAN_POINT('Ctrl Pts',(23.9644478316175,9.86886061132446,-5.05624886598056));
#65612=CARTESIAN_POINT('Ctrl Pts',(24.0832528675977,11.085495527855,0.268050857838114));
#65613=CARTESIAN_POINT('Ctrl Pts',(24.202057903578,9.61294637529592,5.52732524338546));
#65614=CARTESIAN_POINT('Ctrl Pts',(24.3208629395582,5.80843270346912,9.44574887924464));
#65615=CARTESIAN_POINT('Ctrl Pts',(24.4396679755385,0.594875597066088,11.0727677382169));
#65616=CARTESIAN_POINT('Ctrl Pts',(24.5584730115187,-4.76298989633692,10.0136901094388));
#65617=CARTESIAN_POINT('Ctrl Pts',(24.6772780474989,-8.96542156016692,6.5254332123603));
#65618=CARTESIAN_POINT('Ctrl Pts',(24.7960830834791,-10.9929690456855,1.45419872131733));
#65619=CARTESIAN_POINT('Ctrl Pts',(24.9148881194594,-10.3537780750502,-3.96980376506072));
#65620=CARTESIAN_POINT('Ctrl Pts',(25.0336931554395,-7.20290731668222,-8.43078813325103));
#65621=CARTESIAN_POINT('Ctrl Pts',(25.1524981914198,-2.30471335039094,-10.8465828136336));
#65622=CARTESIAN_POINT('Ctrl Pts',(25.2713032274001,3.152571403508,-10.6311502626134));
#65623=CARTESIAN_POINT('Ctrl Pts',(25.3901082633803,7.84508702519461,-7.83675136313537));
#65624=CARTESIAN_POINT('Ctrl Pts',(25.5089132993605,10.6344957450956,-3.14126767532242));
#65625=CARTESIAN_POINT('Ctrl Pts',(25.6277183353407,10.8441265499134,2.31624302048462));
#65626=CARTESIAN_POINT('Ctrl Pts',(25.746523371321,8.42312597808756,7.21186599416179));
#65627=CARTESIAN_POINT('Ctrl Pts',(25.8653284073012,3.95879444867925,10.3579925117557));
#65628=CARTESIAN_POINT('Ctrl Pts',(25.9841334432814,-1.46588449482872,10.9914168790152));
#65629=CARTESIAN_POINT('Ctrl Pts',(26.1029384792616,-6.53496064000315,8.95847932375191));
#65630=CARTESIAN_POINT('Ctrl Pts',(26.2217435152419,-10.0187479723261,4.75234167831954));
#65631=CARTESIAN_POINT('Ctrl Pts',(26.3405485512221,-11.0721290705114,-0.60664668994202));
#65632=CARTESIAN_POINT('Ctrl Pts',(26.4593535872023,-9.43956861267816,-5.81847117093678));
#65633=CARTESIAN_POINT('Ctrl Pts',(26.5781586231826,-5.51710262301666,-9.61881702745111));
#65634=CARTESIAN_POINT('Ctrl Pts',(26.6969636591628,-0.256265746454476,
-11.0857742277062));
#65635=CARTESIAN_POINT('Ctrl Pts',(26.815768695143,5.06673756742096,-9.86347975023855));
#65636=CARTESIAN_POINT('Ctrl Pts',(26.9345737311232,9.16062217259013,-6.24844490825766));
#65637=CARTESIAN_POINT('Ctrl Pts',(27.0533787671035,11.0322696980024,-1.11762590835179));
#65638=CARTESIAN_POINT('Ctrl Pts',(27.1721838030837,10.2276449861276,4.28431329365864));
#65639=CARTESIAN_POINT('Ctrl Pts',(27.2909888390639,6.94193858585298,8.64693882427338));
#65640=CARTESIAN_POINT('Ctrl Pts',(27.4097938750442,1.97221629230903,10.9119395735511));
#65641=CARTESIAN_POINT('Ctrl Pts',(27.5285989110243,-3.47593771596974,10.5298584679558));
#65642=CARTESIAN_POINT('Ctrl Pts',(27.6474039470046,-8.08087850861496,7.59338296739243));
#65643=CARTESIAN_POINT('Ctrl Pts',(27.7662089829848,-10.7255127281339,2.8148604013553));
#65644=CARTESIAN_POINT('Ctrl Pts',(27.8850140189651,-10.7682896027249,-2.64650739510166));
#65645=CARTESIAN_POINT('Ctrl Pts',(28.0038190549453,-8.19883206900931,-7.46587001391433));
#65646=CARTESIAN_POINT('Ctrl Pts',(28.1226240909255,-3.640454100504,-10.4741184021666));
#65647=CARTESIAN_POINT('Ctrl Pts',(28.2414291269057,1.80104642636852,-10.9414941452503));
#65648=CARTESIAN_POINT('Ctrl Pts',(28.3602341628859,6.80563862151046,-8.75461851332687));
#65649=CARTESIAN_POINT('Ctrl Pts',(28.4790391988662,10.1592793625691,-4.44399653394987));
#65650=CARTESIAN_POINT('Ctrl Pts',(28.5978442348464,11.0484229463646,0.9446760072769));
#65651=CARTESIAN_POINT('Ctrl Pts',(28.7166492708266,9.25737574380593,6.1041835406936));
#65652=CARTESIAN_POINT('Ctrl Pts',(28.8354543068069,5.22062041667441,9.78290267893343));
#65653=CARTESIAN_POINT('Ctrl Pts',(28.9542593427871,-0.0825834169769951,
11.0884283079128));
#65654=CARTESIAN_POINT('Ctrl Pts',(29.0730643787673,-5.36575368435728,9.70405841693499));
#65655=CARTESIAN_POINT('Ctrl Pts',(29.1918694147476,-9.34726817186065,5.9656215169756));
#65656=CARTESIAN_POINT('Ctrl Pts',(29.3106744507278,-11.0612679060438,0.780009404563282));
#65657=CARTESIAN_POINT('Ctrl Pts',(29.429479486708,-10.0919608487423,-4.59482193212467));
#65658=CARTESIAN_POINT('Ctrl Pts',(29.5482845226883,-6.674487151337,-8.85501460343903));
#65659=CARTESIAN_POINT('Ctrl Pts',(29.6670895586685,-1.637877487333,-10.9671062590352));
#65660=CARTESIAN_POINT('Ctrl Pts',(29.7858945946487,3.79605803684459,-10.4187334038926));
#65661=CARTESIAN_POINT('Ctrl Pts',(29.9046996306289,8.30912369351186,-7.34292351903524));
#65662=CARTESIAN_POINT('Ctrl Pts',(30.0235046666091,10.8065137307592,-2.4858244804078));
#65663=CARTESIAN_POINT('Ctrl Pts',(30.1423097025894,10.682396728097,2.97430033857092));
#65664=CARTESIAN_POINT('Ctrl Pts',(30.2611147385696,7.96688171091128,7.71290205855278));
#65665=CARTESIAN_POINT('Ctrl Pts',(30.3799197745498,3.31871412772438,10.5804630758263));
#65666=CARTESIAN_POINT('Ctrl Pts',(30.4987248105301,-2.13452645736081,10.8813537376242));
#65667=CARTESIAN_POINT('Ctrl Pts',(30.6175298465103,-7.06996118254902,8.5425822347655));
#65668=CARTESIAN_POINT('Ctrl Pts',(30.7363348824905,-10.2903235473343,4.1315013798445));
#65669=CARTESIAN_POINT('Ctrl Pts',(30.8551399184707,-11.0143992932911,-1.28182314241475));
#65670=CARTESIAN_POINT('Ctrl Pts',(30.973944954451,-9.06653790881608,-6.38419554121599));
#65671=CARTESIAN_POINT('Ctrl Pts',(31.0927499904312,-4.91926295325431,-9.93785260291279));
#65672=CARTESIAN_POINT('Ctrl Pts',(31.2115550264114,0.421355460190115,-11.0807275003336));
#65673=CARTESIAN_POINT('Ctrl Pts',(31.3303600623916,5.65975901205077,-9.53557498455079));
#65674=CARTESIAN_POINT('Ctrl Pts',(31.4491650983719,9.52518525930219,-5.67722715209228));
#65675=CARTESIAN_POINT('Ctrl Pts',(31.5679701343521,11.0799365899403,-0.441664491875456));
#65676=CARTESIAN_POINT('Ctrl Pts',(31.6867751703324,9.94685237102434,4.90103971311473));
#65677=CARTESIAN_POINT('Ctrl Pts',(31.8055802063125,6.40080277166773,9.05482115995073));
#65678=CARTESIAN_POINT('Ctrl Pts',(31.9243852422929,1.30200915652012,11.0120313528803));
#65679=CARTESIAN_POINT('Ctrl Pts',(32.043190278273,-4.11263342295433,10.2978788441543));
#65680=CARTESIAN_POINT('Ctrl Pts',(32.1619953142533,-8.52960943396321,7.08560690869358));
#65681=CARTESIAN_POINT('Ctrl Pts',(32.2808003502334,-10.8774231104844,2.15446718145846));
#65682=CARTESIAN_POINT('Ctrl Pts',(32.3996053862137,-10.5865281367733,-3.29931574266375));
#65683=CARTESIAN_POINT('Ctrl Pts',(32.5184104221939,-7.72749150977794,-7.95273143811551));
#65684=CARTESIAN_POINT('Ctrl Pts',(32.6372154581741,-2.99387498602447,-10.6769272231545));
#65685=CARTESIAN_POINT('Ctrl Pts',(32.7560204941544,2.46601316871136,-10.8110518180343));
#65686=CARTESIAN_POINT('Ctrl Pts',(32.8748255301346,7.32768148647199,-8.32256849736289));
#65687=CARTESIAN_POINT('Ctrl Pts',(32.9936305661149,10.4117581514942,-3.81514803844816));
#65688=CARTESIAN_POINT('Ctrl Pts',(33.112435602095,10.9700898841534,1.6177732517494));
#65689=CARTESIAN_POINT('Ctrl Pts',(33.2312406380753,8.86723332091563,6.6582456843319));
#65690=CARTESIAN_POINT('Ctrl Pts',(33.3500456740555,4.61331165431016,10.0835220999752));
#65691=CARTESIAN_POINT('Ctrl Pts',(33.4688507100358,-0.759734022164224,
11.0626789963393));
#65692=CARTESIAN_POINT('Ctrl Pts',(33.587655746016,-5.94847899471272,9.35818679071654));
#65693=CARTESIAN_POINT('Ctrl Pts',(33.7064607819962,-9.6942072877001,5.3835311296196));
#65694=CARTESIAN_POINT('Ctrl Pts',(33.8252658179765,-11.0882583160105,0.102907132434762));
#65695=CARTESIAN_POINT('Ctrl Pts',(33.9440708539566,-9.7924550619894,-5.20268067628595));
#65696=CARTESIAN_POINT('Ctrl Pts',(34.0628758899369,-6.1211410259913,-9.2461719051944));
#65697=CARTESIAN_POINT('Ctrl Pts',(34.1816809259171,-0.964924949269453,
-11.0466729019537));
#65698=CARTESIAN_POINT('Ctrl Pts',(34.3004859618973,4.42536824154476,-10.1674076483246));
#65699=CARTESIAN_POINT('Ctrl Pts',(34.4192909978776,8.74212983017532,-6.82167343053299));
#65700=CARTESIAN_POINT('Ctrl Pts',(34.5380960338578,10.9381746488474,-1.82109794129582));
#65701=CARTESIAN_POINT('Ctrl Pts',(34.656901069838,10.4807733552833,3.62125009294656));
#65702=CARTESIAN_POINT('Ctrl Pts',(34.7757061058182,7.48088501926381,8.1851341888228));
#65703=CARTESIAN_POINT('Ctrl Pts',(34.8945111417985,2.66624002523605,10.7634207614638));
#65704=CARTESIAN_POINT('Ctrl Pts',(35.0133161777787,-2.79519700278029,10.7306540376684));
#65705=CARTESIAN_POINT('Ctrl Pts',(35.132121213759,-7.57855886212637,8.09478276013425));
#65706=CARTESIAN_POINT('Ctrl Pts',(35.2509262497391,-10.5234697737925,3.49523193515934));
#65707=CARTESIAN_POINT('Ctrl Pts',(35.3697312857194,-10.9155360971296,-1.95221260951319));
#65708=CARTESIAN_POINT('Ctrl Pts',(35.4885363216996,-8.65964809995706,-6.92607804932851));
#65709=CARTESIAN_POINT('Ctrl Pts',(35.6073413576799,-4.30305223133123,-10.2197751371993));
#65710=CARTESIAN_POINT('Ctrl Pts',(35.7261463936601,1.09740310933007,-11.0342996504588));
#65711=CARTESIAN_POINT('Ctrl Pts',(35.8449514296403,6.23164401225468,-9.17205948874139));
#65712=CARTESIAN_POINT('Ctrl Pts',(35.9637564656205,9.85417641645815,-5.08480771650223));
#65713=CARTESIAN_POINT('Ctrl Pts',(36.0825615016008,11.0862253130412,0.235946326451047));
#65714=CARTESIAN_POINT('Ctrl Pts',(36.201366537581,9.62891310499385,5.4994631353395));
#65715=CARTESIAN_POINT('Ctrl Pts',(36.3201715735612,5.83576307539561,9.42888814698371));
#65716=CARTESIAN_POINT('Ctrl Pts',(36.4389766095415,0.626939650422058,11.0709985563729));
#65717=CARTESIAN_POINT('Ctrl Pts',(36.5577816455217,-4.73397044636147,10.0274416564474));
#65718=CARTESIAN_POINT('Ctrl Pts',(36.6765866815019,-8.94648642076145,6.55136955785668));
#65719=CARTESIAN_POINT('Ctrl Pts',(36.7953917174821,-10.9887116132488,1.48602807555302));
#65720=CARTESIAN_POINT('Ctrl Pts',(36.9141967534624,-10.3652311423388,-3.93980275221625));
#65721=CARTESIAN_POINT('Ctrl Pts',(37.0330017894426,-7.22729253192845,-8.40989328222494));
#65722=CARTESIAN_POINT('Ctrl Pts',(37.1518068254228,-2.33611520605651,-10.8398629190831));
#65723=CARTESIAN_POINT('Ctrl Pts',(37.270611861403,3.12177055246052,-10.6402354756965));
#65724=CARTESIAN_POINT('Ctrl Pts',(37.3894168973832,7.82235902860223,-7.8594377399485));
#65725=CARTESIAN_POINT('Ctrl Pts',(37.5082219333635,10.6253540927435,-3.17205182244854));
#65726=CARTESIAN_POINT('Ctrl Pts',(37.6270269693437,10.8507888770719,2.28482890074772));
#65727=CARTESIAN_POINT('Ctrl Pts',(37.7458320053239,8.44397609863201,7.18744252194146));
#65728=CARTESIAN_POINT('Ctrl Pts',(37.8646370413042,3.98877441893296,10.34648447519));
#65729=CARTESIAN_POINT('Ctrl Pts',(37.9834420772844,-1.43404739065872,10.9956159646391));
#65730=CARTESIAN_POINT('Ctrl Pts',(38.1022471132647,-6.50898963207139,8.9773668929184));
#65731=CARTESIAN_POINT('Ctrl Pts',(38.2210521492448,-10.0049432589966,4.78133587449576));
#65732=CARTESIAN_POINT('Ctrl Pts',(38.3398571852251,-11.0738394795448,-0.574579447732101));
#65733=CARTESIAN_POINT('Ctrl Pts',(38.4586622212053,-9.45637922308937,-5.79110994107388));
#65734=CARTESIAN_POINT('Ctrl Pts',(38.5774672571856,-5.54493541902412,-9.60279925643206));
#65735=CARTESIAN_POINT('Ctrl Pts',(38.6962722931657,-0.288368886299457,
-11.0849855997153));
#65736=CARTESIAN_POINT('Ctrl Pts',(38.815077329146,5.03815185037667,-9.87811157524692));
#65737=CARTESIAN_POINT('Ctrl Pts',(38.9338823651262,9.14248836807556,-6.27494771293632));
#65738=CARTESIAN_POINT('Ctrl Pts',(39.0526874011065,11.0289868099311,-1.14957048798467));
#65739=CARTESIAN_POINT('Ctrl Pts',(39.1714924370867,10.2400093966084,4.2546762412498));
#65740=CARTESIAN_POINT('Ctrl Pts',(39.2902974730669,6.9669508641783,8.62679882787384));
#65741=CARTESIAN_POINT('Ctrl Pts',(39.4091025090471,2.00380881432751,10.906182310786));
#65742=CARTESIAN_POINT('Ctrl Pts',(39.5279075450274,-3.44542884825149,10.5398805691588));
#65743=CARTESIAN_POINT('Ctrl Pts',(39.6467125810076,-8.05885431401402,7.61675321288158));
#65744=CARTESIAN_POINT('Ctrl Pts',(39.7655176169878,-10.7173159640559,2.84590950087059));
#65745=CARTESIAN_POINT('Ctrl Pts',(39.884322652968,-10.775908687927,-2.61531151296288));
#65746=CARTESIAN_POINT('Ctrl Pts',(40.0031276889483,-8.22041872145184,-7.44209502791889));
#65747=CARTESIAN_POINT('Ctrl Pts',(40.1219327249285,-3.67077170426739,-10.4635317869118));
#65748=CARTESIAN_POINT('Ctrl Pts',(40.2407377609087,1.76935249209249,-10.9466640634754));
#65749=CARTESIAN_POINT('Ctrl Pts',(40.359542796889,6.78025685605987,-8.77429081625043));
#65750=CARTESIAN_POINT('Ctrl Pts',(40.4783478328692,10.1463670221061,-4.47339899957534));
#65751=CARTESIAN_POINT('Ctrl Pts',(40.5971528688494,11.0511123822778,0.912675999961777));
#65752=CARTESIAN_POINT('Ctrl Pts',(40.7159579048297,9.27501453584036,6.07734874050287));
#65753=CARTESIAN_POINT('Ctrl Pts',(40.8347629408098,5.24892964629817,9.76774282670191));
#65754=CARTESIAN_POINT('Ctrl Pts',(40.9535679767901,-0.0504711721462242,
11.0886209713737));
#65755=CARTESIAN_POINT('Ctrl Pts',(41.0723730127703,-5.33762839084401,9.71955685386182));
#65756=CARTESIAN_POINT('Ctrl Pts',(41.1911780487505,-9.32995264428081,5.99266603555205));
#65757=CARTESIAN_POINT('Ctrl Pts',(41.3099830847308,-11.0589626128679,0.812039370030842));
#65758=CARTESIAN_POINT('Ctrl Pts',(41.4287881207109,-10.1052250852938,-4.56557650069153));
#65759=CARTESIAN_POINT('Ctrl Pts',(41.5475931566913,-6.70010307842909,-8.83564830007348));
#65760=CARTESIAN_POINT('Ctrl Pts',(41.6663981926714,-1.66963128268295,-10.9623169450435));
#65761=CARTESIAN_POINT('Ctrl Pts',(41.7852032286517,3.76586985470756,-10.4296831489108));
#65762=CARTESIAN_POINT('Ctrl Pts',(41.9040082646319,8.28782345913155,-7.36695558716213));
#65763=CARTESIAN_POINT('Ctrl Pts',(42.0228133006121,10.7992702997436,-2.51710996584518));
#65764=CARTESIAN_POINT('Ctrl Pts',(42.1416183365924,10.6909639292641,2.94335265440253));
#65765=CARTESIAN_POINT('Ctrl Pts',(42.2604233725726,7.98918768727431,7.68979616062515));
#65766=CARTESIAN_POINT('Ctrl Pts',(42.3792284085528,3.34933535155228,10.5708108604624));
#65767=CARTESIAN_POINT('Ctrl Pts',(42.498033444533,-2.10299427337038,10.8874836852967));
#65768=CARTESIAN_POINT('Ctrl Pts',(42.6168384805133,-7.04521365042229,8.56303244677587));
#65769=CARTESIAN_POINT('Ctrl Pts',(42.7356435164936,-10.2782744983466,4.16126234317112));
#65770=CARTESIAN_POINT('Ctrl Pts',(42.8544485524737,-11.0181447843576,-1.24987709865003));
#65771=CARTESIAN_POINT('Ctrl Pts',(42.973253588454,-9.08483426530408,-6.35799597328381));
#65772=CARTESIAN_POINT('Ctrl Pts',(43.0920586244342,-4.94832440765994,-9.92339956047573));
#65773=CARTESIAN_POINT('Ctrl Pts',(43.2108636604144,0.389890408287668,-11.0822539695185));
#65774=CARTESIAN_POINT('Ctrl Pts',(43.2900670177346,3.88363789590143,-10.061376679587));
#65775=CARTESIAN_POINT('Ctrl Pts',(43.3296686963946,5.40394888763259,-9.16495275798366));
#65776=CARTESIAN_POINT('Ctrl Pts',(0.724690091710019,-4.7497252809788,9.83848722343372));
#65777=CARTESIAN_POINT('Ctrl Pts',(0.764291770370095,-6.38176427373451,
9.05058795727707));
#65778=CARTESIAN_POINT('Ctrl Pts',(0.843495127690246,-9.24459967102367,
6.6478403015334));
#65779=CARTESIAN_POINT('Ctrl Pts',(0.962300163670475,-11.2964458044567,
1.42746426059089));
#65780=CARTESIAN_POINT('Ctrl Pts',(1.0811051996507,-10.6078078797354,-4.13765978144332));
#65781=CARTESIAN_POINT('Ctrl Pts',(1.19991023563093,-7.34593427736715,-8.69980636432208));
#65782=CARTESIAN_POINT('Ctrl Pts',(1.31871527161116,-2.30200560961547,-11.1511133748792));
#65783=CARTESIAN_POINT('Ctrl Pts',(1.43752030759139,3.30033856221425,-10.8975197627363));
#65784=CARTESIAN_POINT('Ctrl Pts',(1.55632534357161,8.10207692169732,-8.00023814271438));
#65785=CARTESIAN_POINT('Ctrl Pts',(1.67513037955184,10.9383613371761,-3.16226607850738));
#65786=CARTESIAN_POINT('Ctrl Pts',(1.79393541553207,11.1211569071951,2.44285481274663));
#65787=CARTESIAN_POINT('Ctrl Pts',(1.91274045151229,8.6061161408957,7.45535931490402));
#65788=CARTESIAN_POINT('Ctrl Pts',(2.03154548749252,4.00335428178553,10.6593068066296));
#65789=CARTESIAN_POINT('Ctrl Pts',(2.15035052347275,-1.57056492937082,11.277453703726));
#65790=CARTESIAN_POINT('Ctrl Pts',(2.26915555945298,-6.76348716944584,9.15985220107415));
#65791=CARTESIAN_POINT('Ctrl Pts',(2.38796059543321,-10.3156833950177,4.82019936694276));
#65792=CARTESIAN_POINT('Ctrl Pts',(2.50676563141343,-11.3654410131272,-0.688764967238368));
#65793=CARTESIAN_POINT('Ctrl Pts',(2.62557066739367,-9.65810378127762,-6.0306449616193));
#65794=CARTESIAN_POINT('Ctrl Pts',(2.74437570337389,-5.60784747046655,-9.90957583405303));
#65795=CARTESIAN_POINT('Ctrl Pts',(2.86318073935412,-0.197206865949118,
-11.3845841597981));
#65796=CARTESIAN_POINT('Ctrl Pts',(2.98198577533434,5.26127333219972,-10.0978537157138));
#65797=CARTESIAN_POINT('Ctrl Pts',(3.10079081131458,9.44344320098848,-6.36152712543684));
#65798=CARTESIAN_POINT('Ctrl Pts',(3.2195958472948,11.3347676186933,-1.08198422408035));
#65799=CARTESIAN_POINT('Ctrl Pts',(3.33840088327503,10.476438091219,4.46003270669612));
#65800=CARTESIAN_POINT('Ctrl Pts',(3.45720591925525,7.07667319514803,8.92010893019902));
#65801=CARTESIAN_POINT('Ctrl Pts',(3.57601095523549,1.96020769943535,11.2162931756495));
#65802=CARTESIAN_POINT('Ctrl Pts',(3.69481599121571,-3.63177639654495,10.7915636975579));
#65803=CARTESIAN_POINT('Ctrl Pts',(3.81362102719593,-8.34274302215997,7.74895384530025));
#65804=CARTESIAN_POINT('Ctrl Pts',(3.93242606317617,-11.0298784557883,2.8265576381307));
#65805=CARTESIAN_POINT('Ctrl Pts',(4.05123109915639,-11.0413217336023,-2.78152138338488));
#65806=CARTESIAN_POINT('Ctrl Pts',(4.17003613513662,-8.37429687860779,-7.71484274757944));
#65807=CARTESIAN_POINT('Ctrl Pts',(4.28884117111685,-3.67578631337471,-10.776652625446));
#65808=CARTESIAN_POINT('Ctrl Pts',(4.40764620709708,1.91441790420627,-11.2241993442323));
#65809=CARTESIAN_POINT('Ctrl Pts',(4.5264512430773,7.04021147666608,-8.94891441432332));
#65810=CARTESIAN_POINT('Ctrl Pts',(4.64525627905754,10.4581495456442,-4.50274970567849));
#65811=CARTESIAN_POINT('Ctrl Pts',(4.76406131503776,11.3390887876744,1.03571825140128));
#65812=CARTESIAN_POINT('Ctrl Pts',(4.88286635101799,9.46932583067473,6.32293564284563));
#65813=CARTESIAN_POINT('Ctrl Pts',(5.00167138699822,5.30243866259372,10.0762984801205));
#65814=CARTESIAN_POINT('Ctrl Pts',(5.12047642297844,-0.150744958626614,
11.3852941458927));
#65815=CARTESIAN_POINT('Ctrl Pts',(5.23928145895868,-5.56735998981724,9.93237884772986));
#65816=CARTESIAN_POINT('Ctrl Pts',(5.35808649493889,-9.63341240936064,6.07000924070351));
#65817=CARTESIAN_POINT('Ctrl Pts',(5.47689153091913,-11.362535539895,0.735141439229234));
#65818=CARTESIAN_POINT('Ctrl Pts',(5.59569656689935,-10.3352686216877,-4.77806125417073));
#65819=CARTESIAN_POINT('Ctrl Pts',(5.71450160287958,-6.80081204674675,-9.13217402023604));
#65820=CARTESIAN_POINT('Ctrl Pts',(5.83330663885981,-1.61657487633946,-11.2709508250297));
#65821=CARTESIAN_POINT('Ctrl Pts',(5.95211167484003,3.95982044279639,-10.6755547346197));
#65822=CARTESIAN_POINT('Ctrl Pts',(6.07091671082027,8.57561945620412,-7.49042040031286));
#65823=CARTESIAN_POINT('Ctrl Pts',(6.18972174680049,11.1110947559581,-2.48821625972711));
#65824=CARTESIAN_POINT('Ctrl Pts',(6.30852678278072,10.9511759767746,3.11759387296738));
#65825=CARTESIAN_POINT('Ctrl Pts',(6.42733181876094,8.13465714750414,7.9671199265236));
#65826=CARTESIAN_POINT('Ctrl Pts',(6.54613685474117,3.34478580966904,10.8839356263479));
#65827=CARTESIAN_POINT('Ctrl Pts',(6.6649418907214,-2.25648315051658,11.1604628319118));
#65828=CARTESIAN_POINT('Ctrl Pts',(6.78374692670163,-7.31036128588154,8.72961996314467));
#65829=CARTESIAN_POINT('Ctrl Pts',(6.90255196268185,-10.5908494036434,4.18109504082322));
#65830=CARTESIAN_POINT('Ctrl Pts',(7.02135699866209,-11.3021475900358,-1.38170426795924));
#65831=CARTESIAN_POINT('Ctrl Pts',(7.14016203464231,-9.27170498827382,-6.60932170812317));
#65832=CARTESIAN_POINT('Ctrl Pts',(7.25896707062254,-4.99207819035984,-10.2336113944386));
#65833=CARTESIAN_POINT('Ctrl Pts',(7.37777210660277,0.498556009743158,-11.3753720262767));
#65834=CARTESIAN_POINT('Ctrl Pts',(7.496577142583,5.86824758932174,-9.75762865974459));
#65835=CARTESIAN_POINT('Ctrl Pts',(7.61538217856323,9.8143854909412,-5.77282290272728));
#65836=CARTESIAN_POINT('Ctrl Pts',(7.73418721454345,11.3796925994017,-0.387612143995621));
#65837=CARTESIAN_POINT('Ctrl Pts',(7.85299225052368,10.1844475996994,5.09162782615011));
#65838=CARTESIAN_POINT('Ctrl Pts',(7.9717972865039,6.51859998518659,9.33571106366168));
#65839=CARTESIAN_POINT('Ctrl Pts',(8.09060232248414,1.27143242075507,11.3150831384706));
#65840=CARTESIAN_POINT('Ctrl Pts',(8.20940735846436,-4.28416662535695,10.5495764444468));
#65841=CARTESIAN_POINT('Ctrl Pts',(8.32821239444459,-8.80048757972408,7.22489205387676));
#65842=CARTESIAN_POINT('Ctrl Pts',(8.44701743042481,-11.1819350013612,2.14755126979166));
#65843=CARTESIAN_POINT('Ctrl Pts',(8.56582246640505,-10.8508035047444,-3.4507550090488));
#65844=CARTESIAN_POINT('Ctrl Pts',(8.68462750238527,-7.8874208968933,-8.21195703996925));
#65845=CARTESIAN_POINT('Ctrl Pts',(8.8034325383655,-3.01066179009962,-10.9810547042023));
#65846=CARTESIAN_POINT('Ctrl Pts',(8.92223757434573,2.59644118837836,-11.0863041626298));
#65847=CARTESIAN_POINT('Ctrl Pts',(9.04104261032595,7.5736843412337,-8.50217338863428));
#65848=CARTESIAN_POINT('Ctrl Pts',(9.15984764630619,10.7136590360772,-3.85553587581941));
#65849=CARTESIAN_POINT('Ctrl Pts',(9.2786526822864,11.2546519236499,1.72639998509404));
#65850=CARTESIAN_POINT('Ctrl Pts',(9.39745771826665,9.06542579844344,6.88953568275583));
#65851=CARTESIAN_POINT('Ctrl Pts',(9.51626275424685,4.67705588436159,10.3813676885855));
#65852=CARTESIAN_POINT('Ctrl Pts',(9.6350677902271,-0.845901486172953,11.3548270575443));
#65853=CARTESIAN_POINT('Ctrl Pts',(9.75387282620731,-6.1636551475075,9.57376634630559));
#65854=CARTESIAN_POINT('Ctrl Pts',(9.87267786218755,-9.98619344491093,5.47024563542331));
#65855=CARTESIAN_POINT('Ctrl Pts',(9.99148289816778,-11.3862227750406,0.0397208785943149));
#65856=CARTESIAN_POINT('Ctrl Pts',(10.110287934148,-10.0241158689682,-5.4004396003057));
#65857=CARTESIAN_POINT('Ctrl Pts',(10.2290929701282,-6.2303005531271,-9.53052998782092));
#65858=CARTESIAN_POINT('Ctrl Pts',(10.3478980061085,-0.925102642704641,
-11.3486489033501));
#65859=CARTESIAN_POINT('Ctrl Pts',(10.4667030420887,4.60451205475118,-10.413746471309));
#65860=CARTESIAN_POINT('Ctrl Pts',(10.5855080780689,9.01713740044963,-6.95261676870385));
#65861=CARTESIAN_POINT('Ctrl Pts',(10.7043131140491,11.2423330380984,-1.80488079704169));
#65862=CARTESIAN_POINT('Ctrl Pts',(10.8231181500293,10.7402980499726,3.78069367032094));
#65863=CARTESIAN_POINT('Ctrl Pts',(10.9419231860096,7.6328190074347,8.44912544768943));
#65864=CARTESIAN_POINT('Ctrl Pts',(11.0607282219898,2.67372627514691,11.0679191647138));
#65865=CARTESIAN_POINT('Ctrl Pts',(11.1795332579701,-2.93397454923425,11.0017925891873));
#65866=CARTESIAN_POINT('Ctrl Pts',(11.2983382939503,-7.82993473946065,8.26678709093423));
#65867=CARTESIAN_POINT('Ctrl Pts',(11.4171433299305,-10.8264637576244,3.52637623289054));
#65868=CARTESIAN_POINT('Ctrl Pts',(11.5359483659107,-11.1966461421692,-2.06948350998442));
#65869=CARTESIAN_POINT('Ctrl Pts',(11.654753401891,-8.85068089424261,-7.16331588995894));
#65870=CARTESIAN_POINT('Ctrl Pts',(11.7735584378712,-4.35766592701509,-10.5194293808923));
#65871=CARTESIAN_POINT('Ctrl Pts',(11.8923634738514,1.19245702062684,-11.3236784255386));
#65872=CARTESIAN_POINT('Ctrl Pts',(12.0111685098316,6.45330679911851,-9.38096360655451));
#65873=CARTESIAN_POINT('Ctrl Pts',(12.1299735458119,10.1486758290472,-5.16255999945393));
#65874=CARTESIAN_POINT('Ctrl Pts',(12.2487785817921,11.3821199686315,0.308207480002802));
#65875=CARTESIAN_POINT('Ctrl Pts',(12.3675836177723,9.85442315468784,5.704208193904));
#65876=CARTESIAN_POINT('Ctrl Pts',(12.4863886537525,5.93618297792691,9.71644886178178));
#65877=CARTESIAN_POINT('Ctrl Pts',(12.6051936897328,0.577908960970914,11.3716167744028));
#65878=CARTESIAN_POINT('Ctrl Pts',(12.723998725713,-4.92055757758432,10.2681916595244));
#65879=CARTESIAN_POINT('Ctrl Pts',(12.8428037616932,-9.2253666007467,6.67384880806248));
#65880=CARTESIAN_POINT('Ctrl Pts',(12.9616087976735,-11.2922324636866,1.46052484303119));
#65881=CARTESIAN_POINT('Ctrl Pts',(13.0804138336537,-10.6197628075694,-4.10710174478497));
#65882=CARTESIAN_POINT('Ctrl Pts',(13.1992188696339,-7.37108923816147,-8.6784036708435));
#65883=CARTESIAN_POINT('Ctrl Pts',(13.3180239056141,-2.3342939107957,-11.1444478898271));
#65884=CARTESIAN_POINT('Ctrl Pts',(13.4368289415944,3.26876802880323,-10.9070070324046));
#65885=CARTESIAN_POINT('Ctrl Pts',(13.5556339775746,8.07887318207548,-8.0236808846683));
#65886=CARTESIAN_POINT('Ctrl Pts',(13.6744390135549,10.9291582260128,-3.19392349655205));
#65887=CARTESIAN_POINT('Ctrl Pts',(13.793244049535,11.1281844140782,2.41063445534924));
#65888=CARTESIAN_POINT('Ctrl Pts',(13.9120490855153,8.62767081440613,7.43040666109832));
#65889=CARTESIAN_POINT('Ctrl Pts',(14.0308541214955,4.03420657945111,10.6476675429581));
#65890=CARTESIAN_POINT('Ctrl Pts',(14.1496591574758,-1.53789898350016,11.2819552182943));
#65891=CARTESIAN_POINT('Ctrl Pts',(14.268464193456,-6.73693205403051,9.17940048861721));
#65892=CARTESIAN_POINT('Ctrl Pts',(14.3872692294362,-10.3016809097763,4.85005332591301));
#65893=CARTESIAN_POINT('Ctrl Pts',(14.5060742654164,-11.3673880115649,-0.655848020184032));
#65894=CARTESIAN_POINT('Ctrl Pts',(14.6248793013967,-9.67552792377249,-6.0026499337666));
#65895=CARTESIAN_POINT('Ctrl Pts',(14.7436843373769,-5.63652192019662,-9.89329406589092));
#65896=CARTESIAN_POINT('Ctrl Pts',(14.8624893733571,-0.230175601090452,
-11.3839653031671));
#65897=CARTESIAN_POINT('Ctrl Pts',(14.9812944093373,5.23200805591287,-10.1130479349162));
#65898=CARTESIAN_POINT('Ctrl Pts',(15.1000994453176,9.42498072654614,-6.38884849838243));
#65899=CARTESIAN_POINT('Ctrl Pts',(15.2189044812978,11.3315866797316,-1.11480498329518));
#65900=CARTESIAN_POINT('Ctrl Pts',(15.337709517278,10.4893103389255,4.42967441746683));
#65901=CARTESIAN_POINT('Ctrl Pts',(15.4565145532582,7.10247600445132,8.89957759881011));
#65902=CARTESIAN_POINT('Ctrl Pts',(15.5753195892385,1.99268167470505,11.2105694134751));
#65903=CARTESIAN_POINT('Ctrl Pts',(15.6941246252187,-3.60050898143174,10.8020360074237));
#65904=CARTESIAN_POINT('Ctrl Pts',(15.8129296611989,-8.32026719883354,7.77308179366874));
#65905=CARTESIAN_POINT('Ctrl Pts',(15.9317346971792,-11.0216465403926,2.85848812656316));
#65906=CARTESIAN_POINT('Ctrl Pts',(16.0505397331594,-11.0493306721087,-2.74953423863894));
#65907=CARTESIAN_POINT('Ctrl Pts',(16.1693447691396,-8.39660381607284,-7.69055857444444));
#65908=CARTESIAN_POINT('Ctrl Pts',(16.2881498051199,-3.70697990298594,-10.765962420049));
#65909=CARTESIAN_POINT('Ctrl Pts',(16.4069548411001,1.88190478509257,-11.2296963988745));
#65910=CARTESIAN_POINT('Ctrl Pts',(16.5257598770803,7.01426604984754,-8.96926522146634));
#65911=CARTESIAN_POINT('Ctrl Pts',(16.6445649130605,10.445065803869,-4.53301744800261));
#65912=CARTESIAN_POINT('Ctrl Pts',(16.7633699490408,11.3420406612246,1.00287609911588));
#65913=CARTESIAN_POINT('Ctrl Pts',(16.882174985021,9.4875972368722,6.29548612117796));
#65914=CARTESIAN_POINT('Ctrl Pts',(17.0009800210012,5.33159721730714,10.0609004539083));
#65915=CARTESIAN_POINT('Ctrl Pts',(17.1197850569814,-0.117772707424389,
11.3856829580151));
#65916=CARTESIAN_POINT('Ctrl Pts',(17.2385900929617,-5.53857264285922,9.94846017787783));
#65917=CARTESIAN_POINT('Ctrl Pts',(17.3573951289419,-9.61579336893467,6.0978819861491));
#65918=CARTESIAN_POINT('Ctrl Pts',(17.4762001649221,-11.3603589354441,0.768044067046353));
#65919=CARTESIAN_POINT('Ctrl Pts',(17.5950052009023,-10.3490624665965,-4.74811045506887));
#65920=CARTESIAN_POINT('Ctrl Pts',(17.7138102368826,-6.82723014977938,-9.11244068913444));
#65921=CARTESIAN_POINT('Ctrl Pts',(17.8326152728628,-1.64920858019848,-11.2662219883175));
#65922=CARTESIAN_POINT('Ctrl Pts',(17.951420308843,3.92888761205777,-10.6869775410482));
#65923=CARTESIAN_POINT('Ctrl Pts',(18.0702253448232,8.55389136482486,-7.51522383897009));
#65924=CARTESIAN_POINT('Ctrl Pts',(18.1890303808035,11.1038423308934,-2.52038336800384));
#65925=CARTESIAN_POINT('Ctrl Pts',(18.3078354167837,10.9601585535361,3.08586637954394));
#65926=CARTESIAN_POINT('Ctrl Pts',(18.426640452764,8.15769568030482,7.94352868809483));
#65927=CARTESIAN_POINT('Ctrl Pts',(18.5454454887442,3.37629147704163,10.8742035429316));
#65928=CARTESIAN_POINT('Ctrl Pts',(18.6642505247244,-2.22415317685811,11.1669507689844));
#65929=CARTESIAN_POINT('Ctrl Pts',(18.7830555607046,-7.28504979924292,8.7507540391443));
#65930=CARTESIAN_POINT('Ctrl Pts',(18.9018605966848,-10.5786966118721,4.21174842850516));
#65931=CARTESIAN_POINT('Ctrl Pts',(19.0206656326651,-11.3061015881399,-1.34896764590979));
#65932=CARTESIAN_POINT('Ctrl Pts',(19.1394706686453,-9.29080659236423,-6.58244329214698));
#65933=CARTESIAN_POINT('Ctrl Pts',(19.2582757046255,-5.02169362206521,-10.219111507228));
#65934=CARTESIAN_POINT('Ctrl Pts',(19.3770807406058,0.465611034331595,-11.3767681349212));
#65935=CARTESIAN_POINT('Ctrl Pts',(19.495885776586,5.83996505421686,-9.77458208807802));
#65936=CARTESIAN_POINT('Ctrl Pts',(19.6146908125662,9.79762633823136,-5.80122098936464));
#65937=CARTESIAN_POINT('Ctrl Pts',(19.7334958485464,11.3785223619596,-0.420565915684839));
#65938=CARTESIAN_POINT('Ctrl Pts',(19.8523008845267,10.1991501605395,5.0621124872742));
#65939=CARTESIAN_POINT('Ctrl Pts',(19.9711059205069,6.5456087114698,9.31679416040626));
#65940=CARTESIAN_POINT('Ctrl Pts',(20.0899109564871,1.30419537835593,11.3113536434029));
#65941=CARTESIAN_POINT('Ctrl Pts',(20.2087159924674,-4.25359726551069,10.5619390802016));
#65942=CARTESIAN_POINT('Ctrl Pts',(20.3275210284476,-8.77952751098542,7.25034782027039));
#65943=CARTESIAN_POINT('Ctrl Pts',(20.4463260644278,-11.17566883928,2.17992495875334));
#65944=CARTESIAN_POINT('Ctrl Pts',(20.565131100408,-10.8607513314137,-3.41931679553761));
#65945=CARTESIAN_POINT('Ctrl Pts',(20.6839361363883,-7.91116951058155,-8.18908076684401));
#65946=CARTESIAN_POINT('Ctrl Pts',(20.8027411723685,-3.04245011378217,-10.9722898310333));
#65947=CARTESIAN_POINT('Ctrl Pts',(20.9215462083487,2.56432455140143,-11.0937769233985));
#65948=CARTESIAN_POINT('Ctrl Pts',(21.0403512443289,7.54903043181337,-8.5240709975108));
#65949=CARTESIAN_POINT('Ctrl Pts',(21.1591562803092,10.7024485431495,-3.88654628330681));
#65950=CARTESIAN_POINT('Ctrl Pts',(21.2779613162894,11.2596043538812,1.69379946425435));
#65951=CARTESIAN_POINT('Ctrl Pts',(21.3967663522696,9.08533976246439,6.86325347278047));
#65952=CARTESIAN_POINT('Ctrl Pts',(21.5155713882499,4.70710053679739,10.3677794810428));
#65953=CARTESIAN_POINT('Ctrl Pts',(21.6343764242301,-0.813014552095728,
11.3572291589599));
#65954=CARTESIAN_POINT('Ctrl Pts',(21.7531814602103,-6.13590383579682,9.59157604092798));
#65955=CARTESIAN_POINT('Ctrl Pts',(21.8719864961906,-9.97030983039016,5.49914254380397));
#65956=CARTESIAN_POINT('Ctrl Pts',(21.9907915321708,-11.3860599974293,0.0726950203974673));
#65957=CARTESIAN_POINT('Ctrl Pts',(22.109596568151,-10.0397134158073,-5.37138728444609));
#65958=CARTESIAN_POINT('Ctrl Pts',(22.2284016041312,-6.25787468066144,-9.51244717789204));
#65959=CARTESIAN_POINT('Ctrl Pts',(22.3472066401115,-0.957964258480223,
-11.3459222327021));
#65960=CARTESIAN_POINT('Ctrl Pts',(22.4660116760917,4.57433471288123,-10.4270373915883));
#65961=CARTESIAN_POINT('Ctrl Pts',(22.5848167120719,8.99696492783447,-6.9787010910603));
#65962=CARTESIAN_POINT('Ctrl Pts',(22.7036217480521,11.2370589906332,-1.83743083463828));
#65963=CARTESIAN_POINT('Ctrl Pts',(22.8224267840324,10.7512018368084,3.74957409518175));
#65964=CARTESIAN_POINT('Ctrl Pts',(22.9412318200126,7.65725552445528,8.42698550279093));
#65965=CARTESIAN_POINT('Ctrl Pts',(23.0600368559928,2.70576756973069,11.0601296868366));
#65966=CARTESIAN_POINT('Ctrl Pts',(23.178841891973,-2.9021012409417,11.0102431952421));
#65967=CARTESIAN_POINT('Ctrl Pts',(23.2976469279533,-7.80596143022092,8.28942778368647));
#65968=CARTESIAN_POINT('Ctrl Pts',(23.4164519639335,-10.8162060324177,3.55771470122882));
#65969=CARTESIAN_POINT('Ctrl Pts',(23.5352569999137,-11.2025923797191,-2.03704953423052));
#65970=CARTESIAN_POINT('Ctrl Pts',(23.6540620358939,-8.87138862161232,-7.13765442952913));
#65971=CARTESIAN_POINT('Ctrl Pts',(23.7728670718742,-4.3881117430937,-10.5067655423147));
#65972=CARTESIAN_POINT('Ctrl Pts',(23.8916721078544,1.15965883922563,-11.3270842765319));
#65973=CARTESIAN_POINT('Ctrl Pts',(24.0104771438346,6.42611262626162,-9.3996129359485));
#65974=CARTESIAN_POINT('Ctrl Pts',(24.1292821798149,10.1336825855701,-5.19192874430711));
#65975=CARTESIAN_POINT('Ctrl Pts',(24.2480872157951,11.3829648028602,0.275243760865819));
#65976=CARTESIAN_POINT('Ctrl Pts',(24.3668922517753,9.87090112181471,5.67564603145818));
#65977=CARTESIAN_POINT('Ctrl Pts',(24.4856972877555,5.9642967567156,9.69921703174444));
#65978=CARTESIAN_POINT('Ctrl Pts',(24.6045023237358,0.610838547223132,11.3698954744657));
#65979=CARTESIAN_POINT('Ctrl Pts',(24.723307359716,-4.89080043468954,10.2823984526515));
#65980=CARTESIAN_POINT('Ctrl Pts',(24.8421123956962,-9.2060005622438,6.700537327634));
#65981=CARTESIAN_POINT('Ctrl Pts',(24.9609174316765,-11.287955455987,1.49322083253071));
#65982=CARTESIAN_POINT('Ctrl Pts',(25.0797224676567,-10.6316123721108,-4.07632986891764));
#65983=CARTESIAN_POINT('Ctrl Pts',(25.198527503637,-7.39619083856349,-8.65702072947726));
#65984=CARTESIAN_POINT('Ctrl Pts',(25.3173325396171,-2.36655825463655,-11.1376410814167));
#65985=CARTESIAN_POINT('Ctrl Pts',(25.4361375755974,3.23716781396592,-10.9164275921783));
#65986=CARTESIAN_POINT('Ctrl Pts',(25.5549426115776,8.05560286040231,-8.04704351836921));
#65987=CARTESIAN_POINT('Ctrl Pts',(25.6737476475578,10.9198628476658,-3.22556076042874));
#65988=CARTESIAN_POINT('Ctrl Pts',(25.792552683538,11.1351189060748,2.37839731302918));
#65989=CARTESIAN_POINT('Ctrl Pts',(25.9113577195183,8.64915296729008,7.40538991407386));
#65990=CARTESIAN_POINT('Ctrl Pts',(26.0301627554985,4.06502512745981,10.6359398994245));
#65991=CARTESIAN_POINT('Ctrl Pts',(26.1489677914787,-1.50522018323548,11.2863616383239));
#65992=CARTESIAN_POINT('Ctrl Pts',(26.267772827459,-6.71032041520536,9.19887203717542));
#65993=CARTESIAN_POINT('Ctrl Pts',(26.3865778634392,-10.2875920387279,4.87986648134475));
#65994=CARTESIAN_POINT('Ctrl Pts',(26.5053828994194,-11.3692396686883,-0.622925506760649));
#65995=CARTESIAN_POINT('Ctrl Pts',(26.6241879353996,-9.6928709232983,-5.97460459740457));
#65996=CARTESIAN_POINT('Ctrl Pts',(26.7429929713799,-5.66514909629104,-9.87692930762605));
#65997=CARTESIAN_POINT('Ctrl Pts',(26.8617980073601,-0.263142406646583,
-11.3832509813706));
#65998=CARTESIAN_POINT('Ctrl Pts',(26.9806030433403,5.20269890059145,-10.1281573339297));
#65999=CARTESIAN_POINT('Ctrl Pts',(27.0994080793206,9.40643920705916,-6.41611629219342));
#66000=CARTESIAN_POINT('Ctrl Pts',(27.2182131153008,11.3283107058654,-1.14761639166837));
#66001=CARTESIAN_POINT('Ctrl Pts',(27.337018151281,10.5020946155004,4.3992789770742));
#66002=CARTESIAN_POINT('Ctrl Pts',(27.4558231872612,7.12821924719783,8.87897162935709));
#66003=CARTESIAN_POINT('Ctrl Pts',(27.5746282232415,2.0251389378644,11.2047516310445));
#66004=CARTESIAN_POINT('Ctrl Pts',(27.6934332592217,-3.56921136979376,10.8124177235614));
#66005=CARTESIAN_POINT('Ctrl Pts',(27.812238295202,-8.29772159563105,7.79714455120897));
#66006=CARTESIAN_POINT('Ctrl Pts',(27.9310433311821,-11.0133221893601,2.89039464163601));
#66007=CARTESIAN_POINT('Ctrl Pts',(28.0498483671624,-11.0572469428023,-2.71752403428923));
#66008=CARTESIAN_POINT('Ctrl Pts',(28.1686534031426,-8.41884033344178,-7.66620990262223));
#66009=CARTESIAN_POINT('Ctrl Pts',(28.2874584391229,-3.73814240313741,-10.7551819233761));
#66010=CARTESIAN_POINT('Ctrl Pts',(28.406263475103,1.84937588294144,-11.2350992730213));
#66011=CARTESIAN_POINT('Ctrl Pts',(28.5250685110833,6.98826179623471,-8.98954080575508));
#66012=CARTESIAN_POINT('Ctrl Pts',(28.6438735470635,10.4318944620895,-4.56324717310783));
#66013=CARTESIAN_POINT('Ctrl Pts',(28.7626785830438,11.3448974120795,0.970025535973534));
#66014=CARTESIAN_POINT('Ctrl Pts',(28.881483619024,9.50578907310103,6.26798380093333));
#66015=CARTESIAN_POINT('Ctrl Pts',(29.0002886550042,5.3607110573249,10.0454180495848));
#66016=CARTESIAN_POINT('Ctrl Pts',(29.1190936909844,-0.0847994684935192,
11.3859762814259));
#66017=CARTESIAN_POINT('Ctrl Pts',(29.2378987269646,-5.50973884535723,9.96445807292153));
#66018=CARTESIAN_POINT('Ctrl Pts',(29.3567037629449,-9.59809368339291,6.12570359027135));
#66019=CARTESIAN_POINT('Ctrl Pts',(29.4755087989251,-11.3580870546674,0.80094025348108));
#66020=CARTESIAN_POINT('Ctrl Pts',(29.5943138349054,-10.3627695166555,-4.7181198348204));
#66021=CARTESIAN_POINT('Ctrl Pts',(29.7131188708855,-6.85359099463842,-9.09263093440294));
#66022=CARTESIAN_POINT('Ctrl Pts',(29.8319239068658,-1.68182845258121,-11.2613986647813));
#66023=CARTESIAN_POINT('Ctrl Pts',(29.950728942846,3.8979218307779,-10.6983107186225));
#66024=CARTESIAN_POINT('Ctrl Pts',(30.0695339788262,8.53209153422109,-7.53996424943265));
#66025=CARTESIAN_POINT('Ctrl Pts',(30.1883390148065,11.0964967808398,-2.55252933849185));
#66026=CARTESIAN_POINT('Ctrl Pts',(30.3071440507867,10.9690492103465,3.05411300577552));
#66027=CARTESIAN_POINT('Ctrl Pts',(30.425949086767,8.18066579666925,7.91987082939201));
#66028=CARTESIAN_POINT('Ctrl Pts',(30.5447541227472,3.40776882835034,10.8643802604462));
#66029=CARTESIAN_POINT('Ctrl Pts',(30.6635591587274,-2.19180454981553,11.1733450517944));
#66030=CARTESIAN_POINT('Ctrl Pts',(30.7823641947076,-7.25967721481869,8.77181472488401));
#66031=CARTESIAN_POINT('Ctrl Pts',(30.9011692306878,-10.5664550993703,4.24236649336666));
#66032=CARTESIAN_POINT('Ctrl Pts',(31.0199742666681,-11.3099607649601,-1.31621971042573));
#66033=CARTESIAN_POINT('Ctrl Pts',(31.1387793026483,-9.3098302769169,-6.55550967096015));
#66034=CARTESIAN_POINT('Ctrl Pts',(31.2575843386285,-5.05126693815397,-10.2045259150321));
#66035=CARTESIAN_POINT('Ctrl Pts',(31.3763893746087,0.432662153963747,-11.3780688296203));
#66036=CARTESIAN_POINT('Ctrl Pts',(31.495194410589,5.81163354086987,-9.79145353957655));
#66037=CARTESIAN_POINT('Ctrl Pts',(31.6139994465692,9.78078501542091,-5.82957042269564));
#66038=CARTESIAN_POINT('Ctrl Pts',(31.7328044825494,11.3772566958599,-0.45351616019857));
#66039=CARTESIAN_POINT('Ctrl Pts',(31.8516095185297,10.2137671838044,5.03255469379998));
#66040=CARTESIAN_POINT('Ctrl Pts',(31.9704145545099,6.57256254146375,9.29779911966252));
#66041=CARTESIAN_POINT('Ctrl Pts',(32.0892195904901,1.33694739801475,11.307529283004));
#66042=CARTESIAN_POINT('Ctrl Pts',(32.2080246264704,-4.22299223186951,10.5742131357666));
#66043=CARTESIAN_POINT('Ctrl Pts',(32.3268296624505,-8.75849381067178,7.27574277991417));
#66044=CARTESIAN_POINT('Ctrl Pts',(32.4456346984308,-11.1693089498201,2.21228036526069));
#66045=CARTESIAN_POINT('Ctrl Pts',(32.564439734411,-10.8706080718339,-3.38784990512113));
#66046=CARTESIAN_POINT('Ctrl Pts',(32.6832447703913,-7.93485177538323,-8.16613581406452));
#66047=CARTESIAN_POINT('Ctrl Pts',(32.8020498063715,-3.07421292123998,-10.9634329361715));
#66048=CARTESIAN_POINT('Ctrl Pts',(32.9208548423517,2.53218640811296,-11.1011566435943));
#66049=CARTESIAN_POINT('Ctrl Pts',(33.0396598783319,7.52431321067168,-8.54589711725819));
#66050=CARTESIAN_POINT('Ctrl Pts',(33.1584649143122,10.6911482916167,-3.91752409535808));
#66051=CARTESIAN_POINT('Ctrl Pts',(33.2772699502924,11.2644623527887,1.66118473796684));
#66052=CARTESIAN_POINT('Ctrl Pts',(33.3960749862726,9.10517753014351,6.83691370251369));
#66053=CARTESIAN_POINT('Ctrl Pts',(33.5148800222529,4.73710571202568,10.3541043216757));
#66054=CARTESIAN_POINT('Ctrl Pts',(33.6336850582331,-0.780120799480794,
11.3595360102984));
#66055=CARTESIAN_POINT('Ctrl Pts',(33.7524900942133,-6.10810106388364,9.60930529353878));
#66056=CARTESIAN_POINT('Ctrl Pts',(33.8712951301936,-9.9543425975179,5.52799333233048));
#66057=CARTESIAN_POINT('Ctrl Pts',(33.9901001661737,-11.3858017279442,0.105668552526543));
#66058=CARTESIAN_POINT('Ctrl Pts',(34.108905202154,-10.0552267622252,-5.34228992018216));
#66059=CARTESIAN_POINT('Ctrl Pts',(34.2277102381342,-6.2853963250558,-9.49428458958461));
#66060=CARTESIAN_POINT('Ctrl Pts',(34.3465152741144,-0.990817840062839,
-11.3431004068051));
#66061=CARTESIAN_POINT('Ctrl Pts',(34.4653203100947,4.54411900727605,-10.4402408630626));
#66062=CARTESIAN_POINT('Ctrl Pts',(34.5841253460749,8.97671700005413,-7.00472688489628));
#66063=CARTESIAN_POINT('Ctrl Pts',(34.7029303820551,11.2316907009262,-1.86996546218826));
#66064=CARTESIAN_POINT('Ctrl Pts',(34.8217354180354,10.7620154561579,3.71842307335641));
#66065=CARTESIAN_POINT('Ctrl Pts',(34.9405404540156,7.6816278220989,8.40477488299397));
#66066=CARTESIAN_POINT('Ctrl Pts',(35.0593454899958,2.73778617175729,11.0522474505769));
#66067=CARTESIAN_POINT('Ctrl Pts',(35.178150525976,-2.87020359349378,11.0186014612992));
#66068=CARTESIAN_POINT('Ctrl Pts',(35.2969555619563,-7.78192265444729,8.31199895520023));
#66069=CARTESIAN_POINT('Ctrl Pts',(35.4157605979365,-10.8058575945519,3.58902333195472));
#66070=CARTESIAN_POINT('Ctrl Pts',(35.5345656339167,-11.2084446640896,-2.00459847428116));
#66071=CARTESIAN_POINT('Ctrl Pts',(35.6533706698969,-8.89202194699182,-7.11193310747962));
#66072=CARTESIAN_POINT('Ctrl Pts',(35.7721757058772,-4.41852075723942,-10.4940135862736));
#66073=CARTESIAN_POINT('Ctrl Pts',(35.8909807418574,1.12685093207293,-11.3303951302652));
#66074=CARTESIAN_POINT('Ctrl Pts',(36.0097857778376,6.39886455929819,-9.41818343327454));
#66075=CARTESIAN_POINT('Ctrl Pts',(36.1285908138179,10.1186043535776,-5.22125394582665));
#66076=CARTESIAN_POINT('Ctrl Pts',(36.247395849798,11.3837141711737,0.242277733332544));
#66077=CARTESIAN_POINT('Ctrl Pts',(36.3662008857784,9.88729630430444,5.64703626887032));
#66078=CARTESIAN_POINT('Ctrl Pts',(36.4850059217585,5.99236051452477,9.6819038569392));
#66079=CARTESIAN_POINT('Ctrl Pts',(36.6038109577388,0.643763010533854,11.3680788182225));
#66080=CARTESIAN_POINT('Ctrl Pts',(36.722615993719,-4.86100227394527,10.2965190100222));
#66081=CARTESIAN_POINT('Ctrl Pts',(36.8414210296992,-9.18655731544908,6.72716965157099));
#66082=CARTESIAN_POINT('Ctrl Pts',(36.9602260656795,-11.2835837791904,1.52590429878194));
#66083=CARTESIAN_POINT('Ctrl Pts',(37.0790311016597,-10.6433727721311,-4.04552380594999));
#66084=CARTESIAN_POINT('Ctrl Pts',(37.1978361376399,-7.42123040906898,-8.63556518396795));
#66085=CARTESIAN_POINT('Ctrl Pts',(37.3166411736201,-2.39880275077906,-11.1307408645563));
#66086=CARTESIAN_POINT('Ctrl Pts',(37.4354462096004,3.20554044985842,-10.9257565987611));
#66087=CARTESIAN_POINT('Ctrl Pts',(37.5542512455806,8.03226497851866,-8.07033866364434));
#66088=CARTESIAN_POINT('Ctrl Pts',(37.6730562815608,10.9104758873174,-3.25717097238022));
#66089=CARTESIAN_POINT('Ctrl Pts',(37.791861317541,11.1419600107742,2.34614022372005));
#66090=CARTESIAN_POINT('Ctrl Pts',(37.9106663535213,8.6705625820156,7.38031106000288));
#66091=CARTESIAN_POINT('Ctrl Pts',(38.0294713895015,4.09580958317776,10.6241230550761));
#66092=CARTESIAN_POINT('Ctrl Pts',(38.1482764254818,-1.47252875908745,11.2906734026235));
#66093=CARTESIAN_POINT('Ctrl Pts',(38.2670814614619,-6.68365249869776,9.21826643722669));
#66094=CARTESIAN_POINT('Ctrl Pts',(38.3858864974422,-10.273416888366,4.90963871062686));
#66095=CARTESIAN_POINT('Ctrl Pts',(38.5046915334224,-11.3709959750056,-0.589997769025954));
#66096=CARTESIAN_POINT('Ctrl Pts',(38.6234965694026,-9.7101326312792,-5.94650915361411));
#66097=CARTESIAN_POINT('Ctrl Pts',(38.7423016053828,-5.69372876027827,-9.86048171416736));
#66098=CARTESIAN_POINT('Ctrl Pts',(38.8611066413631,-0.296107005297001,
-11.3824411912587));
#66099=CARTESIAN_POINT('Ctrl Pts',(38.9799116773433,5.17334611161038,-10.1431817907664));
#66100=CARTESIAN_POINT('Ctrl Pts',(39.0987167133236,9.38781879825448,-6.443330275734));
#66101=CARTESIAN_POINT('Ctrl Pts',(39.2175217493038,11.3249397244533,-1.18041817528639));
#66102=CARTESIAN_POINT('Ctrl Pts',(39.336326785284,10.5147908137855,4.36884664109223));
#66103=CARTESIAN_POINT('Ctrl Pts',(39.4551318212642,7.15390270745462,8.85829119431749));
#66104=CARTESIAN_POINT('Ctrl Pts',(39.5739368572445,2.05757921671945,11.1988398773252));
#66105=CARTESIAN_POINT('Ctrl Pts',(39.6927418932247,-3.53788382412481,10.8227087588117));
#66106=CARTESIAN_POINT('Ctrl Pts',(39.8115469292049,-8.27510640163055,7.82114191615929));
#66107=CARTESIAN_POINT('Ctrl Pts',(39.9303519651852,-11.0049054725103,2.92227691573508));
#66108=CARTESIAN_POINT('Ctrl Pts',(40.0491570011653,-11.0650704792844,-2.68549103878735));
#66109=CARTESIAN_POINT('Ctrl Pts',(40.1679620371457,-8.44100624423463,-7.64179693631913));
#66110=CARTESIAN_POINT('Ctrl Pts',(40.2867670731258,-3.76927355245578,-10.7443112258486));
#66111=CARTESIAN_POINT('Ctrl Pts',(40.4055721091061,1.81683147052239,-11.2404079213395));
#66112=CARTESIAN_POINT('Ctrl Pts',(40.5243771450863,6.96219893399887,-9.00974099718607));
#66113=CARTESIAN_POINT('Ctrl Pts',(40.6431821810665,10.4186356306152,-4.59343862738167));
#66114=CARTESIAN_POINT('Ctrl Pts',(40.7619872170467,11.3476590165799,0.937166837321403));
#66115=CARTESIAN_POINT('Ctrl Pts',(40.880792253027,9.52390118621212,6.24042891308052));
#66116=CARTESIAN_POINT('Ctrl Pts',(40.9995972890072,5.38977993959484,10.0298513963906));
#66117=CARTESIAN_POINT('Ctrl Pts',(41.1184023249874,-0.0518255205332239,
11.386174114837));
#66118=CARTESIAN_POINT('Ctrl Pts',(41.2372073609677,-5.48085883495741,9.98037239642597));
#66119=CARTESIAN_POINT('Ctrl Pts',(41.3560123969479,-9.58031350924652,6.15347382411363));
#66120=CARTESIAN_POINT('Ctrl Pts',(41.4748174329281,-11.3557199010282,0.833829714185648));
#66121=CARTESIAN_POINT('Ctrl Pts',(41.5936224689083,-10.3763896870325,-4.68808962860982));
#66122=CARTESIAN_POINT('Ctrl Pts',(41.7124275048886,-6.87989430203223,-9.07274495375211));
#66123=CARTESIAN_POINT('Ctrl Pts',(41.8312325408687,-1.71443433239213,-11.2564808338679));
#66124=CARTESIAN_POINT('Ctrl Pts',(41.9500375768491,3.86692357599851,-10.7095542901733));
#66125=CARTESIAN_POINT('Ctrl Pts',(42.0688426128291,8.51021972726088,-7.56464119643434));
#66126=CARTESIAN_POINT('Ctrl Pts',(42.1876476488096,11.0890589788854,-2.58465434171604));
#66127=CARTESIAN_POINT('Ctrl Pts',(42.3064526847897,10.9778463046305,3.02233486841273));
#66128=CARTESIAN_POINT('Ctrl Pts',(42.4252577207699,8.20357033379128,7.89614490553161));
#66129=CARTESIAN_POINT('Ctrl Pts',(42.5440627567502,3.43921174510382,10.8544690365879));
#66130=CARTESIAN_POINT('Ctrl Pts',(42.6628677927304,-2.1594262281051,11.1796394910844));
#66131=CARTESIAN_POINT('Ctrl Pts',(42.7816728287106,-7.23426560498598,8.79281369989061));
#66132=CARTESIAN_POINT('Ctrl Pts',(42.9004778646909,-10.5540827250195,4.27292606530414));
#66133=CARTESIAN_POINT('Ctrl Pts',(43.019282900671,-11.3138067629015,-1.2834164233872));
#66134=CARTESIAN_POINT('Ctrl Pts',(43.1380879366513,-9.3286175996306,-6.52860706125067));
#66135=CARTESIAN_POINT('Ctrl Pts',(43.2568929726315,-5.08110823047943,-10.1896850382358));
#66136=CARTESIAN_POINT('Ctrl Pts',(43.3756980086117,0.400352765770355,-11.3796362602292));
#66137=CARTESIAN_POINT('Ctrl Pts',(43.4549013659319,3.98785181636839,-10.3313646489034));
#66138=CARTESIAN_POINT('Ctrl Pts',(43.494503044592,5.54895898246599,-9.41088599980616));
#66139=CARTESIAN_POINT('',(0.724999999999993,-5.84323637812456,-8.19946832906633));
#66140=CARTESIAN_POINT('Ctrl Pts',(0.724999999999994,-5.84362420709187,
-8.19964058298314));
#66141=CARTESIAN_POINT('Ctrl Pts',(0.724999999999994,-6.05459248715557,
-8.06228587138525));
#66142=CARTESIAN_POINT('Ctrl Pts',(0.724999999999993,-6.26011272811705,
-7.91716467428617));
#66143=CARTESIAN_POINT('Ctrl Pts',(0.724999999999993,-6.4597129648342,-7.76452859810948));
#66144=CARTESIAN_POINT('Ctrl Pts',(0.724999999999993,-6.47926405855697,
-7.74957770286061));
#66145=CARTESIAN_POINT('Ctrl Pts',(0.724999999999994,-6.49875833816115,
-7.73455466802475));
#66146=CARTESIAN_POINT('Ctrl Pts',(0.724999999999994,-6.51819534971905,
-7.71945970526014));
#66147=CARTESIAN_POINT('Ctrl Pts',(0.724999999999994,-6.71529186459291,
-7.56639273073105));
#66148=CARTESIAN_POINT('Ctrl Pts',(0.724999999999993,-6.90650209024528,
-7.40593351388788));
#66149=CARTESIAN_POINT('Ctrl Pts',(0.724999999999994,-7.09155771173187,
-7.23853845120389));
#66150=CARTESIAN_POINT('Ctrl Pts',(0.724999999999994,-7.22536229604805,
-7.11750334511479));
#66151=CARTESIAN_POINT('Ctrl Pts',(0.724999999999994,-7.35594873254017,
-6.9928411360138));
#66152=CARTESIAN_POINT('Ctrl Pts',(0.724999999999994,-7.48320550323649,
-6.86471075727357));
#66153=CARTESIAN_POINT('Ctrl Pts',(0.724999999999994,-7.55090721007478,
-6.79654428337136));
#66154=CARTESIAN_POINT('Ctrl Pts',(0.724999999999993,-7.61766635790337,
-6.72739602064615));
#66155=CARTESIAN_POINT('Ctrl Pts',(0.724999999999993,-7.68346504003637,
-6.6572887440922));
#66156=CARTESIAN_POINT('Ctrl Pts',(0.724999999999993,-7.71711063119756,
-6.62143999016745));
#66157=CARTESIAN_POINT('Ctrl Pts',(0.724999999999994,-7.75050507634197,
-6.58534047055983));
#66158=CARTESIAN_POINT('Ctrl Pts',(0.724999999999994,-7.78364589711456,
-6.54899315593021));
#66159=CARTESIAN_POINT('Ctrl Pts',(0.724999999999994,-7.81268828291639,
-6.51714081462649));
#66160=CARTESIAN_POINT('Ctrl Pts',(0.724999999999993,-7.84153824136138,
-6.48509543714251));
#66161=CARTESIAN_POINT('Ctrl Pts',(0.724999999999993,-7.87017661171247,
-6.45287892646051));
#66162=CARTESIAN_POINT('Ctrl Pts',(0.724999999999993,-8.03763596799428,
-6.26449683368372));
#66163=CARTESIAN_POINT('Ctrl Pts',(0.724999999999993,-8.19798163435683,
-6.07013933040428));
#66164=CARTESIAN_POINT('Ctrl Pts',(0.724999999999993,-8.35094787320371,
-5.87027275961279));
#66165=CARTESIAN_POINT('Ctrl Pts',(0.724999999999993,-8.50503312400608,
-5.66894408133991));
#66166=CARTESIAN_POINT('Ctrl Pts',(0.724999999999994,-8.65163104540178,
-5.46202498011212));
#66167=CARTESIAN_POINT('Ctrl Pts',(0.724999999999993,-8.79043530712676,
-5.24995266825496));
#66168=CARTESIAN_POINT('Ctrl Pts',(0.724999999999993,-8.92881462569918,
-5.03852960646875));
#66169=CARTESIAN_POINT('Ctrl Pts',(0.724999999999994,-9.05944833941144,
-4.82198431992977));
#66170=CARTESIAN_POINT('Ctrl Pts',(0.724999999999994,-9.18199212058087,
-4.60071839213501));
#66171=CARTESIAN_POINT('Ctrl Pts',(0.724999999999994,-9.22706211498565,
-4.51933968786695));
#66172=CARTESIAN_POINT('Ctrl Pts',(0.724999999999994,-9.27103737759854,
-4.43732216559539));
#66173=CARTESIAN_POINT('Ctrl Pts',(0.724999999999994,-9.31389921338204,
-4.35468493648143));
#66174=CARTESIAN_POINT('Ctrl Pts',(0.724999999999994,-9.32639788476886,
-4.33058761185376));
#66175=CARTESIAN_POINT('Ctrl Pts',(0.724999999999993,-9.33880080596761,
-4.30643959406877));
#66176=CARTESIAN_POINT('Ctrl Pts',(0.724999999999993,-9.35110356217466,
-4.28224936887147));
#66177=CARTESIAN_POINT('Ctrl Pts',(0.724999999999993,-9.44079116130515,
-4.10590163151419));
#66178=CARTESIAN_POINT('Ctrl Pts',(0.724999999999994,-9.52521914037613,
-3.92719166007731));
#66179=CARTESIAN_POINT('Ctrl Pts',(0.724999999999994,-9.60426374701328,
-3.7463347748938));
#66180=CARTESIAN_POINT('Ctrl Pts',(0.724999999999994,-9.70511183645256,
-3.51559074176297));
#66181=CARTESIAN_POINT('Ctrl Pts',(0.724999999999993,-9.79719891971918,
-3.28135288395628));
#66182=CARTESIAN_POINT('Ctrl Pts',(0.724999999999993,-9.88054543068308,
-3.04415886228902));
#66183=CARTESIAN_POINT('Ctrl Pts',(0.724999999999993,-9.96480898230241,
-2.8043550545782));
#66184=CARTESIAN_POINT('Ctrl Pts',(0.724999999999994,-10.0401387660408,
-2.56152911069881));
#66185=CARTESIAN_POINT('Ctrl Pts',(0.724999999999993,-10.1065096789136,
-2.31620930938537));
#66186=CARTESIAN_POINT('Ctrl Pts',(0.724999999999993,-10.1731973459982,
-2.06971872290517));
#66187=CARTESIAN_POINT('Ctrl Pts',(0.724999999999994,-10.230840598825,-1.82070980135915));
#66188=CARTESIAN_POINT('Ctrl Pts',(0.724999999999994,-10.2793647960243,
-1.56969994651305));
#66189=CARTESIAN_POINT('Ctrl Pts',(0.724999999999994,-10.3252045541866,
-1.33257637298439));
#66190=CARTESIAN_POINT('Ctrl Pts',(0.724999999999994,-10.3629060199728,
-1.09366653348239));
#66191=CARTESIAN_POINT('Ctrl Pts',(0.724999999999994,-10.3923641605725,
-0.85339914527474));
#66192=CARTESIAN_POINT('Ctrl Pts',(0.724999999999994,-10.4034109632973,
-0.763298874696871));
#66193=CARTESIAN_POINT('Ctrl Pts',(0.724999999999994,-10.4132981275469,
-0.673007664148894));
#66194=CARTESIAN_POINT('Ctrl Pts',(0.724999999999994,-10.4220185799031,
-0.582548077174242));
#66195=CARTESIAN_POINT('Ctrl Pts',(0.724999999999994,-10.4248219014662,
-0.553468472081048));
#66196=CARTESIAN_POINT('Ctrl Pts',(0.724999999999994,-10.4275046486325,
-0.524371467242655));
#66197=CARTESIAN_POINT('Ctrl Pts',(0.724999999999994,-10.4300665676683,
-0.495257813240309));
#66198=CARTESIAN_POINT('Ctrl Pts',(0.724999999999994,-10.4325653520722,
-0.466861621345176));
#66199=CARTESIAN_POINT('Ctrl Pts',(0.724999999999994,-10.4349484725205,
-0.438457592267791));
#66200=CARTESIAN_POINT('Ctrl Pts',(0.724999999999994,-10.4372155250113,
-0.410051402805783));
#66201=CARTESIAN_POINT('Ctrl Pts',(0.724999999999994,-10.4577567710926,
-0.15266939232543));
#66202=CARTESIAN_POINT('Ctrl Pts',(0.724999999999994,-10.4687845119503,
0.105017586375021));
#66203=CARTESIAN_POINT('Ctrl Pts',(0.724999999999994,-10.4702959390391,
0.362470394026527));
#66204=CARTESIAN_POINT('Ctrl Pts',(0.724999999999994,-10.4718149618008,
0.621217030100876));
#66205=CARTESIAN_POINT('Ctrl Pts',(0.724999999999993,-10.4637219392879,
0.879727772197104));
#66206=CARTESIAN_POINT('Ctrl Pts',(0.724999999999993,-10.4459639413827,
1.13747054496583));
#66207=CARTESIAN_POINT('Ctrl Pts',(0.724999999999993,-10.4418041705112,
1.19784620691876));
#66208=CARTESIAN_POINT('Ctrl Pts',(0.724999999999994,-10.4371138417348,
1.25817977071446));
#66209=CARTESIAN_POINT('Ctrl Pts',(0.724999999999994,-10.4318918655191,
1.31846445863066));
#66210=CARTESIAN_POINT('Ctrl Pts',(0.724999999999994,-10.4097057147322,
1.57459070681758));
#66211=CARTESIAN_POINT('Ctrl Pts',(0.724999999999993,-10.3779271422183,
1.82983479584259));
#66212=CARTESIAN_POINT('Ctrl Pts',(0.724999999999993,-10.3367810724392,
2.08371653173242));
#66213=CARTESIAN_POINT('Ctrl Pts',(0.724999999999993,-10.2954668803757,
2.33863562496042));
#66214=CARTESIAN_POINT('Ctrl Pts',(0.724999999999993,-10.244708341432,2.59218183014901));
#66215=CARTESIAN_POINT('Ctrl Pts',(0.724999999999993,-10.1846808988108,
2.84386269118601));
#66216=CARTESIAN_POINT('Ctrl Pts',(0.724999999999993,-10.1485099935167,
2.99551873701108));
#66217=CARTESIAN_POINT('Ctrl Pts',(0.724999999999994,-10.1089726084179,
3.1464973237586));
#66218=CARTESIAN_POINT('Ctrl Pts',(0.724999999999994,-10.0660983557501,
3.2966881458436));
#66219=CARTESIAN_POINT('Ctrl Pts',(0.724999999999994,-10.0447844817427,
3.37135179733125));
#66220=CARTESIAN_POINT('Ctrl Pts',(0.724999999999994,-10.0226458555074,
3.44582072890303));
#66221=CARTESIAN_POINT('Ctrl Pts',(0.724999999999994,-9.99968552784372,
3.52008113894002));
#66222=CARTESIAN_POINT('Ctrl Pts',(0.724999999999994,-9.99007798101697,
3.55115475327404));
#66223=CARTESIAN_POINT('Ctrl Pts',(0.724999999999994,-9.98032608318451,
3.58219316803561));
#66224=CARTESIAN_POINT('Ctrl Pts',(0.724999999999994,-9.97043650651514,
3.61317559496846));
#66225=CARTESIAN_POINT('Ctrl Pts',(0.724999999999994,-9.89111838036777,
3.86166631706605));
#66226=CARTESIAN_POINT('Ctrl Pts',(0.724999999999994,-9.80285909739519,
4.106848173817));
#66227=CARTESIAN_POINT('Ctrl Pts',(0.724999999999994,-9.70593507543463,
4.34824175812628));
#66228=CARTESIAN_POINT('Ctrl Pts',(0.724999999999994,-9.60844176596236,
4.59105317828449));
#66229=CARTESIAN_POINT('Ctrl Pts',(0.724999999999993,-9.50218147766871,
4.83003231917608));
#66230=CARTESIAN_POINT('Ctrl Pts',(0.724999999999993,-9.38738267911701,
5.064686430357));
#66231=CARTESIAN_POINT('Ctrl Pts',(0.724999999999993,-9.27278083222799,
5.29893796313176));
#66232=CARTESIAN_POINT('Ctrl Pts',(0.724999999999993,-9.14966953604564,
5.52887991404994));
#66233=CARTESIAN_POINT('Ctrl Pts',(0.724999999999993,-9.0182264279511,5.75400791175182));
#66234=CARTESIAN_POINT('Ctrl Pts',(0.724999999999993,-8.91834778786122,
5.92507415160708));
#66235=CARTESIAN_POINT('Ctrl Pts',(0.724999999999993,-8.81365741051102,
6.09336064383297));
#66236=CARTESIAN_POINT('Ctrl Pts',(0.724999999999993,-8.70421511552432,
6.25863727727093));
#66237=CARTESIAN_POINT('Ctrl Pts',(0.724999999999993,-8.56594004163737,
6.46745635131534));
#66238=CARTESIAN_POINT('Ctrl Pts',(0.724999999999994,-8.42008030880078,
6.67147181811569));
#66239=CARTESIAN_POINT('Ctrl Pts',(0.724999999999994,-8.26697046681593,
6.87038216935151));
#66240=CARTESIAN_POINT('Ctrl Pts',(0.724999999999994,-8.20955427607161,
6.94497355106494));
#66241=CARTESIAN_POINT('Ctrl Pts',(0.724999999999994,-8.15111819503291,
7.01884674205683));
#66242=CARTESIAN_POINT('Ctrl Pts',(0.724999999999994,-8.09167868745761,
7.09198475901793));
#66243=CARTESIAN_POINT('Ctrl Pts',(0.724999999999994,-8.0697669952949,7.1189462494208));
#66244=CARTESIAN_POINT('Ctrl Pts',(0.724999999999993,-8.04771893723002,
7.14580782762178));
#66245=CARTESIAN_POINT('Ctrl Pts',(0.724999999999993,-8.02553531777951,
7.17256862068183));
#66246=CARTESIAN_POINT('Ctrl Pts',(0.724999999999993,-8.00773648109852,
7.19403991332602));
#66247=CARTESIAN_POINT('Ctrl Pts',(0.724999999999993,-7.9898540090722,7.21544191375683));
#66248=CARTESIAN_POINT('Ctrl Pts',(0.724999999999993,-7.97189307755571,
7.2367688006789));
#66249=CARTESIAN_POINT('Ctrl Pts',(0.724999999999994,-7.80423370685344,
7.43584825472124));
#66250=CARTESIAN_POINT('Ctrl Pts',(0.724999999999994,-7.62961526028927,
7.62853692515369));
#66251=CARTESIAN_POINT('Ctrl Pts',(0.724999999999994,-7.44850865398731,
7.81456975312634));
#66252=CARTESIAN_POINT('Ctrl Pts',(0.724999999999993,-7.26476715322843,
8.00330914645981));
#66253=CARTESIAN_POINT('Ctrl Pts',(0.724999999999994,-7.0743469862355,8.18519809903005));
#66254=CARTESIAN_POINT('Ctrl Pts',(0.724999999999993,-6.87769284169641,
8.35993466078694));
#66255=CARTESIAN_POINT('Ctrl Pts',(0.724999999999993,-6.82338787478308,
8.40818720703761));
#66256=CARTESIAN_POINT('Ctrl Pts',(0.724999999999993,-6.7686072751131,8.45589417230036));
#66257=CARTESIAN_POINT('Ctrl Pts',(0.724999999999993,-6.71335984205473,
8.50304879018143));
#66258=CARTESIAN_POINT('Ctrl Pts',(0.724999999999994,-5.84362420709187,
-8.19964058298314));
#66259=CARTESIAN_POINT('Ctrl Pts',(0.75807074233972,-4.70712093344169,-9.0078742953982));
#66260=CARTESIAN_POINT('Ctrl Pts',(0.830743163339522,-1.83770484000176,
-10.2640347617308));
#66261=CARTESIAN_POINT('Ctrl Pts',(0.943017262999401,3.04159683638712,-10.0431701202702));
#66262=CARTESIAN_POINT('Ctrl Pts',(1.06182229897963,7.46688591750615,-7.37303115014316));
#66263=CARTESIAN_POINT('Ctrl Pts',(1.18062733495986,10.0808097748896,-2.91434903386085));
#66264=CARTESIAN_POINT('Ctrl Pts',(1.29943237094008,10.249274439043,2.25133856122268));
#66265=CARTESIAN_POINT('Ctrl Pts',(1.41823740692031,7.93140919765733,6.87087002708225));
#66266=CARTESIAN_POINT('Ctrl Pts',(1.53704244290054,3.68949714972476,9.82363271220668));
#66267=CARTESIAN_POINT('Ctrl Pts',(1.65584747888077,-1.44743493143616,10.3933177948697));
#66268=CARTESIAN_POINT('Ctrl Pts',(1.774652514861,-6.23323964791348,8.44173315899732));
#66269=CARTESIAN_POINT('Ctrl Pts',(1.88864091159203,-9.37422490179139,4.60444921031521));
#66270=CARTESIAN_POINT('Ctrl Pts',(1.96302762966299,-10.0677887342179,1.46660577231488));
#66271=CARTESIAN_POINT('Ctrl Pts',(1.99781266907388,-10.0690473037901,-0.000187867633422503));
#66272=CARTESIAN_POINT('Ctrl Pts',(42.9923131746348,-10.9250461896976,-0.000265489735796583));
#66273=CARTESIAN_POINT('Ctrl Pts',(42.9948754497565,-10.9251662217889,-0.117518583538486));
#66274=CARTESIAN_POINT('Ctrl Pts',(42.9974377248782,-10.9234003795194,-0.234768005463963));
#66275=CARTESIAN_POINT('Ctrl Pts',(43.,-10.9197403196571,-0.351952921252015));
#66276=CARTESIAN_POINT('Ctrl Pts',(0.724999999999993,-4.12761311060678,
-9.09590817756005));
#66277=CARTESIAN_POINT('Ctrl Pts',(0.724999999999993,-5.07083433738308,
-8.71410438480677));
#66278=CARTESIAN_POINT('Ctrl Pts',(0.724999999999994,-7.71164281680344,
-7.15328739647488));
#66279=CARTESIAN_POINT('Ctrl Pts',(0.724999999999994,-10.6476594428495,
-2.69915475322739));
#66280=CARTESIAN_POINT('Ctrl Pts',(0.724999999999993,-10.5832508201471,
3.68636503788138));
#66281=CARTESIAN_POINT('Ctrl Pts',(0.724999999999994,-8.23383227269803,
7.20734712971691));
#66282=CARTESIAN_POINT('Ctrl Pts',(0.724999999999994,-6.71403705763906,
8.50428280208053));
#66283=CARTESIAN_POINT('Ctrl Pts',(0.54021611338146,-4.16673338810089,-9.1739436324887));
#66284=CARTESIAN_POINT('Ctrl Pts',(0.542188125511685,-5.11480475354192,
-8.78060130055235));
#66285=CARTESIAN_POINT('Ctrl Pts',(0.549829057165572,-7.76158824171289,
-7.18547782947134));
#66286=CARTESIAN_POINT('Ctrl Pts',(0.56972870387115,-10.6718612335829,-2.69120359150766));
#66287=CARTESIAN_POINT('Ctrl Pts',(0.607973748439418,-10.5658372241333,
3.69335407655768));
#66288=CARTESIAN_POINT('Ctrl Pts',(0.643682625723488,-8.20946185826682,
7.19379340695978));
#66289=CARTESIAN_POINT('Ctrl Pts',(0.670851656178822,-6.6941661911063,8.48871903980218));
#66290=CARTESIAN_POINT('Ctrl Pts',(0.11603639422774,-4.20098941410116,-9.22140044511724));
#66291=CARTESIAN_POINT('Ctrl Pts',(0.128651711507678,-5.14922408433979,
-8.81403982725145));
#66292=CARTESIAN_POINT('Ctrl Pts',(0.169416672559358,-7.78615968126346,
-7.17995266741247));
#66293=CARTESIAN_POINT('Ctrl Pts',(0.251307272645807,-10.6445810843281,
-2.66074290006108));
#66294=CARTESIAN_POINT('Ctrl Pts',(0.379918724725771,-10.4931844219905,
3.68853728670262));
#66295=CARTESIAN_POINT('Ctrl Pts',(0.487855668801451,-8.14709590799179,
7.15349993224077));
#66296=CARTESIAN_POINT('Ctrl Pts',(0.56701689065259,-6.64808612899144,8.45016391490677));
#66297=CARTESIAN_POINT('Ctrl Pts',(-0.263756150020116,-4.13508037506425,
-9.03493950971657));
#66298=CARTESIAN_POINT('Ctrl Pts',(-0.238822515641171,-5.06541537697735,
-8.63644332671582));
#66299=CARTESIAN_POINT('Ctrl Pts',(-0.161580251226922,-7.65452628554427,
-7.03742568805577));
#66300=CARTESIAN_POINT('Ctrl Pts',(-0.019254670531333,-10.4739580436883,
-2.60642705242705));
#66301=CARTESIAN_POINT('Ctrl Pts',(0.187728836148095,-10.353432692806,3.64864328643095));
#66302=CARTESIAN_POINT('Ctrl Pts',(0.35342602904065,-8.06080450131726,7.08924457321249));
#66303=CARTESIAN_POINT('Ctrl Pts',(0.475431666076765,-6.59080396888544,
8.39798701307191));
#66304=CARTESIAN_POINT('Ctrl Pts',(-0.408125826329177,-4.08300106590614,
-8.8999945016169));
#66305=CARTESIAN_POINT('Ctrl Pts',(-0.379507549551991,-5.00109873234858,
-8.51029008272195));
#66306=CARTESIAN_POINT('Ctrl Pts',(-0.290906254360935,-7.55953608322051,
-6.9418989057511));
#66307=CARTESIAN_POINT('Ctrl Pts',(-0.12908321161831,-10.3617241905342,
-2.57549773458398));
#66308=CARTESIAN_POINT('Ctrl Pts',(0.105595500813863,-10.2704899304828,
3.62161712433814));
#66309=CARTESIAN_POINT('Ctrl Pts',(0.293278752248673,-8.0127450289758,7.05198273979294));
#66310=CARTESIAN_POINT('Ctrl Pts',(0.433434319459543,-6.55982112175522,
8.36891105681224));
#66311=CARTESIAN_POINT('',(0.292893218813451,-8.08129599809058,6.69279187579194));
#66312=CARTESIAN_POINT('Ctrl Pts',(0.435005558411317,-6.57572732894909,
8.35840209456398));
#66313=CARTESIAN_POINT('Ctrl Pts',(0.382251408826999,-7.12834252168661,
7.85646014185166));
#66314=CARTESIAN_POINT('Ctrl Pts',(0.336116843866004,-7.63392213499947,
7.29680540123552));
#66315=CARTESIAN_POINT('Ctrl Pts',(0.294503024240271,-8.08003783661177,
6.69175349258125));
#66316=CARTESIAN_POINT('',(0.125832807865084,-10.1217996775674,-1.74673005675864));
#66317=CARTESIAN_POINT('Ctrl Pts',(0.125832807864998,-10.1217996775674,
-1.74673005675862));
#66318=CARTESIAN_POINT('Ctrl Pts',(0.132205270288902,-10.2171295955181,
-1.26177410637066));
#66319=CARTESIAN_POINT('Ctrl Pts',(0.138916752563787,-10.2776190378748,
-0.769532124451515));
#66320=CARTESIAN_POINT('Ctrl Pts',(0.16417493077499,-10.3658446216758,0.989972291322507));
#66321=CARTESIAN_POINT('Ctrl Pts',(0.1845279037431,-10.1966343705713,2.25432259478106));
#66322=CARTESIAN_POINT('Ctrl Pts',(0.232017154312988,-9.43031413187586,
4.61210749050356));
#66323=CARTESIAN_POINT('Ctrl Pts',(0.258196822839283,-8.85745589801152,
5.69115766808526));
#66324=CARTESIAN_POINT('Ctrl Pts',(0.291919559723898,-8.10307581650266,
6.6648953556432));
#66325=CARTESIAN_POINT('Ctrl Pts',(0.292405594246003,-8.09220329443071,
6.67885723020437));
#66326=CARTESIAN_POINT('Ctrl Pts',(0.292893218813444,-8.08129599809067,
6.69279187579183));
#66327=CARTESIAN_POINT('',(0.475355112906105,-4.16569943627783,-9.16633189758011));
#66328=CARTESIAN_POINT('Ctrl Pts',(0.475355112906066,-4.16569943627857,
-9.16633189757981));
#66329=CARTESIAN_POINT('Ctrl Pts',(0.427886534680796,-5.08975858274379,
-8.7917566486846));
#66330=CARTESIAN_POINT('Ctrl Pts',(0.385530767363199,-5.95263627434214,
-8.2728587056254));
#66331=CARTESIAN_POINT('Ctrl Pts',(0.29926267203596,-7.64515638769987,-6.86186047960224));
#66332=CARTESIAN_POINT('Ctrl Pts',(0.257497246713814,-8.41962158888031,
-5.92768421433392));
#66333=CARTESIAN_POINT('Ctrl Pts',(0.184526253224387,-9.55248442131784,
-3.90485136748501));
#66334=CARTESIAN_POINT('Ctrl Pts',(0.153282207439182,-9.92949895697148,
-2.84555641526849));
#66335=CARTESIAN_POINT('Ctrl Pts',(0.125832807865115,-10.1217996775674,
-1.74673005675863));
#66336=CARTESIAN_POINT('Ctrl Pts',(0.724999999999999,-5.84323637812459,
-8.19946832906631));
#66337=CARTESIAN_POINT('Ctrl Pts',(0.640484621491153,-5.17453815259049,
-8.6760067630983));
#66338=CARTESIAN_POINT('Ctrl Pts',(0.55690999773333,-4.57007071997486,-8.98256272498574));
#66339=CARTESIAN_POINT('Ctrl Pts',(0.475355112906103,-4.16569943627783,
-9.16633189758011));
#66340=CARTESIAN_POINT('Origin',(0.399999999999991,0.,0.));
#66341=CARTESIAN_POINT('',(0.292893218813464,-1.71858793961045,-10.3512544686487));
#66342=CARTESIAN_POINT('Ctrl Pts',(0.292893218813463,-1.71858793961049,
-10.3512544686487));
#66343=CARTESIAN_POINT('Ctrl Pts',(0.295370685504836,-1.54953129267453,
-10.3816491189871));
#66344=CARTESIAN_POINT('Ctrl Pts',(0.297849178161302,-1.37958511318198,
-10.4079194567052));
#66345=CARTESIAN_POINT('Ctrl Pts',(0.30032945062728,-1.20890379305856,-10.4300457424659));
#66346=CARTESIAN_POINT('Ctrl Pts',(0.301142734555239,-1.15293721020792,
-10.4373009746395));
#66347=CARTESIAN_POINT('Ctrl Pts',(0.301956209846706,-1.09689158818819,
-10.4441105603769));
#66348=CARTESIAN_POINT('Ctrl Pts',(0.302769903078932,-1.04077238530596,
-10.4504735638106));
#66349=CARTESIAN_POINT('Ctrl Pts',(0.303351314427838,-1.00067331583471,
-10.4550201450809));
#66350=CARTESIAN_POINT('Ctrl Pts',(0.303932923881008,-0.960530674908709,
-10.4593392685354));
#66351=CARTESIAN_POINT('Ctrl Pts',(0.30451425402037,-0.920380122981467,
-10.4634273085986));
#66352=CARTESIAN_POINT('Ctrl Pts',(0.308224974168982,-0.66409294307074,
-10.4895219003007));
#66353=CARTESIAN_POINT('Ctrl Pts',(0.311927374753782,-0.407274147500252,
-10.5062318220592));
#66354=CARTESIAN_POINT('Ctrl Pts',(0.315623936094389,-0.150459369271352,
-10.5136295680564));
#66355=CARTESIAN_POINT('Ctrl Pts',(0.31936105791558,0.109173306421204,-10.5211084857442));
#66356=CARTESIAN_POINT('Ctrl Pts',(0.323092211647468,0.368802502438476,
-10.5190698591536));
#66357=CARTESIAN_POINT('Ctrl Pts',(0.326819960154648,0.627887657781203,
-10.5075372262153));
#66358=CARTESIAN_POINT('Ctrl Pts',(0.330545124169206,0.886793186287292,
-10.4960125889893));
#66359=CARTESIAN_POINT('Ctrl Pts',(0.334266887679186,1.1451560830394,-10.4750071262638));
#66360=CARTESIAN_POINT('Ctrl Pts',(0.337987808222285,1.40244003864855,-10.4444924879455));
#66361=CARTESIAN_POINT('Ctrl Pts',(0.341671322008511,1.65713749495914,-10.4142846160963));
#66362=CARTESIAN_POINT('Ctrl Pts',(0.345354009691509,1.91077821648196,-10.374757752577));
#66363=CARTESIAN_POINT('Ctrl Pts',(0.34903835244832,2.16283547778415,-10.3258339017055));
#66364=CARTESIAN_POINT('Ctrl Pts',(0.350081930208472,2.23422985380774,-10.3119763846175));
#66365=CARTESIAN_POINT('Ctrl Pts',(0.351125640752989,2.30549711945091,-10.2973646488453));
#66366=CARTESIAN_POINT('Ctrl Pts',(0.352169540465385,2.37662510408095,-10.2819961824987));
#66367=CARTESIAN_POINT('Ctrl Pts',(0.355325621437656,2.59167035816169,-10.2355318300004));
#66368=CARTESIAN_POINT('Ctrl Pts',(0.358483431533814,2.80544332134696,-10.1821522462807));
#66369=CARTESIAN_POINT('Ctrl Pts',(0.36164452894309,3.01764956468017,-10.1219806909546));
#66370=CARTESIAN_POINT('Ctrl Pts',(0.362244945216604,3.05795584612044,-10.1105517546256));
#66371=CARTESIAN_POINT('Ctrl Pts',(0.362845578583556,3.09821214519677,-10.0988757007015));
#66372=CARTESIAN_POINT('Ctrl Pts',(0.363445922707591,3.13838184933902,-10.0869637126654));
#66373=CARTESIAN_POINT('Ctrl Pts',(0.367131837381407,3.38501056779072,-10.0138280397424));
#66374=CARTESIAN_POINT('Ctrl Pts',(0.370809553744273,3.62855766148032,-9.93175459699036));
#66375=CARTESIAN_POINT('Ctrl Pts',(0.374481502668837,3.86859366032192,-9.84107991525181));
#66376=CARTESIAN_POINT('Ctrl Pts',(0.378195725709086,4.11139312613754,-9.74936132139353));
#66377=CARTESIAN_POINT('Ctrl Pts',(0.381904047748811,4.35060076429901,-9.64884211119538));
#66378=CARTESIAN_POINT('Ctrl Pts',(0.385608984588813,4.58576422516573,-9.53981779427593));
#66379=CARTESIAN_POINT('Ctrl Pts',(0.389331721631913,4.82205751834679,-9.43026967490923));
#66380=CARTESIAN_POINT('Ctrl Pts',(0.39305104086907,5.05426827607086,-9.31213427953758));
#66381=CARTESIAN_POINT('Ctrl Pts',(0.396769494536738,5.28192083979082,-9.18566181599591));
#66382=CARTESIAN_POINT('Ctrl Pts',(0.400470324926094,5.50849446456264,-9.05978875737441));
#66383=CARTESIAN_POINT('Ctrl Pts',(0.404170297931097,5.73055356171349,-8.92565715833079));
#66384=CARTESIAN_POINT('Ctrl Pts',(0.407871929671624,5.94760402087416,-8.78346899095218));
#66385=CARTESIAN_POINT('Ctrl Pts',(0.411165837008073,6.14074697779815,-8.65694245332906));
#66386=CARTESIAN_POINT('Ctrl Pts',(0.414461057794326,6.32992383703218,-8.52403568235594));
#66387=CARTESIAN_POINT('Ctrl Pts',(0.417759364936873,6.51476406975381,-8.38486391006944));
#66388=CARTESIAN_POINT('Ctrl Pts',(0.418667417814794,6.56565220661442,-8.34654870081564));
#66389=CARTESIAN_POINT('Ctrl Pts',(0.419575704622837,6.61621150904747,-8.30775849513671));
#66390=CARTESIAN_POINT('Ctrl Pts',(0.420484262356252,6.66643391070339,-8.26849538237134));
#66391=CARTESIAN_POINT('Ctrl Pts',(0.420875964578254,6.68808605849699,-8.25156806124765));
#66392=CARTESIAN_POINT('Ctrl Pts',(0.421267748956308,6.70967733121888,-8.23455145055552));
#66393=CARTESIAN_POINT('Ctrl Pts',(0.421659515941323,6.73120144365869,-8.21745018822553));
#66394=CARTESIAN_POINT('Ctrl Pts',(0.423659727562703,6.84109528741988,-8.13013771688129));
#66395=CARTESIAN_POINT('Ctrl Pts',(0.425657482755154,6.94912881506172,-8.04070675268601));
#66396=CARTESIAN_POINT('Ctrl Pts',(0.427653169672452,7.05523324461425,-7.94920222677801));
#66397=CARTESIAN_POINT('Ctrl Pts',(0.4291387996276,7.13421954128772,-7.88108439549787));
#66398=CARTESIAN_POINT('Ctrl Pts',(0.430623283423957,7.21213678679135,-7.81181740016394));
#66399=CARTESIAN_POINT('Ctrl Pts',(0.432106781186298,7.2889708632371,-7.74143516723137));
#66400=CARTESIAN_POINT('',(0.292893218813452,-1.28500880942149E-15,10.4928932188135));
#66401=CARTESIAN_POINT('Origin',(0.292893218813452,0.,-1.60626101177686E-15));
#66402=CARTESIAN_POINT('Origin',(0.292893218813452,0.,-1.60626101177686E-15));
#66403=CARTESIAN_POINT('Origin',(43.,7.36678071053767,-7.8083313754256));
#66404=CARTESIAN_POINT('',(43.,7.42881003951057,-8.80640570249106));
#66405=CARTESIAN_POINT('',(43.,8.35955976908767,-7.92828862157849));
#66406=CARTESIAN_POINT('Origin',(43.,10.6623800874337,-1.24625349616493));
#66407=CARTESIAN_POINT('',(43.,11.5,-0.7));
#66408=CARTESIAN_POINT('',(43.,11.3514471211877,-1.97095110413219));
#66409=CARTESIAN_POINT('Origin',(43.,8.96893332226436,-5.89896024451612));
#66410=CARTESIAN_POINT('',(43.,9.25946242264882,-6.85582640121192));
#66411=CARTESIAN_POINT('',(43.,9.96261593757892,-5.78673342053171));
#66412=CARTESIAN_POINT('Origin',(1.,0.,0.));
#66413=CARTESIAN_POINT('',(0.,-1.19841320379794E-15,9.78578643762691));
#66414=CARTESIAN_POINT('Origin',(1.,-1.19841320379794E-15,9.78578643762691));
#66415=CARTESIAN_POINT('Origin',(0.,0.,0.));
#66416=CARTESIAN_POINT('Ctrl Pts',(0.292893218813464,-1.71858793961045,
-10.3512544686487));
#66417=CARTESIAN_POINT('Ctrl Pts',(0.291330567135518,-1.82522246842754,
-10.332082603105));
#66418=CARTESIAN_POINT('Ctrl Pts',(0.289770284081505,-1.93162153324712,
-10.311241812675));
#66419=CARTESIAN_POINT('Ctrl Pts',(0.288212344255969,-2.03774315891834,
-10.288723757919));
#66420=CARTESIAN_POINT('Ctrl Pts',(0.284388495362714,-2.29821089600425,
-10.2334548461512));
#66421=CARTESIAN_POINT('Ctrl Pts',(0.280592473031578,-2.55603087173463,
-10.1682940675651));
#66422=CARTESIAN_POINT('Ctrl Pts',(0.276821992997328,-2.8106315051574,-10.0933032792352));
#66423=CARTESIAN_POINT('Ctrl Pts',(0.27319178413024,-3.05576036636922,-10.0211023333947));
#66424=CARTESIAN_POINT('Ctrl Pts',(0.269585252438158,-3.29790561863323,
-9.93978895171091));
#66425=CARTESIAN_POINT('Ctrl Pts',(0.266000359229949,-3.53664200198086,
-9.84969425493053));
#66426=CARTESIAN_POINT('Ctrl Pts',(0.262374337422124,-3.77811734924026,
-9.75856592381398));
#66427=CARTESIAN_POINT('Ctrl Pts',(0.258770453452344,-4.01610574925818,
-9.65845337162361));
#66428=CARTESIAN_POINT('Ctrl Pts',(0.25518659765317,-4.25014962204483,-9.54964920416749));
#66429=CARTESIAN_POINT('Ctrl Pts',(0.251604729076463,-4.48406371917409,
-9.44090536784583));
#66430=CARTESIAN_POINT('Ctrl Pts',(0.248042866465565,-4.71403822595297,
-9.3234792015879));
#66431=CARTESIAN_POINT('Ctrl Pts',(0.244498903660475,-4.93959030274802,
-9.19761786010767));
#66432=CARTESIAN_POINT('Ctrl Pts',(0.240990742110669,-5.16286384336041,
-9.07302797497862));
#66433=CARTESIAN_POINT('Ctrl Pts',(0.237500120544247,-5.38180435007924,
-8.94017208700871));
#66434=CARTESIAN_POINT('Ctrl Pts',(0.234024995988112,-5.59591015114204,
-8.79925149071518));
#66435=CARTESIAN_POINT('Ctrl Pts',(0.232960928997251,-5.66146835251949,
-8.75610225896068));
#66436=CARTESIAN_POINT('Ctrl Pts',(0.2318983149378,-5.72657300664438,-8.7121966635391));
#66437=CARTESIAN_POINT('Ctrl Pts',(0.230837095161052,-5.79120896769444,
-8.66753983740276));
#66438=CARTESIAN_POINT('Ctrl Pts',(0.227358029862829,-6.00310921120067,
-8.52113848158199));
#66439=CARTESIAN_POINT('Ctrl Pts',(0.223906601041763,-6.20920033169496,
-8.36720119226211));
#66440=CARTESIAN_POINT('Ctrl Pts',(0.220481063087816,-6.40905516126478,
-8.20604534608939));
#66441=CARTESIAN_POINT('Ctrl Pts',(0.217054296845572,-6.60898165238136,
-8.04483171458705));
#66442=CARTESIAN_POINT('Ctrl Pts',(0.213653440041048,-6.80266792814952,
-7.87639398395583));
#66443=CARTESIAN_POINT('Ctrl Pts',(0.210276745185777,-6.98965925623536,
-7.7010056291283));
#66444=CARTESIAN_POINT('Ctrl Pts',(0.208756517146038,-7.07384496810101,
-7.62204371332585));
#66445=CARTESIAN_POINT('Ctrl Pts',(0.207241186508959,-7.15667326118802,
-7.54167240817136));
#66446=CARTESIAN_POINT('Ctrl Pts',(0.205730593809645,-7.23810039237002,
-7.45991404149759));
#66447=CARTESIAN_POINT('Ctrl Pts',(0.202372519099092,-7.41911436794365,
-7.27816372347462));
#66448=CARTESIAN_POINT('Ctrl Pts',(0.199037858371459,-7.59320684721615,
-7.08956092043285));
#66449=CARTESIAN_POINT('Ctrl Pts',(0.195724859788499,-7.76010964904612,
-6.89458007875885));
#66450=CARTESIAN_POINT('Ctrl Pts',(0.192417926702888,-7.92670688222682,
-6.69995621151408));
#66451=CARTESIAN_POINT('Ctrl Pts',(0.189132576515672,-8.0861410603453,-6.49897705430775));
#66452=CARTESIAN_POINT('Ctrl Pts',(0.185867066992887,-8.23810179363612,
-6.29208696278111));
#66453=CARTESIAN_POINT('Ctrl Pts',(0.183066686923793,-8.36841769252515,
-6.1146656798966));
#66454=CARTESIAN_POINT('Ctrl Pts',(0.180280897962253,-8.49323692936344,
-5.93289676293096));
#66455=CARTESIAN_POINT('Ctrl Pts',(0.177508601343955,-8.61233534860918,
-5.74704918122061));
#66456=CARTESIAN_POINT('Ctrl Pts',(0.17429172943195,-8.75053281171868,-5.53139842380447));
#66457=CARTESIAN_POINT('Ctrl Pts',(0.171104705604424,-8.88052271436299,
-5.31104632067348));
#66458=CARTESIAN_POINT('Ctrl Pts',(0.167946257256198,-9.00209070919836,
-5.08649297571782));
#66459=CARTESIAN_POINT('Ctrl Pts',(0.164779523498679,-9.12397760764813,
-4.86135057051295));
#66460=CARTESIAN_POINT('Ctrl Pts',(0.161641515338527,-9.23739868230339,
-4.63198426685119));
#66461=CARTESIAN_POINT('Ctrl Pts',(0.158530950129171,-9.34209507871624,
-4.39886763892668));
#66462=CARTESIAN_POINT('Ctrl Pts',(0.155443777182003,-9.44600413090373,
-4.16750410888441));
#66463=CARTESIAN_POINT('Ctrl Pts',(0.152383635981344,-9.54131948405809,
-3.93244584919283));
#66464=CARTESIAN_POINT('Ctrl Pts',(0.149349272601062,-9.62774177162519,
-3.69413477335953));
#66465=CARTESIAN_POINT('Ctrl Pts',(0.146691673443462,-9.70343336483665,
-3.48541378809569));
#66466=CARTESIAN_POINT('Ctrl Pts',(0.144053848078294,-9.77230266037022,
-3.27419706912089));
#66467=CARTESIAN_POINT('Ctrl Pts',(0.141434954068194,-9.83411665656242,
-3.06077343288983));
#66468=CARTESIAN_POINT('Ctrl Pts',(0.138426785307503,-9.90511874049622,
-2.81562631627215));
#66469=CARTESIAN_POINT('Ctrl Pts',(0.135443594120566,-9.96681311658494,
-2.56756692392355));
#66470=CARTESIAN_POINT('Ctrl Pts',(0.132484103802723,-10.0191384154099,
-2.31712733653137));
#66471=CARTESIAN_POINT('Ctrl Pts',(0.131224405632153,-10.0414105217949,
-2.21052847787847));
#66472=CARTESIAN_POINT('Ctrl Pts',(0.129969001475245,-10.0619845399194,
-2.10349839539028));
#66473=CARTESIAN_POINT('Ctrl Pts',(0.128717792876683,-10.0808528748036,
-1.99607835619919));
#66474=CARTESIAN_POINT('Ctrl Pts',(0.12775241951272,-10.0954107893995,-1.91319813565873));
#66475=CARTESIAN_POINT('Ctrl Pts',(0.126790832213565,-10.1089354598065,
-1.83018611430223));
#66476=CARTESIAN_POINT('Ctrl Pts',(0.125832807865099,-10.1214304492659,
-1.74706222539384));
#66477=CARTESIAN_POINT('Origin',(0.,10.2,0.));
#66478=CARTESIAN_POINT('',(-2.77555756156289E-16,-3.5,4.28626379701574E-16));
#66479=CARTESIAN_POINT('Origin',(-2.77555756156289E-16,0.,0.));
#66480=CARTESIAN_POINT('Origin',(43.,10.0875684170659,-3.67157463993583));
#66481=CARTESIAN_POINT('',(43.,10.5909347898596,-4.53564772407893));
#66482=CARTESIAN_POINT('',(43.,11.0285849021483,-3.33321392294394));
#66483=CARTESIAN_POINT('Origin',(1.,0.,0.));
#66484=CARTESIAN_POINT('',(1.,-2.5,-3.06161699786838E-16));
#66485=CARTESIAN_POINT('Origin',(1.,0.,0.));
#66486=CARTESIAN_POINT('Origin',(1.,-3.5,-4.28626379701574E-16));
#66487=CARTESIAN_POINT('Origin',(4.3,0.,0.));
#66488=CARTESIAN_POINT('',(8.,-2.5,-3.06161699786838E-16));
#66489=CARTESIAN_POINT('',(4.3,-2.5,-3.06161699786838E-16));
#66490=CARTESIAN_POINT('Origin',(8.,0.,0.));
#66491=CARTESIAN_POINT('Origin',(-2.04781266907391,0.,0.));
#66492=CARTESIAN_POINT('',(0.724999999999993,5.84349639654627,-8.1993893803249));
#66493=CARTESIAN_POINT('Ctrl Pts',(0.475355112906608,-4.16530317223385,
-9.16608022370811));
#66494=CARTESIAN_POINT('Ctrl Pts',(0.487687460938802,-3.69195469470312,
-9.381686696241));
#66495=CARTESIAN_POINT('Ctrl Pts',(0.539707849920727,-1.62562104739945,
-10.1372037941637));
#66496=CARTESIAN_POINT('Ctrl Pts',(0.622922812285357,1.99424355166152,-10.2177440901867));
#66497=CARTESIAN_POINT('Ctrl Pts',(0.693805426617792,4.77136435052723,-8.96178055745778));
#66498=CARTESIAN_POINT('Ctrl Pts',(0.725000000000497,5.84349639654576,-8.19938938032419));
#66499=CARTESIAN_POINT('Ctrl Pts',(0.725000000000497,5.84349639654576,-8.19938938032419));
#66500=CARTESIAN_POINT('Ctrl Pts',(0.733493467567523,6.13540994986514,-7.99181017553978));
#66501=CARTESIAN_POINT('Ctrl Pts',(0.781674976084279,7.72826920962671,-6.72609144941552));
#66502=CARTESIAN_POINT('Ctrl Pts',(0.869544525550766,9.87292364246029,-3.56115337744866));
#66503=CARTESIAN_POINT('Ctrl Pts',(0.988608648399958,10.373608620426,1.59501402068791));
#66504=CARTESIAN_POINT('Ctrl Pts',(1.10767277124915,8.34708153225567,6.36256533997802));
#66505=CARTESIAN_POINT('Ctrl Pts',(1.22673689409834,4.28699419088582,9.58006712539813));
#66506=CARTESIAN_POINT('Ctrl Pts',(1.34580101694754,-0.817493434454986,
10.463635277209));
#66507=CARTESIAN_POINT('Ctrl Pts',(1.46486513979672,-5.72282606115532,8.79802612159381));
#66508=CARTESIAN_POINT('Ctrl Pts',(1.58366057778975,-9.22602072287202,4.99760873621947));
#66509=CARTESIAN_POINT('Ctrl Pts',(1.66276797483305,-10.0692455480444,1.66204732692402));
#66510=CARTESIAN_POINT('Ctrl Pts',(1.70218733092661,-10.0693625248661,-1.1992009720295E-5));
#66511=CARTESIAN_POINT('Ctrl Pts',(-0.339340843899389,-10.7137153436476,
2.13820797253966));
#66512=CARTESIAN_POINT('Ctrl Pts',(-0.299652802949658,-11.0691814654222,
0.357107681121413));
#66513=CARTESIAN_POINT('Ctrl Pts',(-0.220276721050197,-10.874371249301,
-3.38398574376631));
#66514=CARTESIAN_POINT('Ctrl Pts',(-0.101212598201006,-7.93014445777923,
-8.17355408554336));
#66515=CARTESIAN_POINT('Ctrl Pts',(0.0178515246481864,-3.05511357269883,
-10.9708197458404));
#66516=CARTESIAN_POINT('Ctrl Pts',(0.136915647497378,2.56478531368309,-11.095859870282));
#66517=CARTESIAN_POINT('Ctrl Pts',(0.25597977034657,7.55955037712473,-8.51742713350504));
#66518=CARTESIAN_POINT('Ctrl Pts',(0.375043893195762,10.7127867072662,-3.86409111890594));
#66519=CARTESIAN_POINT('Ctrl Pts',(0.494108016044953,11.2560636099064,1.73069757424675));
#66520=CARTESIAN_POINT('Ctrl Pts',(0.613172138894146,9.05714531191615,6.90381166376007));
#66521=CARTESIAN_POINT('Ctrl Pts',(0.732236261743336,4.65167725847051,10.3950176738234));
#66522=CARTESIAN_POINT('Ctrl Pts',(0.85130038459253,-0.887035402587716,
11.3537485922895));
#66523=CARTESIAN_POINT('Ctrl Pts',(0.97036450744172,-6.20965148482242,9.546450544826));
#66524=CARTESIAN_POINT('Ctrl Pts',(1.08942863029091,-10.0194508413342,5.41341509935058));
#66525=CARTESIAN_POINT('Ctrl Pts',(1.2084927531401,-11.3882832174297,-0.0384513017546332));
#66526=CARTESIAN_POINT('Ctrl Pts',(1.3275568759893,-9.98266729745013,-5.48095079261517));
#66527=CARTESIAN_POINT('Ctrl Pts',(1.44662099883849,-6.14504460896131,-9.58816434057055));
#66528=CARTESIAN_POINT('Ctrl Pts',(1.56568512168768,-0.810347620278259,
-11.3594808926036));
#66529=CARTESIAN_POINT('Ctrl Pts',(1.68474924453687,4.72176856349981,-10.3633667395971));
#66530=CARTESIAN_POINT('Ctrl Pts',(1.80381336738606,9.10355346673582,-6.84249833133797));
#66531=CARTESIAN_POINT('Ctrl Pts',(1.92287749023525,11.2675035006204,-1.65464005039914));
#66532=CARTESIAN_POINT('Ctrl Pts',(2.04194161308445,10.6864307496016,3.93632655969533));
#66533=CARTESIAN_POINT('Ctrl Pts',(2.16100573593364,7.5018978670731,8.56831356317135));
#66534=CARTESIAN_POINT('Ctrl Pts',(2.28006985878283,2.48973026125074,11.1128624639612));
#66535=CARTESIAN_POINT('Ctrl Pts',(2.39913398163202,-3.12899285671391,10.9500626771552));
#66536=CARTESIAN_POINT('Ctrl Pts',(2.51819810448121,-7.98542140390107,8.11957596936534));
#66537=CARTESIAN_POINT('Ctrl Pts',(2.63726222733041,-10.896417778522,3.3109739537018));
#66538=CARTESIAN_POINT('Ctrl Pts',(2.75632635017959,-11.1527963630143,-2.30425740939608));
#66539=CARTESIAN_POINT('Ctrl Pts',(2.87539047302879,-8.6920974426009,-7.35811871150985));
#66540=CARTESIAN_POINT('Ctrl Pts',(2.99445459587798,-4.11380382528908,-10.6193731929624));
#66541=CARTESIAN_POINT('Ctrl Pts',(3.11351871872717,1.46670694632534,-11.2935043125574));
#66542=CARTESIAN_POINT('Ctrl Pts',(3.23258284157637,6.68989419831079,-9.21627823688887));
#66543=CARTESIAN_POINT('Ctrl Pts',(3.35164696442556,10.2832694779525,-4.8937549762976));
#66544=CARTESIAN_POINT('Ctrl Pts',(3.47071108727475,11.3714039850141,0.62099946367668));
#66545=CARTESIAN_POINT('Ctrl Pts',(3.58977521012394,9.68920314630753,5.98446416263376));
#66546=CARTESIAN_POINT('Ctrl Pts',(3.70883933297313,5.64648974610255,9.88997585797983));
#66547=CARTESIAN_POINT('Ctrl Pts',(3.82790345582233,0.228161677405186,11.3860621451506));
#66548=CARTESIAN_POINT('Ctrl Pts',(3.94696757867151,-5.24575181946737,10.108242021876));
#66549=CARTESIAN_POINT('Ctrl Pts',(4.06603170152071,-9.44167961644461,6.36782183675721));
#66550=CARTESIAN_POINT('Ctrl Pts',(4.18509582436989,-11.3373972723258,1.07605390837347));
#66551=CARTESIAN_POINT('Ctrl Pts',(4.3041599472191,-10.4710643991872,-4.47786548171576));
#66552=CARTESIAN_POINT('Ctrl Pts',(4.42322407006827,-7.05373959478994,-8.9408739311747));
#66553=CARTESIAN_POINT('Ctrl Pts',(4.54228819291748,-1.91796171766544,-11.2256800138716));
#66554=CARTESIAN_POINT('Ctrl Pts',(4.66135231576666,3.68507571204164,-10.7756524591687));
#66555=CARTESIAN_POINT('Ctrl Pts',(4.78041643861586,8.39034400872485,-7.70042832182221));
#66556=CARTESIAN_POINT('Ctrl Pts',(4.89948056146505,11.0515316799081,-2.74920287579044));
#66557=CARTESIAN_POINT('Ctrl Pts',(5.01854468431424,11.0203122500823,2.87179157233809));
#66558=CARTESIAN_POINT('Ctrl Pts',(5.13760880716343,8.3042914898309,7.79315159458538));
#66559=CARTESIAN_POINT('Ctrl Pts',(5.25667293001263,3.56515447532148,10.8159207879571));
#66560=CARTESIAN_POINT('Ctrl Pts',(5.37573705286181,-2.0425361029442,11.2036831083549));
#66561=CARTESIAN_POINT('Ctrl Pts',(5.49480117571101,-7.15261794543326,8.86197074306457));
#66562=CARTESIAN_POINT('Ctrl Pts',(5.61386529856021,-10.5201576765787,4.36127864097101));
#66563=CARTESIAN_POINT('Ctrl Pts',(5.73292942140939,-11.3247452258424,-1.20192116797532));
#66564=CARTESIAN_POINT('Ctrl Pts',(5.85199354425859,-9.37036457537598,-6.47230535812437));
#66565=CARTESIAN_POINT('Ctrl Pts',(5.97105766710777,-5.13314776676402,-10.165887217987));
#66566=CARTESIAN_POINT('Ctrl Pts',(6.09012178995697,0.354621806664209,-11.3828253214439));
#66567=CARTESIAN_POINT('Ctrl Pts',(6.20918591280615,5.75599735815148,-9.82664557909869));
#66568=CARTESIAN_POINT('Ctrl Pts',(6.32825003565535,9.75507967017305,-5.87646913995496));
#66569=CARTESIAN_POINT('Ctrl Pts',(6.44731415850455,11.3776003855219,-0.494649766643108));
#66570=CARTESIAN_POINT('Ctrl Pts',(6.56637828135373,10.2282761695373,5.00767765775123));
#66571=CARTESIAN_POINT('Ctrl Pts',(6.68544240420294,6.58710881474078,9.29001971941025));
#66572=CARTESIAN_POINT('Ctrl Pts',(6.80450652705211,1.34117036923918,11.3090994763041));
#66573=CARTESIAN_POINT('Ctrl Pts',(6.92357064990131,-4.23150800068092,10.5730226976225));
#66574=CARTESIAN_POINT('Ctrl Pts',(7.0426347727505,-8.77329377408233,7.26111460300103));
#66575=CARTESIAN_POINT('Ctrl Pts',(7.1616988955997,-11.1777035582784,2.18023211780689));
#66576=CARTESIAN_POINT('Ctrl Pts',(7.28076301844888,-10.8589678722411,-3.43180501688287));
#66577=CARTESIAN_POINT('Ctrl Pts',(7.39982714129808,-7.89473805419999,-8.20777558049885));
#66578=CARTESIAN_POINT('Ctrl Pts',(7.51889126414727,-3.00716861108435,-10.9841433834767));
#66579=CARTESIAN_POINT('Ctrl Pts',(7.63795538699645,2.61301621575537,-11.0845214231588));
#66580=CARTESIAN_POINT('Ctrl Pts',(7.75701950984565,7.59661024069373,-8.48445530221321));
#66581=CARTESIAN_POINT('Ctrl Pts',(7.87608363269484,10.7294954274332,-3.81738088182957));
#66582=CARTESIAN_POINT('Ctrl Pts',(7.99514775554403,11.2484289452302,1.77969525154554));
#66583=CARTESIAN_POINT('Ctrl Pts',(8.11421187839323,9.02698666313771,6.9431967210933));
#66584=CARTESIAN_POINT('Ctrl Pts',(8.23327600124242,4.60636297375381,10.4151759024174));
#66585=CARTESIAN_POINT('Ctrl Pts',(8.3523401240916,-0.93647659842093,11.3497788747128));
#66586=CARTESIAN_POINT('Ctrl Pts',(8.47140424694081,-6.25116894932857,9.51931487509565));
#66587=CARTESIAN_POINT('Ctrl Pts',(8.59046836978998,-10.042932881239,5.36972700117933));
#66588=CARTESIAN_POINT('Ctrl Pts',(8.70953249263918,-11.3880075588841,-0.088049776066923));
#66589=CARTESIAN_POINT('Ctrl Pts',(8.82859661548838,-9.95870187858956,-5.52437560432338));
#66590=CARTESIAN_POINT('Ctrl Pts',(8.94766073833756,-6.10322755205279,-9.61483657542498));
#66591=CARTESIAN_POINT('Ctrl Pts',(9.06672486118676,-0.760866730850746,
-11.3629023907693));
#66592=CARTESIAN_POINT('Ctrl Pts',(9.18578898403595,4.76685871205243,-10.3427040440881));
#66593=CARTESIAN_POINT('Ctrl Pts',(9.30485310688515,9.13326782183868,-6.80278529859885));
#66594=CARTESIAN_POINT('Ctrl Pts',(9.42391722973433,11.2746029915446,-1.60555171430894));
#66595=CARTESIAN_POINT('Ctrl Pts',(9.54298135258353,10.6691857621528,3.98283116601037));
#66596=CARTESIAN_POINT('Ctrl Pts',(9.66204547543272,7.46450968430391,8.60090484177098));
#66597=CARTESIAN_POINT('Ctrl Pts',(9.78110959828191,2.4413074996976,11.1236004340405));
#66598=CARTESIAN_POINT('Ctrl Pts',(9.9001737211311,-3.17665329740789,10.9363313205268));
#66599=CARTESIAN_POINT('Ctrl Pts',(10.0192378439803,-8.02070834614241,8.08472056105763));
#66600=CARTESIAN_POINT('Ctrl Pts',(10.1383019668295,-10.9107345116646,3.26348607170872));
#66601=CARTESIAN_POINT('Ctrl Pts',(10.2573660896787,-11.1426550021304,-2.35280862540185));
#66602=CARTESIAN_POINT('Ctrl Pts',(10.3764302125279,-8.65996865611833,-7.39590506965271));
#66603=CARTESIAN_POINT('Ctrl Pts',(10.4954943353771,-4.06751492404904,-10.6371890679307));
#66604=CARTESIAN_POINT('Ctrl Pts',(10.6145584582263,1.51587892221994,-11.2870093478049));
#66605=CARTESIAN_POINT('Ctrl Pts',(10.7336225810754,6.7299698254521,-9.18705475507634));
#66606=CARTESIAN_POINT('Ctrl Pts',(10.8526867039246,10.3044854125708,-4.84892248921169));
#66607=CARTESIAN_POINT('Ctrl Pts',(10.9717508267738,11.3685915378509,0.67051873185693));
#66608=CARTESIAN_POINT('Ctrl Pts',(11.090814949623,9.66304749412977,6.02660618013646));
#66609=CARTESIAN_POINT('Ctrl Pts',(11.2098790724722,5.60336300688245,9.91447386084446));
#66610=CARTESIAN_POINT('Ctrl Pts',(11.3289431953214,0.17857051594646,11.3869478568711));
#66611=CARTESIAN_POINT('Ctrl Pts',(11.4480073181706,-5.28972585654102,10.0852996627224));
#66612=CARTESIAN_POINT('Ctrl Pts',(11.5670714410198,-9.46932344310051,6.32664069267518));
#66613=CARTESIAN_POINT('Ctrl Pts',(11.686135563869,-11.3419762170866,1.02666665247721));
#66614=CARTESIAN_POINT('Ctrl Pts',(11.8051996867182,-10.4514629258768,-4.52342697888334));
#66615=CARTESIAN_POINT('Ctrl Pts',(11.9242638095674,-7.0147330727834,-8.97150984181957));
#66616=CARTESIAN_POINT('Ctrl Pts',(12.0433279324165,-1.86905303216254,-11.2339267260932));
#66617=CARTESIAN_POINT('Ctrl Pts',(12.1623920552658,3.73197128124412,-10.7595008843457));
#66618=CARTESIAN_POINT('Ctrl Pts',(12.2814561781149,8.42380162322588,-7.66381335477341));
#66619=CARTESIAN_POINT('Ctrl Pts',(12.4005203009641,11.0634002959,-2.70104476396572));
#66620=CARTESIAN_POINT('Ctrl Pts',(12.5195844238133,11.0077003999476,2.91976040613947));
#66621=CARTESIAN_POINT('Ctrl Pts',(12.6386485466625,8.2702717101051,7.82924484004058));
#66622=CARTESIAN_POINT('Ctrl Pts',(12.7577126695117,3.51801476618059,10.8313453009865));
#66623=CARTESIAN_POINT('Ctrl Pts',(12.8767767923609,-2.09131142499942,11.1946811231019));
#66624=CARTESIAN_POINT('Ctrl Pts',(12.9958409152101,-7.19114609100685,8.83073535001835));
#66625=CARTESIAN_POINT('Ctrl Pts',(13.1149050380593,-10.5390523039637,4.31541949972229));
#66626=CARTESIAN_POINT('Ctrl Pts',(13.2339691609085,-11.3194031695759,-1.25123171669396));
#66627=CARTESIAN_POINT('Ctrl Pts',(13.3530332837577,-9.34208728313449,-6.51305413140129));
#66628=CARTESIAN_POINT('Ctrl Pts',(13.4720974066068,-5.08882423679978,-10.188146878173));
#66629=CARTESIAN_POINT('Ctrl Pts',(13.5911615294561,0.404193343818669,-11.3811729037512));
#66630=CARTESIAN_POINT('Ctrl Pts',(13.7102256523052,5.7987401368036,-9.80148365045262));
#66631=CARTESIAN_POINT('Ctrl Pts',(13.8292897751544,9.78058056713834,-5.8339277244394));
#66632=CARTESIAN_POINT('Ctrl Pts',(13.9483538980036,11.3796467962436,-0.44509293075486));
#66633=CARTESIAN_POINT('Ctrl Pts',(14.0674180208528,10.2063695413338,5.05217672988585));
#66634=CARTESIAN_POINT('Ctrl Pts',(14.186482143702,6.5465861056954,9.31862003115172));
#66635=CARTESIAN_POINT('Ctrl Pts',(14.3055462665512,1.29190384255911,11.3148333344264));
#66636=CARTESIAN_POINT('Ctrl Pts',(14.4246103894004,-4.27751588686446,10.5544932025128));
#66637=CARTESIAN_POINT('Ctrl Pts',(14.5436745122496,-8.80483444135218,7.22283596550866));
#66638=CARTESIAN_POINT('Ctrl Pts',(14.6627386350988,-11.1870929752271,2.1315298937359));
#66639=CARTESIAN_POINT('Ctrl Pts',(14.781802757948,-10.8439185611146,-3.47906584648528));
#66640=CARTESIAN_POINT('Ctrl Pts',(14.9008668807972,-7.8589163730486,-8.24208119140396));
#66641=CARTESIAN_POINT('Ctrl Pts',(15.0199310036463,-2.95930154468223,-10.9971361404644));
#66642=CARTESIAN_POINT('Ctrl Pts',(15.1389951264955,2.66126714996277,-11.0730359920302));
#66643=CARTESIAN_POINT('Ctrl Pts',(15.2580592493447,7.63349000624141,-8.45128979794676));
#66644=CARTESIAN_POINT('Ctrl Pts',(15.3771233721939,10.7460192658713,-3.77061518346669));
#66645=CARTESIAN_POINT('Ctrl Pts',(15.4961874950431,11.2405712697682,1.82866794512502));
#66646=CARTESIAN_POINT('Ctrl Pts',(15.6152516178923,8.99666178410144,6.98244553625416));
#66647=CARTESIAN_POINT('Ctrl Pts',(15.7343157407415,4.56095872859594,10.4351389257791));
#66648=CARTESIAN_POINT('Ctrl Pts',(15.8533798635907,-0.985898692109967,
11.3455926549988));
#66649=CARTESIAN_POINT('Ctrl Pts',(15.9724439864399,-6.29256853371875,9.49199927163499));
#66650=CARTESIAN_POINT('Ctrl Pts',(16.0915081092891,-10.0662240661371,5.32593672273604));
#66651=CARTESIAN_POINT('Ctrl Pts',(16.2105722321383,-11.3875160763762,-0.137646411285862));
#66652=CARTESIAN_POINT('Ctrl Pts',(16.3296363549875,-9.93454746510981,-5.56769571616006));
#66653=CARTESIAN_POINT('Ctrl Pts',(16.4487004778366,-6.06129477783599,-9.6413263890631));
#66654=CARTESIAN_POINT('Ctrl Pts',(16.5677646006859,-0.711371383385605,
-11.3661083788237));
#66655=CARTESIAN_POINT('Ctrl Pts',(16.686828723535,4.81185842863261,-10.3218451541894));
#66656=CARTESIAN_POINT('Ctrl Pts',(16.8058928463842,9.16280894240169,-6.76294323570071));
#66657=CARTESIAN_POINT('Ctrl Pts',(16.9249569692334,11.281488620214,-1.55643292057454));
#66658=CARTESIAN_POINT('Ctrl Pts',(17.0440210920826,10.6517384015408,4.02926022359041));
#66659=CARTESIAN_POINT('Ctrl Pts',(17.1630852149318,7.42697991242687,8.63333297774818));
#66660=CARTESIAN_POINT('Ctrl Pts',(17.282149337781,2.39283843148538,11.1341274092348));
#66661=CARTESIAN_POINT('Ctrl Pts',(17.4012134606302,-3.22425348303368,10.9223925218522));
#66662=CARTESIAN_POINT('Ctrl Pts',(17.5202775834794,-8.05584315002668,8.04971180020963));
#66663=CARTESIAN_POINT('Ctrl Pts',(17.6393417063286,-10.9248442881212,3.21593628739332));
#66664=CARTESIAN_POINT('Ctrl Pts',(17.7584058291778,-11.1323022853467,-2.40131521294719));
#66665=CARTESIAN_POINT('Ctrl Pts',(17.8774699520269,-8.6276756058267,-7.43355114093453));
#66666=CARTESIAN_POINT('Ctrl Pts',(17.9965340748762,-4.02114886945205,-10.6548031748114));
#66667=CARTESIAN_POINT('Ctrl Pts',(18.1155981977253,1.56502214464837,-11.2803002890449));
#66668=CARTESIAN_POINT('Ctrl Pts',(18.2346623205745,6.76991779733006,-9.15765701157563));
#66669=CARTESIAN_POINT('Ctrl Pts',(18.3537264434237,10.3255058898736,-4.80399802689931));
#66670=CARTESIAN_POINT('Ctrl Pts',(18.4727905662729,11.3655634492198,0.720025281517934));
#66671=CARTESIAN_POINT('Ctrl Pts',(18.5918546891221,9.63670855154612,6.06863388390041));
#66672=CARTESIAN_POINT('Ctrl Pts',(18.7109188119713,5.56012998207523,9.93878380420335));
#66673=CARTESIAN_POINT('Ctrl Pts',(18.8299829348205,0.128975967330204,11.3876175789371));
#66674=CARTESIAN_POINT('Ctrl Pts',(18.9490470576697,-5.33359955715274,10.0621660038088));
#66675=CARTESIAN_POINT('Ctrl Pts',(19.0681111805189,-9.49678765394332,6.28533954374593));
#66676=CARTESIAN_POINT('Ctrl Pts',(19.1871753033681,-11.3463400252229,0.977259922584966));
#66677=CARTESIAN_POINT('Ctrl Pts',(19.3062394262172,-10.4316632073566,-4.56890267488258));
#66678=CARTESIAN_POINT('Ctrl Pts',(19.4253035490664,-6.97559349407083,-9.00197557926834));
#66679=CARTESIAN_POINT('Ctrl Pts',(19.5443676719156,-1.82010889412883,-11.2419603511923));
#66680=CARTESIAN_POINT('Ctrl Pts',(19.6634317947648,3.77879606175089,-10.7431452213941));
#66681=CARTESIAN_POINT('Ctrl Pts',(19.782495917614,8.45709945355788,-7.6270530191482));
#66682=CARTESIAN_POINT('Ctrl Pts',(19.9015600404632,11.0750590593451,-2.65283541824287));
#66683=CARTESIAN_POINT('Ctrl Pts',(20.0206241633124,10.9948797537916,2.96767385740566));
#66684=CARTESIAN_POINT('Ctrl Pts',(20.1396882861616,8.23609505839278,7.86518957898566));
#66685=CARTESIAN_POINT('Ctrl Pts',(20.2587524090108,3.47080832670908,10.8465643631296));
#66686=CARTESIAN_POINT('Ctrl Pts',(20.37781653186,-2.14004707868723,11.185466795144));
#66687=CARTESIAN_POINT('Ctrl Pts',(20.4968806547092,-7.2295378336409,8.79933245401159));
#66688=CARTESIAN_POINT('Ctrl Pts',(20.6159447775584,-10.5577470247281,4.26947850282809));
#66689=CARTESIAN_POINT('Ctrl Pts',(20.7350089004075,-11.3138464048546,-1.30051853182666));
#66690=CARTESIAN_POINT('Ctrl Pts',(20.8540730232567,-9.31363278851791,-6.55367936390778));
#66691=CARTESIAN_POINT('Ctrl Pts',(20.973137146106,-5.04440418111122,-10.2102132877749));
#66692=CARTESIAN_POINT('Ctrl Pts',(21.0922012689551,0.453757214161865,-11.3793046059442));
#66693=CARTESIAN_POINT('Ctrl Pts',(21.2112653918043,5.8413729239202,-9.77613580551942));
#66694=CARTESIAN_POINT('Ctrl Pts',(21.3303295146535,9.80589594430982,-5.79127564994409));
#66695=CARTESIAN_POINT('Ctrl Pts',(21.4493936375027,11.3814773557988,-0.39552765226469));
#66696=CARTESIAN_POINT('Ctrl Pts',(21.5684577603519,10.1842693168954,5.09657997143273));
#66697=CARTESIAN_POINT('Ctrl Pts',(21.6875218832011,6.50593921983901,9.34704358564926));
#66698=CARTESIAN_POINT('Ctrl Pts',(21.8065860060503,1.24261281081684,11.3203525707754));
#66699=CARTESIAN_POINT('Ctrl Pts',(21.9256501288995,-4.3234426363649,10.5357635078967));
#66700=CARTESIAN_POINT('Ctrl Pts',(22.0447142517487,-8.83620809695444,7.18442032397769));
#66701=CARTESIAN_POINT('Ctrl Pts',(22.1637783745979,-11.1962701934044,2.0827872384264));
#66702=CARTESIAN_POINT('Ctrl Pts',(22.2828424974471,-10.82866356061,-3.52626068454731));
#66703=CARTESIAN_POINT('Ctrl Pts',(22.4019066202962,-7.82294562257201,-8.27623046504554));
#66704=CARTESIAN_POINT('Ctrl Pts',(22.5209707431455,-2.91137834572138,-11.0099203018156));
#66705=CARTESIAN_POINT('Ctrl Pts',(22.6400348659946,2.70946760478089,-11.0613405255832));
#66706=CARTESIAN_POINT('Ctrl Pts',(22.7590989888438,7.67022497839136,-8.41796398811068));
#66707=CARTESIAN_POINT('Ctrl Pts',(22.878163111693,10.7623392719026,-3.72377796340366));
#66708=CARTESIAN_POINT('Ctrl Pts',(22.9972272345422,11.2325003811489,1.87760595220527));
#66709=CARTESIAN_POINT('Ctrl Pts',(23.1162913573914,8.96616625478253,7.0215619071447));
#66710=CARTESIAN_POINT('Ctrl Pts',(23.2353554802406,4.51546797036092,10.4549040135676));
#66711=CARTESIAN_POINT('Ctrl Pts',(23.3544196030898,-1.03530208509686,11.3411912300631));
#66712=CARTESIAN_POINT('Ctrl Pts',(23.473483725939,-6.33384875954844,9.46450362224209));
#66713=CARTESIAN_POINT('Ctrl Pts',(23.5925478487882,-10.0893243131047,5.2820454209767));
#66714=CARTESIAN_POINT('Ctrl Pts',(23.7116119716373,-11.3868085934357,-0.187240435603125));
#66715=CARTESIAN_POINT('Ctrl Pts',(23.8306760944865,-9.9102046113648,-5.61091021895294));
#66716=CARTESIAN_POINT('Ctrl Pts',(23.9497402173357,-6.01924703190071,-9.66763332430542));
#66717=CARTESIAN_POINT('Ctrl Pts',(24.0688043401849,-0.661862542501585,
-11.3690987725105));
#66718=CARTESIAN_POINT('Ctrl Pts',(24.1878684630341,4.85676687302519,-10.300790477694));
#66719=CARTESIAN_POINT('Ctrl Pts',(24.3069325858833,9.19217626117312,-6.72297289209112));
#66720=CARTESIAN_POINT('Ctrl Pts',(24.4259967087325,11.2881602595985,-1.50728460414338));
#66721=CARTESIAN_POINT('Ctrl Pts',(24.5450608315817,10.6340889968582,4.07561285344499));
#66722=CARTESIAN_POINT('Ctrl Pts',(24.6641249544309,7.38930926427251,8.66559735512809));
#66723=CARTESIAN_POINT('Ctrl Pts',(24.78318907728,2.34432397548791,11.1444431903177));
#66724=CARTESIAN_POINT('Ctrl Pts',(24.9022532001293,-3.27179251044516,10.9082465452914));
#66725=CARTESIAN_POINT('Ctrl Pts',(25.0213173229785,-8.09082514924365,8.01455035099494));
#66726=CARTESIAN_POINT('Ctrl Pts',(25.1403814458276,-10.9387468401859,3.16832550262579));
#66727=CARTESIAN_POINT('Ctrl Pts',(25.2594455686768,-11.121738409071,-2.44977625191787));
#66728=CARTESIAN_POINT('Ctrl Pts',(25.378509691526,-8.59521890424802,-7.47105621129462));
#66729=CARTESIAN_POINT('Ctrl Pts',(25.4975738143752,-3.97470654098743,-10.6722151794882));
#66730=CARTESIAN_POINT('Ctrl Pts',(25.6166379372244,1.61413568145801,-11.2733772635405));
#66731=CARTESIAN_POINT('Ctrl Pts',(25.7357020600736,6.80973735620175,-9.12808556400613));
#66732=CARTESIAN_POINT('Ctrl Pts',(25.8547661829228,10.3463305111421,-4.75898244149697));
#66733=CARTESIAN_POINT('Ctrl Pts',(25.973830305772,11.3623197765575,0.769518173611109));
#66734=CARTESIAN_POINT('Ctrl Pts',(26.0928944286212,9.61018681815882,6.11054647673616));
#66735=CARTESIAN_POINT('Ctrl Pts',(26.2119585514704,5.51679149173258,9.96290522694128));
#66736=CARTESIAN_POINT('Ctrl Pts',(26.3310226743196,0.0793789722749223,
11.3880712986452));
#66737=CARTESIAN_POINT('Ctrl Pts',(26.4500867971688,-5.37737208909836,10.0388414839389));
#66738=CARTESIAN_POINT('Ctrl Pts',(26.5691509200179,-9.52407172802688,6.24391917337703));
#66739=CARTESIAN_POINT('Ctrl Pts',(26.6882150428671,-11.3504886139613,0.927834655852592));
#66740=CARTESIAN_POINT('Ctrl Pts',(26.8072791657163,-10.4116656191913,-4.61429170712224));
#66741=CARTESIAN_POINT('Ctrl Pts',(26.9263432885655,-6.93632160105888,-9.03227056564133));
#66742=CARTESIAN_POINT('Ctrl Pts',(27.0454074114147,-1.77113023194562,-11.2497807367857));
#66743=CARTESIAN_POINT('Ctrl Pts',(27.1644715342639,3.8255491653811,-10.726585780551));
#66744=CARTESIAN_POINT('Ctrl Pts',(27.2835356571131,8.49023686812152,-7.59014801222325));
#66745=CARTESIAN_POINT('Ctrl Pts',(27.4025997799623,11.086507749098,-2.60457575306547));
#66746=CARTESIAN_POINT('Ctrl Pts',(27.5216639028115,10.9818505547988,3.0155310173057));
#66747=CARTESIAN_POINT('Ctrl Pts',(27.6407280256606,8.20176218296288,7.90098512961429));
#66748=CARTESIAN_POINT('Ctrl Pts',(27.7597921485099,3.42353605232723,10.8615776857086));
#66749=CARTESIAN_POINT('Ctrl Pts',(27.8788562713591,-2.18874213958099,11.1760402992603));
#66750=CARTESIAN_POINT('Ctrl Pts',(27.9979203942083,-7.26779244511403,8.76776265069999));
#66751=CARTESIAN_POINT('Ctrl Pts',(28.1169845170574,-10.576241484267,4.2234565217054));
#66752=CARTESIAN_POINT('Ctrl Pts',(28.2360486399066,-11.3080750370802,-1.34978067849222));
#66753=CARTESIAN_POINT('Ctrl Pts',(28.3551127627558,-9.28500163125622,-6.59418028505711));
#66754=CARTESIAN_POINT('Ctrl Pts',(28.474176885605,-4.999888442266,-10.232086028233));
#66755=CARTESIAN_POINT('Ctrl Pts',(28.5932410084542,0.503312477557374,-11.3772204634613));
#66756=CARTESIAN_POINT('Ctrl Pts',(28.7123051313034,5.88389491083505,-9.7506025251015));
#66757=CARTESIAN_POINT('Ctrl Pts',(28.8313692541526,9.83102532150094,-5.7485137255011));
#66758=CARTESIAN_POINT('Ctrl Pts',(28.9504333770018,11.3830920294648,-0.34595487133575));
#66759=CARTESIAN_POINT('Ctrl Pts',(29.069497499851,10.1619759154233,5.14088654014301));
#66760=CARTESIAN_POINT('Ctrl Pts',(29.1885616227001,6.46516892816917,9.37528984375964));
#66761=CARTESIAN_POINT('Ctrl Pts',(29.3076257455494,1.19329820897357,11.325657080661));
#66762=CARTESIAN_POINT('Ctrl Pts',(29.4266898683985,-4.36928737803557,10.5168339690425));
#66763=CARTESIAN_POINT('Ctrl Pts',(29.5457539912477,-8.86741414578814,7.14586840708276));
#66764=CARTESIAN_POINT('Ctrl Pts',(29.664818114097,-11.2052350387348,2.03400507643787));
#66765=CARTESIAN_POINT('Ctrl Pts',(29.7838822369461,-10.8132031600868,-3.57338863586859));
#66766=CARTESIAN_POINT('Ctrl Pts',(29.9029463597953,-7.78682648506999,-8.31022275367388));
#66767=CARTESIAN_POINT('Ctrl Pts',(30.0220104826445,-2.86339992321776,-11.0224956250381));
#66768=CARTESIAN_POINT('Ctrl Pts',(30.1410746054937,2.75761666593505,-11.0494352456595));
#66769=CARTESIAN_POINT('Ctrl Pts',(30.2601387283429,7.70681446034808,-8.38447850483479));
#66770=CARTESIAN_POINT('Ctrl Pts',(30.3792028511921,10.7784551359661,-3.67687011005731));
#66771=CARTESIAN_POINT('Ctrl Pts',(30.4982669740413,11.2242164324623,1.92650834452133));
#66772=CARTESIAN_POINT('Ctrl Pts',(30.6173310968905,8.93550065362564,7.06054509179871));
#66773=CARTESIAN_POINT('Ctrl Pts',(30.7363952197397,4.46989156192526,10.4744707908751));
#66774=CARTESIAN_POINT('Ctrl Pts',(30.8554593425888,-1.08468584028973,11.3365746833928));
#66775=CARTESIAN_POINT('Ctrl Pts',(30.9745234654381,-6.37500884380716,9.4368284484591));
#66776=CARTESIAN_POINT('Ctrl Pts',(31.0935875882872,-10.1122331839721,5.23805392843931));
#66777=CARTESIAN_POINT('Ctrl Pts',(31.2126517111365,-11.3858851234823,-0.236830908310294));
#66778=CARTESIAN_POINT('Ctrl Pts',(31.3317158339856,-9.88567377909413,-5.65401829300169));
#66779=CARTESIAN_POINT('Ctrl Pts',(31.4507799568348,-5.97708511181582,-9.69375688215753));
#66780=CARTESIAN_POINT('Ctrl Pts',(31.569844079684,-0.612341147290723,-11.3718735151074));
#66781=CARTESIAN_POINT('Ctrl Pts',(31.6889082025332,4.90158319339904,-10.2795404139706));
#66782=CARTESIAN_POINT('Ctrl Pts',(31.8079723253824,9.22136922110839,-6.68287502593459));
#66783=CARTESIAN_POINT('Ctrl Pts',(31.9270364482316,11.2946177831492,-1.45810769726966));
#66784=CARTESIAN_POINT('Ctrl Pts',(32.0461005710808,10.616237882882,4.12188817634924));
#66785=CARTESIAN_POINT('Ctrl Pts',(32.16516469393,7.35149845438419,8.69769736191447));
#66786=CARTESIAN_POINT('Ctrl Pts',(32.2842288167791,2.29576505193558,11.1545475816179));
#66787=CARTESIAN_POINT('Ctrl Pts',(32.4032929396284,-3.31926947791388,10.8938936591678));
#66788=CARTESIAN_POINT('Ctrl Pts',(32.5223570624775,-8.12565368024842,7.97923688036213));
#66789=CARTESIAN_POINT('Ctrl Pts',(32.6414211853267,-10.9524419041528,3.12065462049613));
#66790=CARTESIAN_POINT('Ctrl Pts',(32.7604853081759,-11.1109635736809,-2.49819082309636));
#66791=CARTESIAN_POINT('Ctrl Pts',(32.8795494310251,-8.5625991670266,-7.50841956933033));
#66792=CARTESIAN_POINT('Ctrl Pts',(32.9986135538743,-3.92818881958114,-10.6894247516873));
#66793=CARTESIAN_POINT('Ctrl Pts',(33.1176776767235,1.66321860105479,-11.2662404026087));
#66794=CARTESIAN_POINT('Ctrl Pts',(33.2367417995727,6.84942774676265,-9.09834097328428));
#66795=CARTESIAN_POINT('Ctrl Pts',(33.3558059224219,10.3669588813711,-4.71387658686845));
#66796=CARTESIAN_POINT('Ctrl Pts',(33.4748700452711,11.3588605813904,0.818996469346493));
#66797=CARTESIAN_POINT('Ctrl Pts',(33.5939341681202,9.58348279703671,6.15234316363844));
#66798=CARTESIAN_POINT('Ctrl Pts',(33.7129982909695,5.47334835790634,9.98683767151899));
#66799=CARTESIAN_POINT('Ctrl Pts',(33.8320624138186,0.0297804715449969,
11.3883090073892));
#66800=CARTESIAN_POINT('Ctrl Pts',(33.9511265366678,-5.4210426220926,10.0153265455362));
#66801=CARTESIAN_POINT('Ctrl Pts',(34.070190659517,-9.55117514782195,6.20238036723762));
#66802=CARTESIAN_POINT('Ctrl Pts',(34.1892547823662,-11.3544219046106,0.878391789787302));
#66803=CARTESIAN_POINT('Ctrl Pts',(34.3083189052154,-10.3914705406985,-4.65959321465532));
#66804=CARTESIAN_POINT('Ctrl Pts',(34.4273830280646,-6.89691813866351,-9.06239422629812));
#66805=CARTESIAN_POINT('Ctrl Pts',(34.5464471509138,-1.72211797464862,-11.257387734535));
#66806=CARTESIAN_POINT('Ctrl Pts',(34.665511273763,3.87222970531349,-10.7098228759188));
#66807=CARTESIAN_POINT('Ctrl Pts',(34.7845753966122,8.52321323836035,-7.55309903401944));
#66808=CARTESIAN_POINT('Ctrl Pts',(34.9036395194613,11.0977461479978,-2.55626668383156));
#66809=CARTESIAN_POINT('Ctrl Pts',(35.0227036423106,10.9686130501091,3.06333097807638));
#66810=CARTESIAN_POINT('Ctrl Pts',(35.1417677651597,8.16727373504748,7.9366308129502));
#66811=CARTESIAN_POINT('Ctrl Pts',(35.260831888009,3.37619883970387,10.876384983948));
#66812=CARTESIAN_POINT('Ctrl Pts',(35.3798960108581,-2.23739568402404,11.166401814254));
#66813=CARTESIAN_POINT('Ctrl Pts',(35.4989601337073,-7.30590919980583,8.73602653890538));
#66814=CARTESIAN_POINT('Ctrl Pts',(35.6180242565565,-10.5945353317742,4.17735442930754));
#66815=CARTESIAN_POINT('Ctrl Pts',(35.7370883794057,-11.3020891757249,-1.39901722227757));
#66816=CARTESIAN_POINT('Ctrl Pts',(35.856152502255,-9.25619435443022,-6.63455612662077));
#66817=CARTESIAN_POINT('Ctrl Pts',(35.9752166251041,-4.95527786464635,-10.2537646846615));
#66818=CARTESIAN_POINT('Ctrl Pts',(36.0942807479533,0.552858194032231,-11.3749205158347));
#66819=CARTESIAN_POINT('Ctrl Pts',(36.2133448708025,5.92630529098352,-9.72488429351872));
#66820=CARTESIAN_POINT('Ctrl Pts',(36.3324089936517,9.85596822205322,-5.70564276222618));
#66821=CARTESIAN_POINT('Ctrl Pts',(36.4514731165008,11.3844907866144,-0.296375528273049));
#66822=CARTESIAN_POINT('Ctrl Pts',(36.5705372393501,10.1394897597824,5.18509559560226));
#66823=CARTESIAN_POINT('Ctrl Pts',(36.6896013621993,6.42427600402371,9.403358269703));
#66824=CARTESIAN_POINT('Ctrl Pts',(36.8086654850484,1.14396097243734,11.3307467634665));
#66825=CARTESIAN_POINT('Ctrl Pts',(36.9277296078976,-4.41504924228522,10.4977049450088));
#66826=CARTESIAN_POINT('Ctrl Pts',(37.0467937307468,-8.89845199593134,7.10718094608351));
#66827=CARTESIAN_POINT('Ctrl Pts',(37.165857853596,-11.213987341172,1.9851843330787));
#66828=CARTESIAN_POINT('Ctrl Pts',(37.2849219764453,-10.7975376528006,-3.62044880651819));
#66829=CARTESIAN_POINT('Ctrl Pts',(37.4039860992944,-7.75055964565652,-8.34405741251745));
#66830=CARTESIAN_POINT('Ctrl Pts',(37.5230502221436,-2.81536718723445,-11.0348618716008));
#66831=CARTESIAN_POINT('Ctrl Pts',(37.6421143449928,2.8057134201252,-11.0373203780807));
#66832=CARTESIAN_POINT('Ctrl Pts',(37.761178467842,7.74325775807585,-8.35083398327767));
#66833=CARTESIAN_POINT('Ctrl Pts',(37.8802425906911,10.7943665523734,-3.62989251318388));
#66834=CARTESIAN_POINT('Ctrl Pts',(37.9993067135404,11.2157195808398,1.97537419448435));
#66835=CARTESIAN_POINT('Ctrl Pts',(38.1183708363895,8.9046655623011,7.09939435077635));
#66836=CARTESIAN_POINT('Ctrl Pts',(38.2374349592387,4.42423036779067,10.4938388865555));
#66837=CARTESIAN_POINT('Ctrl Pts',(38.3564990820879,-1.13404902096795,11.3317431025552));
#66838=CARTESIAN_POINT('Ctrl Pts',(38.4755632049371,-6.41604800576263,9.40897427523404));
#66839=CARTESIAN_POINT('Ctrl Pts',(38.5946273277863,-10.1349502442,5.19396307956243));
#66840=CARTESIAN_POINT('Ctrl Pts',(38.7136914506355,-11.3847456840324,-0.286416888766937));
#66841=CARTESIAN_POINT('Ctrl Pts',(38.8327555734847,-9.86095543360296,-5.6970191206248));
#66842=CARTESIAN_POINT('Ctrl Pts',(38.9518196963339,-5.9348098173161,-9.71969656710295));
#66843=CARTESIAN_POINT('Ctrl Pts',(39.0708838191831,-0.562808137084897,
-11.3744325539824));
#66844=CARTESIAN_POINT('Ctrl Pts',(39.1899479420323,4.94630653967062,-10.2580953660947));
#66845=CARTESIAN_POINT('Ctrl Pts',(39.3090120648815,9.25038726846866,-6.64265039781417));
#66846=CARTESIAN_POINT('Ctrl Pts',(39.4280761877307,11.3008610683819,-1.40890313275033));
#66847=CARTESIAN_POINT('Ctrl Pts',(39.5471403105798,10.5981853982089,4.16808531454696));
#66848=CARTESIAN_POINT('Ctrl Pts',(39.666204433429,7.31354819997646,8.72963238922423));
#66849=CARTESIAN_POINT('Ctrl Pts',(39.7852685562782,2.2471625818798,11.1644403914813));
#66850=CARTESIAN_POINT('Ctrl Pts',(39.9043326791274,-3.36668348484207,10.879334135714));
#66851=CARTESIAN_POINT('Ctrl Pts',(40.0233968019766,-8.16032808249549,7.94377205817354));
#66852=CARTESIAN_POINT('Ctrl Pts',(40.1424609248258,-10.9659292200814,3.07292454517561));
#66853=CARTESIAN_POINT('Ctrl Pts',(40.261525047675,-11.099977983884,-2.54655800803447));
#66854=CARTESIAN_POINT('Ctrl Pts',(40.3805891705242,-8.52981701226451,-7.54564050654328));
#66855=CARTESIAN_POINT('Ctrl Pts',(40.4996532933734,-3.88159658881691,-10.7064315645553));
#66856=CARTESIAN_POINT('Ctrl Pts',(40.6187174162226,1.71226997479381,-11.2588898424318));
#66857=CARTESIAN_POINT('Ctrl Pts',(40.7377815390717,6.88898821158214,-9.06842380204854));
#66858=CARTESIAN_POINT('Ctrl Pts',(40.856845661921,10.3873906181177,-4.66868132160697));
#66859=CARTESIAN_POINT('Ctrl Pts',(40.9759097847701,11.3551859122596,0.868459236040161));
#66860=CARTESIAN_POINT('Ctrl Pts',(41.0949739076193,9.55659702768504,6.19402314054106));
#66861=CARTESIAN_POINT('Ctrl Pts',(41.2140380304685,5.42980134093462,10.0105807057282));
#66862=CARTESIAN_POINT('Ctrl Pts',(41.3331021533178,-0.0198184710268861,
11.3883306586547));
#66863=CARTESIAN_POINT('Ctrl Pts',(41.4521662761669,-5.46461056544047,9.99162171577145));
#66864=CARTESIAN_POINT('Ctrl Pts',(41.5712303990161,-9.57809694018392,6.16072375652635));
#66865=CARTESIAN_POINT('Ctrl Pts',(41.6902945218653,-11.3581407092251,0.828932564934985));
#66866=CARTESIAN_POINT('Ctrl Pts',(41.8093586447145,-10.3710766423138,-4.7048069228834));
#66867=CARTESIAN_POINT('Ctrl Pts',(41.9284227675637,-6.8573871623192,-9.09234486049293));
#66868=CARTESIAN_POINT('Ctrl Pts',(42.0474868904129,-1.67306666230694,-11.264783381553));
#66869=CARTESIAN_POINT('Ctrl Pts',(42.1665510132621,3.91882445422349,-10.6928526119433));
#66870=CARTESIAN_POINT('Ctrl Pts',(42.2856151361112,8.55605177827666,-7.51591492621075));
#66871=CARTESIAN_POINT('Ctrl Pts',(42.4046792589605,11.1087279900831,-2.50789340307738));
#66872=CARTESIAN_POINT('Ctrl Pts',(42.5237433818096,10.9552564987174,3.11104243197162));
#66873=CARTESIAN_POINT('Ctrl Pts',(42.6428075046589,8.13245791718728,7.97218496166449));
#66874=CARTESIAN_POINT('Ctrl Pts',(42.7618716275081,3.32913578666725,10.8908692226323));
#66875=CARTESIAN_POINT('Ctrl Pts',(42.8809357503572,-2.28670921768049,11.1568037777588));
#66876=CARTESIAN_POINT('Ctrl Pts',(42.9603118322567,-5.656950401196,9.52119826328445));
#66877=CARTESIAN_POINT('Ctrl Pts',(42.9999998732064,-7.04509306938772,8.34998763126076));
#66878=CARTESIAN_POINT('Ctrl Pts',(-0.174507299781054,-10.4337367209092,
2.08233076243301));
#66879=CARTESIAN_POINT('Ctrl Pts',(-0.134819258831324,-10.7799135427525,
0.347775482764217));
#66880=CARTESIAN_POINT('Ctrl Pts',(-0.0554431769318622,-10.5901942492717,
-3.2955529604118));
#66881=CARTESIAN_POINT('Ctrl Pts',(0.063620945917329,-7.72290813945365,
-7.95995680930942));
#66882=CARTESIAN_POINT('Ctrl Pts',(0.182685068766521,-2.97527511676106,
-10.6841222833608));
#66883=CARTESIAN_POINT('Ctrl Pts',(0.301749191615713,2.49776047340013,-10.8058947680803));
#66884=CARTESIAN_POINT('Ctrl Pts',(0.420813314464905,7.36199869358438,-8.29484351599949));
#66885=CARTESIAN_POINT('Ctrl Pts',(0.539877437314096,10.4328323523309,-3.76311187175351));
#66886=CARTESIAN_POINT('Ctrl Pts',(0.658941560163288,10.9619119467463,1.68546972306047));
#66887=CARTESIAN_POINT('Ctrl Pts',(0.77800568301248,8.82045738536265,6.72339622249938));
#66888=CARTESIAN_POINT('Ctrl Pts',(0.897069805861671,4.53011623594228,10.123367491015));
#66889=CARTESIAN_POINT('Ctrl Pts',(1.01613392871086,-0.863854746543476,
11.0570441539293));
#66890=CARTESIAN_POINT('Ctrl Pts',(1.13519805156006,-6.04737634360005,9.29697573708195));
#66891=CARTESIAN_POINT('Ctrl Pts',(1.25426217440925,-9.75761524488855,5.27194778803861));
#66892=CARTESIAN_POINT('Ctrl Pts',(1.37332629725844,-11.0906762950597,-0.0374464642950963));
#66893=CARTESIAN_POINT('Ctrl Pts',(1.49239042010763,-9.72179295539908,-5.33771858931385));
#66894=CARTESIAN_POINT('Ctrl Pts',(1.61145454295682,-5.98445782173597,-9.33759943749471));
#66895=CARTESIAN_POINT('Ctrl Pts',(1.73051866580601,-0.789171025288819,
-11.0626266535911));
#66896=CARTESIAN_POINT('Ctrl Pts',(1.8495827886552,4.59837586387181,-10.0925436820845));
#66897=CARTESIAN_POINT('Ctrl Pts',(1.9686469115044,8.86565276843565,-6.66368517479524));
#66898=CARTESIAN_POINT('Ctrl Pts',(2.08771103435359,10.9730528818932,-1.61139978989388));
#66899=CARTESIAN_POINT('Ctrl Pts',(2.20677515720278,10.4071651477731,3.83345960332373));
#66900=CARTESIAN_POINT('Ctrl Pts',(2.32583928005197,7.30585280097071,8.34440014437491));
#66901=CARTESIAN_POINT('Ctrl Pts',(2.44490340290116,2.42466681433469,10.8224530375817));
#66902=CARTESIAN_POINT('Ctrl Pts',(2.56396752575036,-3.04722373344697,10.6639076535324));
#66903=CARTESIAN_POINT('Ctrl Pts',(2.68303164859955,-7.7767405481066,7.90738928862895));
#66904=CARTESIAN_POINT('Ctrl Pts',(2.80209577144874,-10.6116646425128,3.2244491676919));
#66905=CARTESIAN_POINT('Ctrl Pts',(2.92115989429793,-10.8613433548614,-2.24404087430769));
#66906=CARTESIAN_POINT('Ctrl Pts',(3.04022401714713,-8.46494921319319,-7.16583098715693));
#66907=CARTESIAN_POINT('Ctrl Pts',(3.15928813999631,-4.0062989035811,-10.3418599881082));
#66908=CARTESIAN_POINT('Ctrl Pts',(3.27835226284551,1.42837789075295,-10.9983742216505));
#66909=CARTESIAN_POINT('Ctrl Pts',(3.3974163856947,6.51506900426455,-8.97543173268633));
#66910=CARTESIAN_POINT('Ctrl Pts',(3.51648050854389,10.0145395804952,-4.76586780230288));
#66911=CARTESIAN_POINT('Ctrl Pts',(3.63554463139308,11.0742381630554,0.60477105280474));
#66912=CARTESIAN_POINT('Ctrl Pts',(3.75460875424228,9.43599782347387,5.82807378074111));
#66913=CARTESIAN_POINT('Ctrl Pts',(3.87367287709146,5.49893155814324,9.63152379622371));
#66914=CARTESIAN_POINT('Ctrl Pts',(3.99273699994066,0.222199190055808,11.0885132654612));
#66915=CARTESIAN_POINT('Ctrl Pts',(4.11180112278985,-5.10866600726,9.8440860695462));
#66916=CARTESIAN_POINT('Ctrl Pts',(4.23086524563904,-9.1949427590091,6.20141327254646));
#66917=CARTESIAN_POINT('Ctrl Pts',(4.34992936848823,-11.0411201385837,1.04793368288726));
#66918=CARTESIAN_POINT('Ctrl Pts',(4.46899349133742,-10.1974269078917,-4.3608466352964));
#66919=CARTESIAN_POINT('Ctrl Pts',(4.58805761418662,-6.86940612749505,-8.70722449313797));
#66920=CARTESIAN_POINT('Ctrl Pts',(4.7071217370358,-1.86784014331401,-10.9323223570014));
#66921=CARTESIAN_POINT('Ctrl Pts',(4.826185859885,3.58877462605504,-10.4940552505574));
#66922=CARTESIAN_POINT('Ctrl Pts',(4.94524998273419,8.17108142011614,-7.49919511309055));
#66923=CARTESIAN_POINT('Ctrl Pts',(5.06431410558339,10.7627249943052,-2.67735870128112));
#66924=CARTESIAN_POINT('Ctrl Pts',(5.18337822843257,10.7323214133876,2.79674382060814));
#66925=CARTESIAN_POINT('Ctrl Pts',(5.30244235128177,8.087277688403,7.58949527366791));
#66926=CARTESIAN_POINT('Ctrl Pts',(5.42150647413096,3.47198725854995,10.5332712580107));
#66927=CARTESIAN_POINT('Ctrl Pts',(5.54057059698015,-1.98915905990607,10.9109002906617));
#66928=CARTESIAN_POINT('Ctrl Pts',(5.65963471982934,-6.9657005169686,8.63038326068267));
#66929=CARTESIAN_POINT('Ctrl Pts',(5.77869884267854,-10.2452372439552,4.24730652689935));
#66930=CARTESIAN_POINT('Ctrl Pts',(5.89776296552772,-11.028798724606,-1.17051168746773));
#66931=CARTESIAN_POINT('Ctrl Pts',(6.01682708837692,-9.12549137460288,-6.3031663543347));
#66932=CARTESIAN_POINT('Ctrl Pts',(6.13589121122611,-4.99900460578266,-9.9002248393525));
#66933=CARTESIAN_POINT('Ctrl Pts',(6.2549553340753,0.345354570991203,-11.0853610287922));
#66934=CARTESIAN_POINT('Ctrl Pts',(6.37401945692449,5.60557743741153,-9.56984851037628));
#66935=CARTESIAN_POINT('Ctrl Pts',(6.49308357977368,9.5001528139748,-5.72290096275441));
#66936=CARTESIAN_POINT('Ctrl Pts',(6.61214770262288,11.0802726347061,-0.481723218199343));
#66937=CARTESIAN_POINT('Ctrl Pts',(6.73121182547206,9.96098339732145,4.87681337316233));
#66938=CARTESIAN_POINT('Ctrl Pts',(6.85027594832127,6.41496968329811,9.04724614900771));
#66939=CARTESIAN_POINT('Ctrl Pts',(6.96934007117045,1.30612192705152,11.0135618412048));
#66940=CARTESIAN_POINT('Ctrl Pts',(7.08840419401965,-4.12092714762138,10.2967207577153));
#66941=CARTESIAN_POINT('Ctrl Pts',(7.20746831686883,-8.54402366292485,7.0713618607556));
#66942=CARTESIAN_POINT('Ctrl Pts',(7.32653243971803,-10.8855996571344,2.12325670208844));
#66943=CARTESIAN_POINT('Ctrl Pts',(7.44559656256721,-10.5751934044946,-3.34212258540929));
#66944=CARTESIAN_POINT('Ctrl Pts',(7.56466068541642,-7.68842700183419,-7.99328400320142));
#66945=CARTESIAN_POINT('Ctrl Pts',(7.6837248082656,-2.92858308784915,-10.6970977379817));
#66946=CARTESIAN_POINT('Ctrl Pts',(7.80278893111479,2.54473097036526,-10.7948526255263));
#66947=CARTESIAN_POINT('Ctrl Pts',(7.92185305396399,7.3980900817713,-8.26273332864893));
#66948=CARTESIAN_POINT('Ctrl Pts',(8.04091717681317,10.449104428037,-3.71762230065761));
#66949=CARTESIAN_POINT('Ctrl Pts',(8.15998129966237,10.9544767966953,1.73318695732269));
#66950=CARTESIAN_POINT('Ctrl Pts',(8.27904542251157,8.79108686438842,6.76175204079136));
#66951=CARTESIAN_POINT('Ctrl Pts',(8.39810954536075,4.48598613716095,10.1429989300782));
#66952=CARTESIAN_POINT('Ctrl Pts',(8.51717366820995,-0.912003908990337,
11.0531781759074));
#66953=CARTESIAN_POINT('Ctrl Pts',(8.63623779105913,-6.08780884344555,9.27054919646268));
#66954=CARTESIAN_POINT('Ctrl Pts',(8.75530191390834,-9.78048363500147,5.22940137910996));
#66955=CARTESIAN_POINT('Ctrl Pts',(8.87436603675751,-11.0904078402242,-0.0857487951051246));
#66956=CARTESIAN_POINT('Ctrl Pts',(8.99343015960672,-9.69845381834187,-5.38000859217331));
#66957=CARTESIAN_POINT('Ctrl Pts',(9.1124942824559,-5.94373355865523,-9.36357465405622));
#66958=CARTESIAN_POINT('Ctrl Pts',(9.23155840530509,-0.740983206549613,
-11.0659587386715));
#66959=CARTESIAN_POINT('Ctrl Pts',(9.35062252815429,4.64228768377877,-10.0724209592036));
#66960=CARTESIAN_POINT('Ctrl Pts',(9.46968665100347,8.89459060634068,-6.62500995198986));
#66961=CARTESIAN_POINT('Ctrl Pts',(9.58875077385267,10.9799668437429,-1.56359426600191));
#66962=CARTESIAN_POINT('Ctrl Pts',(9.70781489670186,10.3903708189128,3.87874891735133));
#66963=CARTESIAN_POINT('Ctrl Pts',(9.82687901955106,7.26944167346037,8.37613972391375));
#66964=CARTESIAN_POINT('Ctrl Pts',(9.94594314240024,2.37750947170057,10.8329103951959));
#66965=CARTESIAN_POINT('Ctrl Pts',(10.0650072652494,-3.09363867674658,10.6505351347294));
#66966=CARTESIAN_POINT('Ctrl Pts',(10.1840713880986,-7.81110534623898,7.87344474727075));
#66967=CARTESIAN_POINT('Ctrl Pts',(10.3031355109478,-10.6256072403439,3.17820227366338));
#66968=CARTESIAN_POINT('Ctrl Pts',(10.422199633797,-10.8514670154161,-2.291323314529));
#66969=CARTESIAN_POINT('Ctrl Pts',(10.5412637566462,-8.43366003959012,-7.20262988463169));
#66970=CARTESIAN_POINT('Ctrl Pts',(10.6603278794954,-3.96121965766618,-10.3592102856389));
#66971=CARTESIAN_POINT('Ctrl Pts',(10.7793920023446,1.47626486871297,-10.9920489880537));
#66972=CARTESIAN_POINT('Ctrl Pts',(10.8984561251938,6.55409734589077,-8.94697194021287));
#66973=CARTESIAN_POINT('Ctrl Pts',(11.017520248043,10.0352010848374,-4.72220691046526));
#66974=CARTESIAN_POINT('Ctrl Pts',(11.1365843708922,11.0714992128125,0.652996247355111));
#66975=CARTESIAN_POINT('Ctrl Pts',(11.2556484937414,9.4105256898738,5.8691145123088));
#66976=CARTESIAN_POINT('Ctrl Pts',(11.3747126165905,5.45693183832424,9.65538159941137));
#66977=CARTESIAN_POINT('Ctrl Pts',(11.4937767394398,0.173903980994529,11.0893758311171));
#66978=CARTESIAN_POINT('Ctrl Pts',(11.6128408622889,-5.15149088272712,9.82174325685352));
#66979=CARTESIAN_POINT('Ctrl Pts',(11.7319049851381,-9.22186417702655,6.16130830415449));
#66980=CARTESIAN_POINT('Ctrl Pts',(11.8509691079873,-11.0455794230206,0.999837050779577));
#66981=CARTESIAN_POINT('Ctrl Pts',(11.9700332308365,-10.1783376745769,-4.40521748619256));
#66982=CARTESIAN_POINT('Ctrl Pts',(12.0890973536857,-6.83141895236856,-8.73705980382349));
#66983=CARTESIAN_POINT('Ctrl Pts',(12.2081614765349,-1.82020957524915,-10.940353560125));
#66984=CARTESIAN_POINT('Ctrl Pts',(12.3272255993841,3.63444468604277,-10.4783257604669));
#66985=CARTESIAN_POINT('Ctrl Pts',(12.4462897222333,8.20366469583483,-7.46353699506351));
#66986=CARTESIAN_POINT('Ctrl Pts',(12.5653538450825,10.7742834509684,-2.63045909235571));
#66987=CARTESIAN_POINT('Ctrl Pts',(12.6844179679317,10.7200391453183,2.84345909786154));
#66988=CARTESIAN_POINT('Ctrl Pts',(12.8034820907808,8.05414693837119,7.62464530411053));
#66989=CARTESIAN_POINT('Ctrl Pts',(12.92254621363,3.42607943866673,10.5482926864168));
#66990=CARTESIAN_POINT('Ctrl Pts',(13.0416103364792,-2.03665974967412,10.9021335518524));
#66991=CARTESIAN_POINT('Ctrl Pts',(13.1606744593284,-7.00322181694395,8.59996413370713));
#66992=CARTESIAN_POINT('Ctrl Pts',(13.2797385821776,-10.2636381031578,4.20264581017423));
#66993=CARTESIAN_POINT('Ctrl Pts',(13.3988027050268,-11.0235962708498,-1.21853361696568));
#66994=CARTESIAN_POINT('Ctrl Pts',(13.517866827876,-9.09795304518452,-6.34285025095079));
#66995=CARTESIAN_POINT('Ctrl Pts',(13.6369309507252,-4.95583937062804,-9.92190279386475));
#66996=CARTESIAN_POINT('Ctrl Pts',(13.7559950735744,0.393630668584838,-11.0837517932836));
#66997=CARTESIAN_POINT('Ctrl Pts',(13.8750591964236,5.64720323060015,-9.54534413159986));
#66998=CARTESIAN_POINT('Ctrl Pts',(13.9941233192728,9.52498730290309,-5.68147127053403));
#66999=CARTESIAN_POINT('Ctrl Pts',(14.1131874421219,11.0822655671305,-0.433461437687701));
#67000=CARTESIAN_POINT('Ctrl Pts',(14.2322515649712,9.93964924910235,4.92014956309131));
#67001=CARTESIAN_POINT('Ctrl Pts',(14.3513156878203,6.37550594323823,9.07509905654491));
#67002=CARTESIAN_POINT('Ctrl Pts',(14.4703798106695,1.25814286917611,11.0191458579651));
#67003=CARTESIAN_POINT('Ctrl Pts',(14.5894439335187,-4.1657327221702,10.2786754888852));
#67004=CARTESIAN_POINT('Ctrl Pts',(14.7085080563679,-8.57474008647537,7.03408354853429));
#67005=CARTESIAN_POINT('Ctrl Pts',(14.8275721792171,-10.8947437029919,2.07582720005479));
#67006=CARTESIAN_POINT('Ctrl Pts',(14.9466363020663,-10.5605373729417,-3.3881483605458));
#67007=CARTESIAN_POINT('Ctrl Pts',(15.0657004249155,-7.65354143897896,-8.02669311486371));
#67008=CARTESIAN_POINT('Ctrl Pts',(15.1847645477647,-2.88196691853509,-10.7097509587683));
#67009=CARTESIAN_POINT('Ctrl Pts',(15.3038286706139,2.59172097597115,-10.7836673400602));
#67010=CARTESIAN_POINT('Ctrl Pts',(15.422892793463,7.43400607838975,-8.23043452952715));
#67011=CARTESIAN_POINT('Ctrl Pts',(15.5419569163123,10.4651964534784,-3.67207871762998));
#67012=CARTESIAN_POINT('Ctrl Pts',(15.6610210391614,10.946824463739,1.78087986075838));
#67013=CARTESIAN_POINT('Ctrl Pts',(15.7800851620107,8.76155445720668,6.79997517729077));
#67014=CARTESIAN_POINT('Ctrl Pts',(15.8991492848598,4.44176842885027,10.1624402651547));
#67015=CARTESIAN_POINT('Ctrl Pts',(16.018213407709,-0.960134468484163,11.0491013535399));
#67016=CARTESIAN_POINT('Ctrl Pts',(16.1372775305582,-6.12812654370427,9.2439474242726));
#67017=CARTESIAN_POINT('Ctrl Pts',(16.2563416534074,-9.80316615766981,5.18675546015864));
#67018=CARTESIAN_POINT('Ctrl Pts',(16.3754057762566,-11.0899292014957,-0.134049334882309));
#67019=CARTESIAN_POINT('Ctrl Pts',(16.4944698991058,-9.67493062561066,-5.42219663125467));
#67020=CARTESIAN_POINT('Ctrl Pts',(16.613534021955,-5.90289660227532,-9.38937221656565));
#67021=CARTESIAN_POINT('Ctrl Pts',(16.7325981448042,-0.692781307600768,
-11.069080945508));
#67022=CARTESIAN_POINT('Ctrl Pts',(16.8516622676534,4.68611143494755,-10.0521071690279));
#67023=CARTESIAN_POINT('Ctrl Pts',(16.9707263905025,8.92335973679715,-6.58620907093569));
#67024=CARTESIAN_POINT('Ctrl Pts',(17.0897905133518,10.9866725321424,-1.5157590804071));
#67025=CARTESIAN_POINT('Ctrl Pts',(17.208854636201,10.3733794054525,3.92396465693857));
#67026=CARTESIAN_POINT('Ctrl Pts',(17.3279187590501,7.23289265695203,8.40772042419215));
#67027=CARTESIAN_POINT('Ctrl Pts',(17.4469828818993,2.33030703252676,10.8431622717971));
#67028=CARTESIAN_POINT('Ctrl Pts',(17.5660470047485,-3.13999493960738,10.6369605949072));
#67029=CARTESIAN_POINT('Ctrl Pts',(17.6851111275977,-7.84532198180477,7.8393508608927));
#67030=CARTESIAN_POINT('Ctrl Pts',(17.8041752504469,-10.639348289832,3.13189509498916));
#67031=CARTESIAN_POINT('Ctrl Pts',(17.9232393732961,-10.8413848433775,-2.33856229255335));
#67032=CARTESIAN_POINT('Ctrl Pts',(18.0423034961453,-8.4022108948396,-7.23929216132397));
#67033=CARTESIAN_POINT('Ctrl Pts',(18.1613676189945,-3.91606527462211,-10.3763640878329));
#67034=CARTESIAN_POINT('Ctrl Pts',(18.2804317418437,1.52412384461338,-10.98551525531));
#67035=CARTESIAN_POINT('Ctrl Pts',(18.3994958646928,6.59300136823403,-8.91834243998472));
#67036=CARTESIAN_POINT('Ctrl Pts',(18.5185599875421,10.0556722396974,-4.67845644696487));
#67037=CARTESIAN_POINT('Ctrl Pts',(18.6376241103913,11.0685502564019,0.701209055755868));
#67038=CARTESIAN_POINT('Ctrl Pts',(18.7566882332404,9.38487505574641,5.91004391746772));
#67039=CARTESIAN_POINT('Ctrl Pts',(18.8757523560896,5.41482861045058,9.67905625760147));
#67040=CARTESIAN_POINT('Ctrl Pts',(18.9948164789388,0.125605473291401,11.0900280515176));
#67041=CARTESIAN_POINT('Ctrl Pts',(19.113880601788,-5.19421804379792,9.79921414358581));
#67042=CARTESIAN_POINT('Ctrl Pts',(19.2329447246372,-9.24861067308231,6.12108646696947));
#67043=CARTESIAN_POINT('Ctrl Pts',(19.3520088474864,-11.0498291929403,0.951721453584586));
#67044=CARTESIAN_POINT('Ctrl Pts',(19.4710729703356,-10.1590553767408,-4.4495047781391));
#67045=CARTESIAN_POINT('Ctrl Pts',(19.5901370931848,-6.79330219767092,-8.76672938840296));
#67046=CARTESIAN_POINT('Ctrl Pts',(19.709201216034,-1.77254448112488,-10.9481772446742));
#67047=CARTESIAN_POINT('Ctrl Pts',(19.8282653388831,3.68004580723661,-10.4623975156275));
#67048=CARTESIAN_POINT('Ctrl Pts',(19.9473294617324,8.23609236298089,-7.42773730733771));
#67049=CARTESIAN_POINT('Ctrl Pts',(20.0663935845815,10.7856375391046,-2.58350958841375));
#67050=CARTESIAN_POINT('Ctrl Pts',(20.1854577074308,10.7075535376376,2.89012043987658));
#67051=CARTESIAN_POINT('Ctrl Pts',(20.3045218302799,8.02086341584602,7.65965070892345));
#67052=CARTESIAN_POINT('Ctrl Pts',(20.4235859531292,3.38010663229854,10.5631140329289));
#67053=CARTESIAN_POINT('Ctrl Pts',(20.5426500759783,-2.08412180771745,10.8931600194326));
#67054=CARTESIAN_POINT('Ctrl Pts',(20.6617141988275,-7.04061027856087,8.56938188108053));
#67055=CARTESIAN_POINT('Ctrl Pts',(20.7807783216767,-10.2818442798454,4.15790537691507));
#67056=CARTESIAN_POINT('Ctrl Pts',(20.8998424445259,-11.0181847195566,-1.26653243310108));
#67057=CARTESIAN_POINT('Ctrl Pts',(21.0189065673751,-9.07024214417277,-6.38241383525395));
#67058=CARTESIAN_POINT('Ctrl Pts',(21.1379706902243,-4.91258013222972,-9.94339254795818));
#67059=CARTESIAN_POINT('Ctrl Pts',(21.2570348130734,0.441899299721911,-11.0819323191975));
#67060=CARTESIAN_POINT('Ctrl Pts',(21.3760989359227,5.68872190663227,-9.52065869503631));
#67061=CARTESIAN_POINT('Ctrl Pts',(21.4951630587718,9.54964112017613,-5.63993381115507));
#67062=CARTESIAN_POINT('Ctrl Pts',(21.6142271816211,11.0840482891683,-0.385191435202369));
#67063=CARTESIAN_POINT('Ctrl Pts',(21.7332913044702,9.91812656384638,4.96339242674735));
#67064=CARTESIAN_POINT('Ctrl Pts',(21.8523554273194,6.3359212714463,9.10277982598737));
#67065=CARTESIAN_POINT('Ctrl Pts',(21.9714195501686,1.21013994662265,11.0245208616047));
#67066=CARTESIAN_POINT('Ctrl Pts',(22.0904836730178,-4.21045928035888,10.2604352523082));
#67067=CARTESIAN_POINT('Ctrl Pts',(22.209547795867,-8.60529386282905,6.99667181256385));
#67068=CARTESIAN_POINT('Ctrl Pts',(22.3286119187162,-10.9036810954109,2.02835832336125));
#67069=CARTESIAN_POINT('Ctrl Pts',(22.4476760415654,-10.5456810272356,-3.43410986868099));
#67070=CARTESIAN_POINT('Ctrl Pts',(22.5667401644146,-7.61851070238682,-8.05994997478185));
#67071=CARTESIAN_POINT('Ctrl Pts',(22.6858042872638,-2.8352960835593,-10.7222010350917));
#67072=CARTESIAN_POINT('Ctrl Pts',(22.8048684101129,2.63866182135198,-10.7722775080717));
#67073=CARTESIAN_POINT('Ctrl Pts',(22.9239325329622,7.46978106545711,-8.19797961405779));
#67074=CARTESIAN_POINT('Ctrl Pts',(23.0429966558114,10.4810899732101,-3.62646548195945));
#67075=CARTESIAN_POINT('Ctrl Pts',(23.1620607786605,10.938964489467,1.82853898414774));
#67076=CARTESIAN_POINT('Ctrl Pts',(23.2811249015097,8.73185585929995,6.83806933065012));
#67077=CARTESIAN_POINT('Ctrl Pts',(23.4001890243589,4.39746646828528,10.1816888372546));
#67078=CARTESIAN_POINT('Ctrl Pts',(23.5192531472081,-1.00824681597625,11.0448149498506));
#67079=CARTESIAN_POINT('Ctrl Pts',(23.6383172700573,-6.16832800456741,9.21717031124185));
#67080=CARTESIAN_POINT('Ctrl Pts',(23.7573813929065,-9.82566273213694,5.14401115790627));
#67081=CARTESIAN_POINT('Ctrl Pts',(23.8764455157557,-11.0892402070153,-0.18234733198782));
#67082=CARTESIAN_POINT('Ctrl Pts',(23.9955096386049,-9.65122391707266,-5.46428182114477));
#67083=CARTESIAN_POINT('Ctrl Pts',(24.1145737614541,-5.86194767870171,-9.41499167979091));
#67084=CARTESIAN_POINT('Ctrl Pts',(24.2336378843033,-0.644566267852898,
-11.0719931920461));
#67085=CARTESIAN_POINT('Ctrl Pts',(24.3527020071525,4.72984629912008,-10.0316027086936));
#67086=CARTESIAN_POINT('Ctrl Pts',(24.4717661300016,8.95195960737725,-6.54728326149517));
#67087=CARTESIAN_POINT('Ctrl Pts',(24.5908302528509,10.9931698233809,-1.46789514362418));
#67088=CARTESIAN_POINT('Ctrl Pts',(24.7098943757,10.3561912278845,3.9691059660654));
#67089=CARTESIAN_POINT('Ctrl Pts',(24.8289584985493,7.19620644564796,8.43914164533236));
#67090=CARTESIAN_POINT('Ctrl Pts',(24.9480226213984,2.28306039167441,10.8532084733657));
#67091=CARTESIAN_POINT('Ctrl Pts',(25.0670867442476,-3.18629164248494,10.6231842913224));
#67092=CARTESIAN_POINT('Ctrl Pts',(25.1861508670968,-7.87938980590626,7.80510827631169));
#67093=CARTESIAN_POINT('Ctrl Pts',(25.305214989946,-10.6528875302673,3.08552850997112));
#67094=CARTESIAN_POINT('Ctrl Pts',(25.4242791127952,-10.8310970300208,-2.38575691231162));
#67095=CARTESIAN_POINT('Ctrl Pts',(25.5433432356443,-8.37060237545685,-7.27581712183344));
#67096=CARTESIAN_POINT('Ctrl Pts',(25.6624073584936,-3.87083661095472,-10.3933210693051));
#67097=CARTESIAN_POINT('Ctrl Pts',(25.7814714813427,1.57195391066121,-10.9787731473569));
#67098=CARTESIAN_POINT('Ctrl Pts',(25.900535604192,6.6317803333534,-8.88954377504918));
#67099=CARTESIAN_POINT('Ctrl Pts',(26.0195997270411,10.0759526567758,-4.63461724166957));
#67100=CARTESIAN_POINT('Ctrl Pts',(26.1386638498903,11.0653913497591,0.749408563498319));
#67101=CARTESIAN_POINT('Ctrl Pts',(26.2577279727395,9.35904640763797,5.95086121986115));
#67102=CARTESIAN_POINT('Ctrl Pts',(26.3767920955887,5.37262267314378,9.70254732172897));
#67103=CARTESIAN_POINT('Ctrl Pts',(26.4958562184379,0.0773045830813761,
11.0904699142914));
#67104=CARTESIAN_POINT('Ctrl Pts',(26.6149203412871,-5.23684668001598,9.7764991570794));
#67105=CARTESIAN_POINT('Ctrl Pts',(26.7339844641363,-9.27518173984396,6.08074852392641));
#67106=CARTESIAN_POINT('Ctrl Pts',(26.8530485869855,-11.0538693677323,0.903587803967694));
#67107=CARTESIAN_POINT('Ctrl Pts',(26.9721127098347,-10.1395803801334,-4.49370767108662));
#67108=CARTESIAN_POINT('Ctrl Pts',(27.0911768326839,-6.75505658640766,-8.7962326840983));
#67109=CARTESIAN_POINT('Ctrl Pts',(27.210240955533,-1.72484576506137,-10.955793262248));
#67110=CARTESIAN_POINT('Ctrl Pts',(27.3293050783823,3.7255771246663,-10.4462708181691));
#67111=CARTESIAN_POINT('Ctrl Pts',(27.4483692012314,8.26836380646045,-7.39179672896808));
#67112=CARTESIAN_POINT('Ctrl Pts',(27.5674333240806,10.7967870433475,-2.53651108000195));
#67113=CARTESIAN_POINT('Ctrl Pts',(27.6864974469298,10.6948648271749,2.93672696157249));
#67114=CARTESIAN_POINT('Ctrl Pts',(27.805561569779,7.98742775215539,7.6945108241178));
#67115=CARTESIAN_POINT('Ctrl Pts',(27.9246256926282,3.33406971146592,10.5777350164132));
#67116=CARTESIAN_POINT('Ctrl Pts',(28.0436898154774,-2.13154433376724,10.8839798636139));
#67117=CARTESIAN_POINT('Ctrl Pts',(28.1627539383266,-7.07786519262839,8.53863708289256));
#67118=CARTESIAN_POINT('Ctrl Pts',(28.2818180611758,-10.2998554286799,4.11308607576633));
#67119=CARTESIAN_POINT('Ctrl Pts',(28.400882184025,-11.0125641733738,-1.31450722542371));
#67120=CARTESIAN_POINT('Ctrl Pts',(28.5199463068742,-9.04235919719298,-6.42185635679498));
#67121=CARTESIAN_POINT('Ctrl Pts',(28.6390104297233,-4.86922771113678,-9.9646936940112));
#67122=CARTESIAN_POINT('Ctrl Pts',(28.7580745525726,0.490159548834338,-11.0799026410458));
#67123=CARTESIAN_POINT('Ctrl Pts',(28.8771386754217,5.73013267797431,-9.4957926689234));
#67124=CARTESIAN_POINT('Ctrl Pts',(28.9962027982709,9.57411379815596,-5.59828937250734));
#67125=CARTESIAN_POINT('Ctrl Pts',(29.1152669211201,11.0856207670046,-0.336914126337478));
#67126=CARTESIAN_POINT('Ctrl Pts',(29.2343310439693,9.89641574979983,5.00654114389187));
#67127=CARTESIAN_POINT('Ctrl Pts',(29.3533951668185,6.29621641877164,9.13028793228118));
#67128=CARTESIAN_POINT('Ctrl Pts',(29.4724592896677,1.16211406991927,11.0296867501695));
#67129=CARTESIAN_POINT('Ctrl Pts',(29.5915234125169,-4.25510597380623,10.2420003939683));
#67130=CARTESIAN_POINT('Ctrl Pts',(29.710587535366,-8.63568441243642,6.95912736247666));
#67131=CARTESIAN_POINT('Ctrl Pts',(29.8296516582153,-10.9124116648652,1.98085097240602));
#67132=CARTESIAN_POINT('Ctrl Pts',(29.9487157810644,-10.530624649174,-3.48000623800852));
#67133=CARTESIAN_POINT('Ctrl Pts',(30.0677799039137,-7.58333545652726,-8.0930539521336));
#67134=CARTESIAN_POINT('Ctrl Pts',(30.1868440267628,-2.78857146818258,-10.7344477307967));
#67135=CARTESIAN_POINT('Ctrl Pts',(30.3059081496121,2.68555261612554,-10.7606833456054));
#67136=CARTESIAN_POINT('Ctrl Pts',(30.4249722724612,7.5054143643871,-8.16536919785142));
#67137=CARTESIAN_POINT('Ctrl Pts',(30.5440363953104,10.4967846857608,-3.58078345884605));
#67138=CARTESIAN_POINT('Ctrl Pts',(30.6631005181596,10.9308970229689,1.87616342348389));
#67139=CARTESIAN_POINT('Ctrl Pts',(30.7821646410088,8.70199163399651,6.8760337782928));
#67140=CARTESIAN_POINT('Ctrl Pts',(30.901228763858,4.35308109579319,10.2007442812678));
#67141=CARTESIAN_POINT('Ctrl Pts',(31.0202928867072,-1.05634003886347,11.0403190461446));
#67142=CARTESIAN_POINT('Ctrl Pts',(31.1393570095564,-6.20841246348675,9.19021836528331));
#67143=CARTESIAN_POINT('Ctrl Pts',(31.2584211324056,-9.8479729316837,5.10116928313431));
#67144=CARTESIAN_POINT('Ctrl Pts',(31.3774852552547,-11.0883408698522,-0.230641870296499));
#67145=CARTESIAN_POINT('Ctrl Pts',(31.4965493781039,-9.62733414240093,-5.50626336356429));
#67146=CARTESIAN_POINT('Ctrl Pts',(31.6156135009532,-5.82088756466064,-9.44043255777764));
#67147=CARTESIAN_POINT('Ctrl Pts',(31.7346776238023,-0.596339001857024,
-11.0746954230459));
#67148=CARTESIAN_POINT('Ctrl Pts',(31.8537417466515,4.77349144672595,-10.0109079671328));
#67149=CARTESIAN_POINT('Ctrl Pts',(31.9728058695007,8.98038967559343,-6.50823326201993));
#67150=CARTESIAN_POINT('Ctrl Pts',(32.0918699923499,10.9994585942168,-1.42000336354497));
#67151=CARTESIAN_POINT('Ctrl Pts',(32.2109341151991,10.3388066122374,4.0141719884835));
#67152=CARTESIAN_POINT('Ctrl Pts',(32.3299982380483,7.15938373541859,8.47040279133127));
#67153=CARTESIAN_POINT('Ctrl Pts',(32.4490623608975,2.23577044532575,10.8630488093434));
#67154=CARTESIAN_POINT('Ctrl Pts',(32.5681264837467,-3.23252790721539,10.6092064852864));
#67155=CARTESIAN_POINT('Ctrl Pts',(32.6871906065959,-7.91330817233882,7.7707176430471));
#67156=CARTESIAN_POINT('Ctrl Pts',(32.8062547294451,-10.6662247048349,3.03910339809907));
#67157=CARTESIAN_POINT('Ctrl Pts',(32.9253188522942,-10.8206037704871,-2.43290627860795));
#67158=CARTESIAN_POINT('Ctrl Pts',(33.0443829751434,-8.33883508099765,-7.31220407334831));
#67159=CARTESIAN_POINT('Ctrl Pts',(33.1634470979927,-3.82553452456902,-10.4100809084127));
#67160=CARTESIAN_POINT('Ctrl Pts',(33.2825112208418,1.61975415960753,-10.9718227920798));
#67161=CARTESIAN_POINT('Ctrl Pts',(33.401575343691,6.67043350568246,-8.86057649166444));
#67162=CARTESIAN_POINT('Ctrl Pts',(33.5206394665402,10.09604195139,-4.59069012612933));
#67163=CARTESIAN_POINT('Ctrl Pts',(33.6397035893894,11.0620225528029,0.797593856325652));
#67164=CARTESIAN_POINT('Ctrl Pts',(33.7587677122386,9.33304023547071,5.99156564525949));
#67165=CARTESIAN_POINT('Ctrl Pts',(33.8778318350878,5.33031482697323,9.72585434621134));
#67166=CARTESIAN_POINT('Ctrl Pts',(33.996895957937,0.0290022265440831,11.0907014110571));
#67167=CARTESIAN_POINT('Ctrl Pts',(34.1159600807861,-5.27937598279364,9.75359872819613));
#67168=CARTESIAN_POINT('Ctrl Pts',(34.2350242036354,-9.30157687330678,6.04029524016277));
#67169=CARTESIAN_POINT('Ctrl Pts',(34.3540883264846,-11.0576998707618,0.85543701493648));
#67170=CARTESIAN_POINT('Ctrl Pts',(34.4731524493337,-10.1199130541598,-4.53782532658701));
#67171=CARTESIAN_POINT('Ctrl Pts',(34.592216572183,-6.71668284402803,-8.825569131286));
#67172=CARTESIAN_POINT('Ctrl Pts',(34.7112806950321,-1.67711433181609,-10.9632014683844));
#67173=CARTESIAN_POINT('Ctrl Pts',(34.8303448178813,3.77103777468565,-10.4299459739858));
#67174=CARTESIAN_POINT('Ctrl Pts',(34.9494089407305,8.30047841414294,-7.35571594168204));
#67175=CARTESIAN_POINT('Ctrl Pts',(35.0684730635797,10.8077317522112,-2.48946445859646));
#67176=CARTESIAN_POINT('Ctrl Pts',(35.1875371864289,10.6819732546117,2.98327777890839));
#67177=CARTESIAN_POINT('Ctrl Pts',(35.3066013092781,7.9538405815129,7.72922498846084));
#67178=CARTESIAN_POINT('Ctrl Pts',(35.4256654321272,3.28796954940527,10.5921553595362));
#67179=CARTESIAN_POINT('Ctrl Pts',(35.5447295549765,-2.17892642830448,10.8745932585271));
#67180=CARTESIAN_POINT('Ctrl Pts',(35.6637936778256,-7.11498585248852,8.5077303223161));
#67181=CARTESIAN_POINT('Ctrl Pts',(35.7828578006749,-10.3176712080225,4.06818875686869));
#67182=CARTESIAN_POINT('Ctrl Pts',(35.901921923524,-11.0067347389129,-1.36245708393928));
#67183=CARTESIAN_POINT('Ctrl Pts',(36.0209860463733,-9.01430473313378,-6.4611770674213));
#67184=CARTESIAN_POINT('Ctrl Pts',(36.1400501692224,-4.82578292966542,-9.98580582797995));
#67185=CARTESIAN_POINT('Ctrl Pts',(36.2591142920716,0.53841050051321,-11.077662797328));
#67186=CARTESIAN_POINT('Ctrl Pts',(36.3781784149208,5.77143475913937,-9.47074652492433));
#67187=CARTESIAN_POINT('Ctrl Pts',(36.49724253777,9.59840487264048,-5.55653874450998));
#67188=CARTESIAN_POINT('Ctrl Pts',(36.6163066606192,11.0869829708122,-0.28863042682529));
#67189=CARTESIAN_POINT('Ctrl Pts',(36.7353707834684,9.87451721877708,5.04959489607276));
#67190=CARTESIAN_POINT('Ctrl Pts',(36.8544349063176,6.25639213834263,9.15762285364781));
#67191=CARTESIAN_POINT('Ctrl Pts',(36.9734990291668,1.11406615002924,11.034643425672));
#67192=CARTESIAN_POINT('Ctrl Pts',(37.092563152016,-4.29967195564575,10.2233712635413));
#67193=CARTESIAN_POINT('Ctrl Pts',(37.2116272748652,-8.66591115884418,6.92145091042253));
#67194=CARTESIAN_POINT('Ctrl Pts',(37.3306913977143,-10.9209352457521,1.93330604831666));
#67195=CARTESIAN_POINT('Ctrl Pts',(37.4497555205636,-10.5153685243489,-3.52583659795832));
#67196=CARTESIAN_POINT('Ctrl Pts',(37.5688196434127,-7.54801636861026,-8.12600441899707));
#67197=CARTESIAN_POINT('Ctrl Pts',(37.6878837662619,-2.74179395868567,-10.7464908135857));
#67198=CARTESIAN_POINT('Ctrl Pts',(37.8069478891111,2.73239247085885,-10.7488850725814));
#67199=CARTESIAN_POINT('Ctrl Pts',(37.9260120119603,7.540905299281,-8.13260389946816));
#67200=CARTESIAN_POINT('Ctrl Pts',(38.0450761348095,10.5122802934306,-3.53503351479428));
#67201=CARTESIAN_POINT('Ctrl Pts',(38.1641402576587,10.9226222172696,1.92375227541842));
#67202=CARTESIAN_POINT('Ctrl Pts',(38.2832043805079,8.67196234776613,6.91386780010257));
#67203=CARTESIAN_POINT('Ctrl Pts',(38.402268503357,4.30861315328385,10.2196062357469));
#67204=CARTESIAN_POINT('Ctrl Pts',(38.5213326262063,-1.10441322490426,11.0356137277011));
#67205=CARTESIAN_POINT('Ctrl Pts',(38.6403967490554,-6.24837916013266,9.16309209762666));
#67206=CARTESIAN_POINT('Ctrl Pts',(38.7594608719047,-9.87009633312644,5.05823064847518));
#67207=CARTESIAN_POINT('Ctrl Pts',(38.8785249947538,-11.087231207065,-0.278932033749407));
#67208=CARTESIAN_POINT('Ctrl Pts',(38.9975891176031,-9.60326175474091,-5.54814046220001));
#67209=CARTESIAN_POINT('Ctrl Pts',(39.1166532404522,-5.77971703898763,-9.46569436795855));
#67210=CARTESIAN_POINT('Ctrl Pts',(39.2357173633014,-0.548100424397701,
-11.0771875872507));
#67211=CARTESIAN_POINT('Ctrl Pts',(39.3547814861506,4.81704604989658,-9.99002333688758));
#67212=CARTESIAN_POINT('Ctrl Pts',(39.4738456089998,9.00864940217757,-6.46905981321688));
#67213=CARTESIAN_POINT('Ctrl Pts',(39.592909731849,11.0055387253667,-1.37208464858992));
#67214=CARTESIAN_POINT('Ctrl Pts',(39.7119738546982,10.3212258882592,4.05916186937483));
#67215=CARTESIAN_POINT('Ctrl Pts',(39.8310379775473,7.12242522473569,8.50150326921757));
#67216=CARTESIAN_POINT('Ctrl Pts',(39.9501021003966,2.18843809046265,10.8726830930847));
#67217=CARTESIAN_POINT('Ctrl Pts',(40.0691662232457,-3.27870285673611,10.5950274419176));
#67218=CARTESIAN_POINT('Ctrl Pts',(40.188230346095,-7.94707643781875,7.73617961345601));
#67219=CARTESIAN_POINT('Ctrl Pts',(40.3072944689441,-10.6793595603875,2.99262063991577));
#67220=CARTESIAN_POINT('Ctrl Pts',(40.4263585917933,-10.8099052641344,-2.48000949699566));
#67221=CARTESIAN_POINT('Ctrl Pts',(40.5454227146425,-8.30690961341144,-7.34845232588526));
#67222=CARTESIAN_POINT('Ctrl Pts',(40.6644868374917,-3.78015987595825,-10.4266432868441));
#67223=CARTESIAN_POINT('Ctrl Pts',(40.783550960341,1.66752368707546,-10.9646643221022));
#67224=CARTESIAN_POINT('Ctrl Pts',(40.9026150831901,6.70896014758431,-8.83144113776567));
#67225=CARTESIAN_POINT('Ctrl Pts',(41.0216792060393,10.1159397510913,-4.5466759365));
#67226=CARTESIAN_POINT('Ctrl Pts',(41.1407433288885,11.0584439128057,0.845764025927499));
#67227=CARTESIAN_POINT('Ctrl Pts',(41.2598074517377,9.3068570646512,6.03215641060902));
#67228=CARTESIAN_POINT('Ctrl Pts',(41.3788715745869,5.2879058124073,9.7489769101351));
#67229=CARTESIAN_POINT('Ctrl Pts',(41.497935697436,-0.0193005602886234,
11.090722496516));
#67230=CARTESIAN_POINT('Ctrl Pts',(41.6169998202853,-5.32180537687239,9.73051337033048));
#67231=CARTESIAN_POINT('Ctrl Pts',(41.7360639431344,-9.32779512575703,5.99972723038225));
#67232=CARTESIAN_POINT('Ctrl Pts',(41.8551280659836,-11.061321492862,0.807270294617997));
#67233=CARTESIAN_POINT('Ctrl Pts',(41.9741921888328,-10.1000521040008,-4.58185747721788));
#67234=CARTESIAN_POINT('Ctrl Pts',(42.093256311682,-6.67818491998701,-8.85473707366541));
#67235=CARTESIAN_POINT('Ctrl Pts',(42.2123204345312,-1.62934486414103,-10.9704038469609));
#67236=CARTESIAN_POINT('Ctrl Pts',(42.3313845573804,3.81641487563617,-10.4134191893246));
#67237=CARTESIAN_POINT('Ctrl Pts',(42.4504486802296,8.33245879338542,-7.3195035560965));
#67238=CARTESIAN_POINT('Ctrl Pts',(42.5695128030788,10.8184266087902,-2.44235530369298));
#67239=CARTESIAN_POINT('Ctrl Pts',(42.6885769259279,10.6689657463618,3.02974240229508));
#67240=CARTESIAN_POINT('Ctrl Pts',(42.8076410487772,7.91993459599576,7.76385001023172));
#67241=CARTESIAN_POINT('Ctrl Pts',(42.9267051716263,3.24213638239311,10.6062610855322));
#67242=CARTESIAN_POINT('Ctrl Pts',(43.0457692944756,-2.22695126473569,10.8652460449213));
#67243=CARTESIAN_POINT('Ctrl Pts',(43.125145376375,-5.50911884776893,9.2723833665778));
#67244=CARTESIAN_POINT('Ctrl Pts',(43.1648334173247,-6.86098555940043,8.13177966493939));
#67245=CARTESIAN_POINT('Ctrl Pts',(-0.00967375566271921,-10.1537580981707,
2.02645355232637));
#67246=CARTESIAN_POINT('Ctrl Pts',(0.0300142852870114,-10.4906456200829,
0.338443284407024));
#67247=CARTESIAN_POINT('Ctrl Pts',(0.109390367186473,-10.3060172492424,
-3.20712017705732));
#67248=CARTESIAN_POINT('Ctrl Pts',(0.228454490035664,-7.51567182112805,
-7.74635953307546));
#67249=CARTESIAN_POINT('Ctrl Pts',(0.347518612884856,-2.8954366608233,-10.3974248208813));
#67250=CARTESIAN_POINT('Ctrl Pts',(0.466582735734047,2.43073563311717,-10.5159296658786));
#67251=CARTESIAN_POINT('Ctrl Pts',(0.58564685858324,7.16444701004403,-8.07225989849393));
#67252=CARTESIAN_POINT('Ctrl Pts',(0.704710981432431,10.1528779973956,-3.66213262460109));
#67253=CARTESIAN_POINT('Ctrl Pts',(0.823775104281623,10.6677602835861,1.64024187187419));
#67254=CARTESIAN_POINT('Ctrl Pts',(0.942839227130814,8.58376945880916,6.5429807812387));
#67255=CARTESIAN_POINT('Ctrl Pts',(1.06190334998001,4.40855521341405,9.85171730820656));
#67256=CARTESIAN_POINT('Ctrl Pts',(1.1809674728292,-0.840674090499226,10.7603397155692));
#67257=CARTESIAN_POINT('Ctrl Pts',(1.30003159567839,-5.8851012023777,9.04750092933787));
#67258=CARTESIAN_POINT('Ctrl Pts',(1.41909571852758,-9.49577964844291,5.13048047672665));
#67259=CARTESIAN_POINT('Ctrl Pts',(1.53815984137677,-10.7930693726897,-0.0364416268355752));
#67260=CARTESIAN_POINT('Ctrl Pts',(1.65722396422597,-9.46091861334803,-5.19448638601251));
#67261=CARTESIAN_POINT('Ctrl Pts',(1.77628808707516,-5.82387103451064,-9.08703453441888));
#67262=CARTESIAN_POINT('Ctrl Pts',(1.89535220992435,-0.767994430299365,
-10.7657724145786));
#67263=CARTESIAN_POINT('Ctrl Pts',(2.01441633277354,4.47498316424379,-9.82172062457192));
#67264=CARTESIAN_POINT('Ctrl Pts',(2.13348045562273,8.62775207013551,-6.48487201825249));
#67265=CARTESIAN_POINT('Ctrl Pts',(2.25254457847192,10.6786022631659,-1.56815952938864));
#67266=CARTESIAN_POINT('Ctrl Pts',(2.37160870132111,10.1278995459446,3.73059264695215));
#67267=CARTESIAN_POINT('Ctrl Pts',(2.49067282417031,7.10980773486832,8.12048672557844));
#67268=CARTESIAN_POINT('Ctrl Pts',(2.6097369470195,2.35960336741865,10.5320436112022));
#67269=CARTESIAN_POINT('Ctrl Pts',(2.72880106986869,-2.96545461018005,10.3777526299095));
#67270=CARTESIAN_POINT('Ctrl Pts',(2.84786519271788,-7.56805969231213,7.69520260789257));
#67271=CARTESIAN_POINT('Ctrl Pts',(2.96692931556707,-10.3269115065036,3.137924381682));
#67272=CARTESIAN_POINT('Ctrl Pts',(3.08599343841627,-10.5698903467086,-2.18382433921929));
#67273=CARTESIAN_POINT('Ctrl Pts',(3.20505756126546,-8.23780098378548,-6.97354326280402));
#67274=CARTESIAN_POINT('Ctrl Pts',(3.32412168411465,-3.89879398187312,-10.064346783254));
#67275=CARTESIAN_POINT('Ctrl Pts',(3.44318580696384,1.39004883518057,-10.7032441307437));
#67276=CARTESIAN_POINT('Ctrl Pts',(3.56224992981304,6.34024381021831,-8.73458522848382));
#67277=CARTESIAN_POINT('Ctrl Pts',(3.68131405266222,9.74580968303781,-4.63798062830814));
#67278=CARTESIAN_POINT('Ctrl Pts',(3.80037817551142,10.7770723410966,0.588542641932791));
#67279=CARTESIAN_POINT('Ctrl Pts',(3.91944229836061,9.18279250064022,5.67168339884847));
#67280=CARTESIAN_POINT('Ctrl Pts',(4.0385064212098,5.35137337018393,9.37307173446758));
#67281=CARTESIAN_POINT('Ctrl Pts',(4.15757054405899,0.216236702706431,10.7909643857718));
#67282=CARTESIAN_POINT('Ctrl Pts',(4.27663466690818,-4.97158019505263,9.57993011721637));
#67283=CARTESIAN_POINT('Ctrl Pts',(4.39569878975738,-8.9482059015736,6.03500470833572));
#67284=CARTESIAN_POINT('Ctrl Pts',(4.51476291260656,-10.7448430048416,1.01981345740105));
#67285=CARTESIAN_POINT('Ctrl Pts',(4.63382703545577,-9.92378941659614,-4.24382778887703));
#67286=CARTESIAN_POINT('Ctrl Pts',(4.75289115830495,-6.68507266020018,-8.47357505510124));
#67287=CARTESIAN_POINT('Ctrl Pts',(4.87195528115415,-1.81771856896256,-10.6389647001313));
#67288=CARTESIAN_POINT('Ctrl Pts',(4.99101940400334,3.49247354006843,-10.2124580419462));
#67289=CARTESIAN_POINT('Ctrl Pts',(5.11008352685253,7.95181883150745,-7.29796190435888));
#67290=CARTESIAN_POINT('Ctrl Pts',(5.22914764970172,10.4739183087024,-2.60551452677181));
#67291=CARTESIAN_POINT('Ctrl Pts',(5.34821177255092,10.4443305766929,2.72169606887819));
#67292=CARTESIAN_POINT('Ctrl Pts',(5.4672758954001,7.8702638869751,7.38583895275045));
#67293=CARTESIAN_POINT('Ctrl Pts',(5.5863400182493,3.37882004177841,10.2506217280644));
#67294=CARTESIAN_POINT('Ctrl Pts',(5.70540414109848,-1.93578201686793,10.6181174729686));
#67295=CARTESIAN_POINT('Ctrl Pts',(5.82446826394768,-6.77878308850393,8.39879577830077));
#67296=CARTESIAN_POINT('Ctrl Pts',(5.94353238679687,-9.97031681133176,4.13333441282769));
#67297=CARTESIAN_POINT('Ctrl Pts',(6.06259650964606,-10.7328522233696,-1.13910220696014));
#67298=CARTESIAN_POINT('Ctrl Pts',(6.18166063249525,-8.88061817382978,-6.13402735054503));
#67299=CARTESIAN_POINT('Ctrl Pts',(6.30072475534445,-4.8648614448013,-9.63456246071798));
#67300=CARTESIAN_POINT('Ctrl Pts',(6.41978887819363,0.33608733531819,-10.7878967361404));
#67301=CARTESIAN_POINT('Ctrl Pts',(6.53885300104283,5.4551575166716,-9.31305144165389));
#67302=CARTESIAN_POINT('Ctrl Pts',(6.65791712389202,9.24522595777654,-5.56933278555386));
#67303=CARTESIAN_POINT('Ctrl Pts',(6.77698124674122,10.7829448838903,-0.468796669755581));
#67304=CARTESIAN_POINT('Ctrl Pts',(6.89604536959039,9.69369062510556,4.74594908857343));
#67305=CARTESIAN_POINT('Ctrl Pts',(7.01510949243961,6.24283055185546,8.80447257860516));
#67306=CARTESIAN_POINT('Ctrl Pts',(7.13417361528878,1.27107348486386,10.7180242061056));
#67307=CARTESIAN_POINT('Ctrl Pts',(7.25323773813798,-4.01034629456184,10.0204188178082));
#67308=CARTESIAN_POINT('Ctrl Pts',(7.37230186098717,-8.31475355176737,6.88160911851016));
#67309=CARTESIAN_POINT('Ctrl Pts',(7.49136598383636,-10.5934957559904,2.06628128636999));
#67310=CARTESIAN_POINT('Ctrl Pts',(7.61043010668555,-10.2914189367481,-3.25244015393571));
#67311=CARTESIAN_POINT('Ctrl Pts',(7.72949422953475,-7.48211594946837,-7.77879242590399));
#67312=CARTESIAN_POINT('Ctrl Pts',(7.84855835238394,-2.84999756461396,-10.4100520924866));
#67313=CARTESIAN_POINT('Ctrl Pts',(7.96762247523312,2.47644572497516,-10.5051838278938));
#67314=CARTESIAN_POINT('Ctrl Pts',(8.08668659808232,7.19956992284888,-8.04101135508465));
#67315=CARTESIAN_POINT('Ctrl Pts',(8.20575072093152,10.1687134286408,-3.61786371948564));
#67316=CARTESIAN_POINT('Ctrl Pts',(8.3248148437807,10.6605246481603,1.68667866309985));
#67317=CARTESIAN_POINT('Ctrl Pts',(8.4438789666299,8.55518706563913,6.58030736048942));
#67318=CARTESIAN_POINT('Ctrl Pts',(8.56294308947908,4.36560930056807,9.87082195773906));
#67319=CARTESIAN_POINT('Ctrl Pts',(8.68200721232828,-0.887531219559736,
10.7565774771019));
#67320=CARTESIAN_POINT('Ctrl Pts',(8.80107133517747,-5.92444873756254,9.02178351782972));
#67321=CARTESIAN_POINT('Ctrl Pts',(8.92013545802667,-9.51803438876389,5.08907575704059));
#67322=CARTESIAN_POINT('Ctrl Pts',(9.03919958087585,-10.7928081215643,-0.0834478141433222));
#67323=CARTESIAN_POINT('Ctrl Pts',(9.15826370372506,-9.43820575809417,-5.23564158002325));
#67324=CARTESIAN_POINT('Ctrl Pts',(9.27732782657423,-5.78423956525768,-9.11231273268744));
#67325=CARTESIAN_POINT('Ctrl Pts',(9.39639194942343,-0.721099682248477,
-10.7690150865737));
#67326=CARTESIAN_POINT('Ctrl Pts',(9.51545607227262,4.5177166555051,-9.80213787431916));
#67327=CARTESIAN_POINT('Ctrl Pts',(9.63452019512182,8.65591339084267,-6.44723460538088));
#67328=CARTESIAN_POINT('Ctrl Pts',(9.753584317971,10.6853306959413,-1.52163681769487));
#67329=CARTESIAN_POINT('Ctrl Pts',(9.8726484408202,10.1115558756728,3.77466666869229));
#67330=CARTESIAN_POINT('Ctrl Pts',(9.99171256366938,7.07437366261684,8.15137460605652));
#67331=CARTESIAN_POINT('Ctrl Pts',(10.1107766865186,2.31371144370355,10.5422203563512));
#67332=CARTESIAN_POINT('Ctrl Pts',(10.2298408093678,-3.01062405608528,10.3647389489321));
#67333=CARTESIAN_POINT('Ctrl Pts',(10.348904932217,-7.60150234633553,7.66216893348388));
#67334=CARTESIAN_POINT('Ctrl Pts',(10.4679690550662,-10.3404799690232,3.09291847561804));
#67335=CARTESIAN_POINT('Ctrl Pts',(10.5870331779154,-10.5602790287019,-2.22983800365615));
#67336=CARTESIAN_POINT('Ctrl Pts',(10.7060973007645,-8.20735142306188,-7.00935469961067));
#67337=CARTESIAN_POINT('Ctrl Pts',(10.8251614236137,-3.85492439128332,-10.0812315033472));
#67338=CARTESIAN_POINT('Ctrl Pts',(10.9442255464629,1.43665081520601,-10.6970886283025));
#67339=CARTESIAN_POINT('Ctrl Pts',(11.0632896693121,6.37822486632941,-8.70688912534939));
#67340=CARTESIAN_POINT('Ctrl Pts',(11.1823537921613,9.76591675710413,-4.59549133171882));
#67341=CARTESIAN_POINT('Ctrl Pts',(11.3014179150105,10.7744068877742,0.635473762853294));
#67342=CARTESIAN_POINT('Ctrl Pts',(11.4204820378597,9.15800388561784,5.71162284448113));
#67343=CARTESIAN_POINT('Ctrl Pts',(11.5395461607089,5.31050066976602,9.39628933797829));
#67344=CARTESIAN_POINT('Ctrl Pts',(11.6586102835581,0.169237446042603,10.791803805363));
#67345=CARTESIAN_POINT('Ctrl Pts',(11.7776744064073,-5.01325590891323,9.55818685098469));
#67346=CARTESIAN_POINT('Ctrl Pts',(11.8967385292565,-8.97440491095257,5.99597591563379));
#67347=CARTESIAN_POINT('Ctrl Pts',(12.0158026521057,-10.7491826289547,0.973007449081952));
#67348=CARTESIAN_POINT('Ctrl Pts',(12.1348667749548,-9.90521242327705,-4.28700799350178));
#67349=CARTESIAN_POINT('Ctrl Pts',(12.253930897804,-6.64810483195373,-8.50260976582741));
#67350=CARTESIAN_POINT('Ctrl Pts',(12.3729950206532,-1.77136611833576,-10.6467803941568));
#67351=CARTESIAN_POINT('Ctrl Pts',(12.4920591435024,3.53691809084141,-10.1971506365881));
#67352=CARTESIAN_POINT('Ctrl Pts',(12.6111232663516,7.98352776844378,-7.26326063535359));
#67353=CARTESIAN_POINT('Ctrl Pts',(12.7301873892008,10.4851666060368,-2.55987342074571));
#67354=CARTESIAN_POINT('Ctrl Pts',(12.84925151205,10.432377890689,2.76715778958364));
#67355=CARTESIAN_POINT('Ctrl Pts',(12.9683156348992,7.83802216663728,7.42004576818046));
#67356=CARTESIAN_POINT('Ctrl Pts',(13.0873797577484,3.33414411115286,10.2652400718471));
#67357=CARTESIAN_POINT('Ctrl Pts',(13.2064438805976,-1.98200807434881,10.6095859806029));
#67358=CARTESIAN_POINT('Ctrl Pts',(13.3255080034467,-6.81529754288107,8.3691929173959));
#67359=CARTESIAN_POINT('Ctrl Pts',(13.444572126296,-9.98822390235193,4.08987212062618));
#67360=CARTESIAN_POINT('Ctrl Pts',(13.5636362491451,-10.7277893721236,-1.1858355172374));
#67361=CARTESIAN_POINT('Ctrl Pts',(13.6827003719943,-8.85381880723454,-6.17264637050028));
#67362=CARTESIAN_POINT('Ctrl Pts',(13.8017644948435,-4.8228545044563,-9.65565870955656));
#67363=CARTESIAN_POINT('Ctrl Pts',(13.9208286176927,0.383067993351009,-10.7863306828161));
#67364=CARTESIAN_POINT('Ctrl Pts',(14.0398927405419,5.4956663243967,-9.28920461274712));
#67365=CARTESIAN_POINT('Ctrl Pts',(14.1589568633911,9.26939403866785,-5.52901481662866));
#67366=CARTESIAN_POINT('Ctrl Pts',(14.2780209862403,10.7848843380173,-0.421829944620547));
#67367=CARTESIAN_POINT('Ctrl Pts',(14.3970851090895,9.67292895687089,4.78812239629677));
#67368=CARTESIAN_POINT('Ctrl Pts',(14.5161492319387,6.20442578078106,8.83157808193808));
#67369=CARTESIAN_POINT('Ctrl Pts',(14.6352133547879,1.2243818957931,10.7234583815038));
#67370=CARTESIAN_POINT('Ctrl Pts',(14.7542774776371,-4.05394955747593,10.0028577752576));
#67371=CARTESIAN_POINT('Ctrl Pts',(14.8733416004862,-8.34464573159859,6.84533113155994));
#67372=CARTESIAN_POINT('Ctrl Pts',(14.9924057233354,-10.6023944307566,2.02012450637368));
#67373=CARTESIAN_POINT('Ctrl Pts',(15.1114698461846,-10.2771561847689,-3.29723087460632));
#67374=CARTESIAN_POINT('Ctrl Pts',(15.2305339690338,-7.44816650490929,-7.81130503832346));
#67375=CARTESIAN_POINT('Ctrl Pts',(15.349598091883,-2.80463229238797,-10.4223657770721));
#67376=CARTESIAN_POINT('Ctrl Pts',(15.4686622147322,2.52217480197953,-10.4942986880901));
#67377=CARTESIAN_POINT('Ctrl Pts',(15.5877263375814,7.23452215053809,-8.00957926110754));
#67378=CARTESIAN_POINT('Ctrl Pts',(15.7067904604306,10.1843736410856,-3.57354225179328));
#67379=CARTESIAN_POINT('Ctrl Pts',(15.8258545832798,10.6530776577097,1.73309177639174));
#67380=CARTESIAN_POINT('Ctrl Pts',(15.944918706129,8.52644713031192,6.61750481832738));
#67381=CARTESIAN_POINT('Ctrl Pts',(16.0639828289782,4.32257812910462,9.88974160453022));
#67382=CARTESIAN_POINT('Ctrl Pts',(16.1830469518274,-0.934370244858374,
10.752610052081));
#67383=CARTESIAN_POINT('Ctrl Pts',(16.3021110746765,-5.96368455368977,8.99589557691018));
#67384=CARTESIAN_POINT('Ctrl Pts',(16.4211751975257,-9.54010824920252,5.04757419758126));
#67385=CARTESIAN_POINT('Ctrl Pts',(16.5402393203749,-10.7923423266151,-0.130452258478766));
#67386=CARTESIAN_POINT('Ctrl Pts',(16.6593034432241,-9.41531378611153,-5.27669754634927));
#67387=CARTESIAN_POINT('Ctrl Pts',(16.7783675660733,-5.74449842671464,-9.13741804406819));
#67388=CARTESIAN_POINT('Ctrl Pts',(16.8974316889225,-0.674191231815933,
-10.7720535121922));
#67389=CARTESIAN_POINT('Ctrl Pts',(17.0164958117717,4.56036444126248,-9.78236918386642));
#67390=CARTESIAN_POINT('Ctrl Pts',(17.1355599346209,8.68391053119262,-6.40947490617067));
#67391=CARTESIAN_POINT('Ctrl Pts',(17.2546240574701,10.6918564440708,-1.47508524023966));
#67392=CARTESIAN_POINT('Ctrl Pts',(17.3736881803193,10.0950204093642,3.81866909028671));
#67393=CARTESIAN_POINT('Ctrl Pts',(17.4927523031685,7.03880540147718,8.18210787063613));
#67394=CARTESIAN_POINT('Ctrl Pts',(17.6118164260177,2.26777563356814,10.5521971343595));
#67395=CARTESIAN_POINT('Ctrl Pts',(17.7308805488668,-3.05573639618109,10.3515286679623));
#67396=CARTESIAN_POINT('Ctrl Pts',(17.849944671716,-7.63480081358285,7.62898992157575));
#67397=CARTESIAN_POINT('Ctrl Pts',(17.9690087945652,-10.3538522915429,3.04785390258501));
#67398=CARTESIAN_POINT('Ctrl Pts',(18.0880729174144,-10.5504674014084,-2.27580937215951));
#67399=CARTESIAN_POINT('Ctrl Pts',(18.2071370402636,-8.17674618385253,-7.04503318171342));
#67400=CARTESIAN_POINT('Ctrl Pts',(18.3262011631128,-3.81098167979215,-10.0979250008543));
#67401=CARTESIAN_POINT('Ctrl Pts',(18.445265285962,1.48322554457836,-10.6907302215752));
#67402=CARTESIAN_POINT('Ctrl Pts',(18.5643294088112,6.41608493913803,-8.67902786839379));
#67403=CARTESIAN_POINT('Ctrl Pts',(18.6833935316604,9.78583858952125,-4.55291486703044));
#67404=CARTESIAN_POINT('Ctrl Pts',(18.8024576545096,10.771537063584,0.682392829993814));
#67405=CARTESIAN_POINT('Ctrl Pts',(18.9215217773588,9.1330415599467,5.751453951035));
#67406=CARTESIAN_POINT('Ctrl Pts',(19.040585900208,5.26952723882593,9.41932871099962));
#67407=CARTESIAN_POINT('Ctrl Pts',(19.1596500230572,0.122234979252591,10.7924385240981));
#67408=CARTESIAN_POINT('Ctrl Pts',(19.2787141459063,-5.0548365304431,9.53626228336279));
#67409=CARTESIAN_POINT('Ctrl Pts',(19.3977782687555,-9.00043369222129,5.95683339019299));
#67410=CARTESIAN_POINT('Ctrl Pts',(19.5168423916048,-10.7533183606577,0.926182984584216));
#67411=CARTESIAN_POINT('Ctrl Pts',(19.6359065144539,-9.88644754612495,-4.33010688139561));
#67412=CARTESIAN_POINT('Ctrl Pts',(19.7549706373031,-6.61101090127101,-8.53148319753759));
#67413=CARTESIAN_POINT('Ctrl Pts',(19.8740347601523,-1.72498006812094,-10.6543941381561));
#67414=CARTESIAN_POINT('Ctrl Pts',(19.9930988830015,3.58129555272233,-10.1816498098609));
#67415=CARTESIAN_POINT('Ctrl Pts',(20.1121630058507,8.0150852724039,-7.22842159552721));
#67416=CARTESIAN_POINT('Ctrl Pts',(20.2312271286999,10.4962160188641,-2.51418375858465));
#67417=CARTESIAN_POINT('Ctrl Pts',(20.350291251549,10.4202273214836,2.8125670223475));
#67418=CARTESIAN_POINT('Ctrl Pts',(20.4693553743983,7.80563177329927,7.45411183886123));
#67419=CARTESIAN_POINT('Ctrl Pts',(20.5884194972474,3.28940493788801,10.2796637027282));
#67420=CARTESIAN_POINT('Ctrl Pts',(20.7074836200966,-2.02819653674767,10.6008532437212));
#67421=CARTESIAN_POINT('Ctrl Pts',(20.8265477429458,-6.85168272348085,8.33943130814951));
#67422=CARTESIAN_POINT('Ctrl Pts',(20.945611865795,-10.0059415349627,4.04633225100204));
#67423=CARTESIAN_POINT('Ctrl Pts',(21.0646759886442,-10.7225230342586,-1.2325463343755));
#67424=CARTESIAN_POINT('Ctrl Pts',(21.1837401114934,-8.82685149982761,-6.2111483066001));
#67425=CARTESIAN_POINT('Ctrl Pts',(21.3028042343426,-4.78075608334823,-9.67657180814152));
#67426=CARTESIAN_POINT('Ctrl Pts',(21.4218683571918,0.430041385281963,-10.7845600324508));
#67427=CARTESIAN_POINT('Ctrl Pts',(21.540932480041,5.53607088934433,-9.26518158455325));
#67428=CARTESIAN_POINT('Ctrl Pts',(21.6599966028902,9.29338629604245,-5.48859197236602));
#67429=CARTESIAN_POINT('Ctrl Pts',(21.7790607257394,10.7866192225379,-0.374855218140065));
#67430=CARTESIAN_POINT('Ctrl Pts',(21.8981248485886,9.65198381079736,4.83020488206198));
#67431=CARTESIAN_POINT('Ctrl Pts',(22.0171889714377,6.16590332305359,8.85851606632548));
#67432=CARTESIAN_POINT('Ctrl Pts',(22.136253094287,1.17766708242847,10.728689152434));
#67433=CARTESIAN_POINT('Ctrl Pts',(22.2553172171361,-4.09747592435287,9.9851069967196));
#67434=CARTESIAN_POINT('Ctrl Pts',(22.3743813399853,-8.37437962870365,6.80892330115003));
#67435=CARTESIAN_POINT('Ctrl Pts',(22.4934454628345,-10.6110919974173,1.9739294082961));
#67436=CARTESIAN_POINT('Ctrl Pts',(22.6125095856837,-10.2626984938611,-3.34195905281468));
#67437=CARTESIAN_POINT('Ctrl Pts',(22.7315737085329,-7.41407578220163,-7.84366948451815));
#67438=CARTESIAN_POINT('Ctrl Pts',(22.8506378313821,-2.75921382139721,-10.4344817683678));
#67439=CARTESIAN_POINT('Ctrl Pts',(22.9697019542313,2.56785603792307,-10.4832144905602));
#67440=CARTESIAN_POINT('Ctrl Pts',(23.0887660770805,7.26933715252287,-7.97799524000491));
#67441=CARTESIAN_POINT('Ctrl Pts',(23.2078301999297,10.1998406745176,-3.52915300051523));
#67442=CARTESIAN_POINT('Ctrl Pts',(23.3268943227789,10.6454285977851,1.77947201609021));
#67443=CARTESIAN_POINT('Ctrl Pts',(23.4459584456281,8.49754546381735,6.65457675415553));
#67444=CARTESIAN_POINT('Ctrl Pts',(23.5650225684772,4.27946496620967,9.90847366094163));
#67445=CARTESIAN_POINT('Ctrl Pts',(23.6840866913264,-0.981191546855646,
10.748438669638));
#67446=CARTESIAN_POINT('Ctrl Pts',(23.8031508141756,-6.0028072495864,8.96983700024163));
#67447=CARTESIAN_POINT('Ctrl Pts',(23.9222149370249,-9.56200115116915,5.00597689483582));
#67448=CARTESIAN_POINT('Ctrl Pts',(24.041279059874,-10.7916718205949,-0.177454228372508));
#67449=CARTESIAN_POINT('Ctrl Pts',(24.1603431827232,-9.39224322278051,-5.3176534233366));
#67450=CARTESIAN_POINT('Ctrl Pts',(24.2794073055724,-5.70464832550272,-9.16235003527637));
#67451=CARTESIAN_POINT('Ctrl Pts',(24.3984714284216,-0.627269993204219,
-10.7748876115817));
#67452=CARTESIAN_POINT('Ctrl Pts',(24.5175355512708,4.60292572521498,-9.76241493969318));
#67453=CARTESIAN_POINT('Ctrl Pts',(24.63659967412,8.71174295358137,-6.37159363089923));
#67454=CARTESIAN_POINT('Ctrl Pts',(24.7556637969692,10.6981793871633,-1.42850568310496));
#67455=CARTESIAN_POINT('Ctrl Pts',(24.8747279198183,10.0782934589109,3.8625990786858));
#67456=CARTESIAN_POINT('Ctrl Pts',(24.9937920426676,7.00310362702341,8.21268593553664));
#67457=CARTESIAN_POINT('Ctrl Pts',(25.1128561655167,2.2217968078609,10.5619737564136));
#67458=CARTESIAN_POINT('Ctrl Pts',(25.2319202883659,-3.10079077452471,10.3381220373534));
#67459=CARTESIAN_POINT('Ctrl Pts',(25.3509844112151,-7.66795446256887,7.59566620162843));
#67460=CARTESIAN_POINT('Ctrl Pts',(25.4700485340643,-10.3670282203486,3.00273151731647));
#67461=CARTESIAN_POINT('Ctrl Pts',(25.5891126569135,-10.5404556509706,-2.32173757270537));
#67462=CARTESIAN_POINT('Ctrl Pts',(25.7081767797627,-8.14598584666568,-7.08057803237226));
#67463=CARTESIAN_POINT('Ctrl Pts',(25.8272409026119,-3.76696668092202,-10.114426959122));
#67464=CARTESIAN_POINT('Ctrl Pts',(25.9463050254611,1.52977213986441,-10.6841690311734));
#67465=CARTESIAN_POINT('Ctrl Pts',(26.0653691483103,6.45382331050506,-8.65100198609224));
#67466=CARTESIAN_POINT('Ctrl Pts',(26.1844332711594,9.80557480240951,-4.51025204184217));
#67467=CARTESIAN_POINT('Ctrl Pts',(26.3034973940087,10.7684629229608,0.729298953385538));
#67468=CARTESIAN_POINT('Ctrl Pts',(26.4225615168578,9.10790599711709,5.79117596298612));
#67469=CARTESIAN_POINT('Ctrl Pts',(26.541625639707,5.22845385455499,9.44218941651667));
#67470=CARTESIAN_POINT('Ctrl Pts',(26.6606897625562,0.0752301938878147,
10.7928685299376));
#67471=CARTESIAN_POINT('Ctrl Pts',(26.7797538854054,-5.09632127093359,9.51415683021992));
#67472=CARTESIAN_POINT('Ctrl Pts',(26.8988180082546,-9.02629175166107,5.91757787447576));
#67473=CARTESIAN_POINT('Ctrl Pts',(27.0178821311038,-10.7572501215032,0.879340952082804));
#67474=CARTESIAN_POINT('Ctrl Pts',(27.136946253953,-9.86749514107549,-4.37312363505099));
#67475=CARTESIAN_POINT('Ctrl Pts',(27.2560103768022,-6.57379157175643,-8.56019480255527));
#67476=CARTESIAN_POINT('Ctrl Pts',(27.3750744996514,-1.67856129817712,-10.6618057877103));
#67477=CARTESIAN_POINT('Ctrl Pts',(27.4941386225006,3.6256050839515,-10.1659558557873));
#67478=CARTESIAN_POINT('Ctrl Pts',(27.6132027453498,8.04649074479939,-7.1934454457129));
#67479=CARTESIAN_POINT('Ctrl Pts',(27.7322668681989,10.507066337597,-2.46844640693843));
#67480=CARTESIAN_POINT('Ctrl Pts',(27.8513309910482,10.407879099551,2.85792290583927));
#67481=CARTESIAN_POINT('Ctrl Pts',(27.9703951138973,7.7730933213479,7.48803651862131));
#67482=CARTESIAN_POINT('Ctrl Pts',(28.0894592367465,3.24460337060461,10.2938923471179));
#67483=CARTESIAN_POINT('Ctrl Pts',(28.2085233595957,-2.07434652795348,10.5919194279676));
#67484=CARTESIAN_POINT('Ctrl Pts',(28.3275874824449,-6.88793794014274,8.30951151508511));
#67485=CARTESIAN_POINT('Ctrl Pts',(28.4466516052941,-10.0234693730927,4.00271562982726));
#67486=CARTESIAN_POINT('Ctrl Pts',(28.5657157281433,-10.7170533096675,-1.2792337723552));
#67487=CARTESIAN_POINT('Ctrl Pts',(28.6847798509925,-8.79971676312973,-6.24953242853283));
#67488=CARTESIAN_POINT('Ctrl Pts',(28.8038439738417,-4.73856698000755,-9.69730135978937));
#67489=CARTESIAN_POINT('Ctrl Pts',(28.9229080966909,0.477006620111307,-10.7825848186304));
#67490=CARTESIAN_POINT('Ctrl Pts',(29.0419722195401,5.57637044511356,-9.2409828127453));
#67491=CARTESIAN_POINT('Ctrl Pts',(29.1610363423893,9.31720227481098,-5.44806501951358));
#67492=CARTESIAN_POINT('Ctrl Pts',(29.2801004652384,10.7881495045443,-0.327873381339212));
#67493=CARTESIAN_POINT('Ctrl Pts',(29.3991645880876,9.63085558417639,4.87219574764075));
#67494=CARTESIAN_POINT('Ctrl Pts',(29.5182287109368,6.1272639093741,8.8852860208027));
#67495=CARTESIAN_POINT('Ctrl Pts',(29.637292833786,1.13092993086498,10.7337164196779));
#67496=CARTESIAN_POINT('Ctrl Pts',(29.7563569566353,-4.14092456957688,9.96716681889415));
#67497=CARTESIAN_POINT('Ctrl Pts',(29.8754210794844,-8.40395467908472,6.77238631787057));
#67498=CARTESIAN_POINT('Ctrl Pts',(29.9944852023336,-10.6195882909956,1.92769686837416));
#67499=CARTESIAN_POINT('Ctrl Pts',(30.1135493251828,-10.2480461382611,-3.38662384014844));
#67500=CARTESIAN_POINT('Ctrl Pts',(30.232613448032,-7.3798444279845,-7.87588515059335));
#67501=CARTESIAN_POINT('Ctrl Pts',(30.3516775708811,-2.71374301314742,-10.4463998365553));
#67502=CARTESIAN_POINT('Ctrl Pts',(30.4707416937304,2.61348856631605,-10.4719314455513));
#67503=CARTESIAN_POINT('Ctrl Pts',(30.5898058165796,7.30401426842611,-7.94625989086803));
#67504=CARTESIAN_POINT('Ctrl Pts',(30.7088699394287,10.2151142355556,-3.4846968076348));
#67505=CARTESIAN_POINT('Ctrl Pts',(30.827934062278,10.6375776134755,1.82581850244647));
#67506=CARTESIAN_POINT('Ctrl Pts',(30.9469981851271,8.4684826143674,6.69152246478688));
#67507=CARTESIAN_POINT('Ctrl Pts',(31.0660623079763,4.2362706296611,9.9270177716604));
#67508=CARTESIAN_POINT('Ctrl Pts',(31.1851264308255,-1.02799423743721,10.7440634088964));
#67509=CARTESIAN_POINT('Ctrl Pts',(31.3041905536747,-6.04181608316635,8.94360828210754));
#67510=CARTESIAN_POINT('Ctrl Pts',(31.4232546765239,-9.58371267939525,4.9642846378293));
#67511=CARTESIAN_POINT('Ctrl Pts',(31.5423187993731,-10.7907966162221,-0.224452832282696));
#67512=CARTESIAN_POINT('Ctrl Pts',(31.6613829222223,-9.36899450570772,-5.3585084341269));
#67513=CARTESIAN_POINT('Ctrl Pts',(31.7804470450715,-5.66469001750546,-9.18710823339773));
#67514=CARTESIAN_POINT('Ctrl Pts',(31.8995111679207,-0.58033685642333,-10.7775173309843));
#67515=CARTESIAN_POINT('Ctrl Pts',(32.0185752907699,4.64539970005286,-9.74227552029498));
#67516=CARTESIAN_POINT('Ctrl Pts',(32.137639413619,8.73941013007846,-6.33359149810527));
#67517=CARTESIAN_POINT('Ctrl Pts',(32.2567035364682,10.7042994052844,-1.38189902982028));
#67518=CARTESIAN_POINT('Ctrl Pts',(32.3757676593175,10.0613753415927,3.90645580061775));
#67519=CARTESIAN_POINT('Ctrl Pts',(32.4948317821666,6.96726901645299,8.24310822074808));
#67520=CARTESIAN_POINT('Ctrl Pts',(32.6138959050159,2.17577583871593,10.5715500370689));
#67521=CARTESIAN_POINT('Ctrl Pts',(32.732960027865,-3.14578633651692,10.3245193114049));
#67522=CARTESIAN_POINT('Ctrl Pts',(32.8520241507142,-7.7009626644292,7.56219840573208));
#67523=CARTESIAN_POINT('Ctrl Pts',(32.9710882735634,-10.380007505517,2.957552175702));
#67524=CARTESIAN_POINT('Ctrl Pts',(33.0901523964126,-10.5302439672932,-2.36762173411953));
#67525=CARTESIAN_POINT('Ctrl Pts',(33.2092165192618,-8.11507099496873,-7.1159885773663));
#67526=CARTESIAN_POINT('Ctrl Pts',(33.328280642111,-3.72288022955689,-10.1307370651382));
#67527=CARTESIAN_POINT('Ctrl Pts',(33.4473447649602,1.57628971816028,-10.677405181551));
#67528=CARTESIAN_POINT('Ctrl Pts',(33.5664088878093,6.49143926460226,-8.6228120100446));
#67529=CARTESIAN_POINT('Ctrl Pts',(33.6854730106585,9.82512502140889,-4.46750366539021));
#67530=CARTESIAN_POINT('Ctrl Pts',(33.8045371335077,10.7651845242154,0.776191243304808));
#67531=CARTESIAN_POINT('Ctrl Pts',(33.9236012563569,9.08259767390472,5.83078812688053));
#67532=CARTESIAN_POINT('Ctrl Pts',(34.0426653792061,5.18728129604011,9.46487102090372));
#67533=CARTESIAN_POINT('Ctrl Pts',(34.1617295020553,0.0282239815431699,
10.793093814725));
#67534=CARTESIAN_POINT('Ctrl Pts',(34.2807936249045,-5.13770934349468,9.49187091085613));
#67535=CARTESIAN_POINT('Ctrl Pts',(34.3998577477537,-9.0519785987916,5.87821011308789));
#67536=CARTESIAN_POINT('Ctrl Pts',(34.5189218706029,-10.760977836913,0.832482240085673));
#67537=CARTESIAN_POINT('Ctrl Pts',(34.637985993452,-9.84835556762113,-4.41605743851872));
#67538=CARTESIAN_POINT('Ctrl Pts',(34.7570501163013,-6.53644754939258,-8.58874403627388));
#67539=CARTESIAN_POINT('Ctrl Pts',(34.8761142391504,-1.63211068898355,-10.6690152022338));
#67540=CARTESIAN_POINT('Ctrl Pts',(34.9951783619997,3.66984584405779,-10.1500690720527));
#67541=CARTESIAN_POINT('Ctrl Pts',(35.1142424848488,8.07774358992556,-7.15833284934464));
#67542=CARTESIAN_POINT('Ctrl Pts',(35.2333066076981,10.5177173564246,-2.42266223336136));
#67543=CARTESIAN_POINT('Ctrl Pts',(35.3523707305472,10.3953334591143,2.9032245797404));
#67544=CARTESIAN_POINT('Ctrl Pts',(35.4714348533964,7.74040742797833,7.52181916397147));
#67545=CARTESIAN_POINT('Ctrl Pts',(35.5904989762456,3.19974025910667,10.3079257351245));
#67546=CARTESIAN_POINT('Ctrl Pts',(35.7095630990948,-2.12045717258492,10.5827847028002));
#67547=CARTESIAN_POINT('Ctrl Pts',(35.828627221944,-6.92406250517119,8.27943410572681));
#67548=CARTESIAN_POINT('Ctrl Pts',(35.9476913447932,-10.0408070842708,3.95902308442984));
#67549=CARTESIAN_POINT('Ctrl Pts',(36.0667554676423,-10.711380302101,-1.32589694560097));
#67550=CARTESIAN_POINT('Ctrl Pts',(36.1858195904916,-8.77241511183733,-6.28779800822183));
#67551=CARTESIAN_POINT('Ctrl Pts',(36.3048837133408,-4.69628799468449,-9.71784697129834));
#67552=CARTESIAN_POINT('Ctrl Pts',(36.4239478361899,0.523962806994189,-10.7804050788213));
#67553=CARTESIAN_POINT('Ctrl Pts',(36.5430119590391,5.61656422729522,-9.21660875632994));
#67554=CARTESIAN_POINT('Ctrl Pts',(36.6620760818884,9.34084152322772,-5.40743472679377));
#67555=CARTESIAN_POINT('Ctrl Pts',(36.7811402047375,10.78947515501,-0.280885325377527));
#67556=CARTESIAN_POINT('Ctrl Pts',(36.9002043275867,9.6095446777717,4.91409419654326));
#67557=CARTESIAN_POINT('Ctrl Pts',(37.0192684504359,6.08850827266157,8.91188743759264));
#67558=CARTESIAN_POINT('Ctrl Pts',(37.1383325732851,1.08417132762113,10.7385400878776));
#67559=CARTESIAN_POINT('Ctrl Pts',(37.2573966961343,-4.18429466900627,9.94903758207373));
#67560=CARTESIAN_POINT('Ctrl Pts',(37.3764608189835,-8.43337032175702,6.73572087476154));
#67561=CARTESIAN_POINT('Ctrl Pts',(37.4955249418327,-10.6278831503323,1.88142776355463));
#67562=CARTESIAN_POINT('Ctrl Pts',(37.6145890646819,-10.233199395897,-3.43122438939844));
#67563=CARTESIAN_POINT('Ctrl Pts',(37.733653187531,-7.34547309156401,-7.9079514254767));
#67564=CARTESIAN_POINT('Ctrl Pts',(37.8527173103803,-2.6682207301369,-10.4581197555706));
#67565=CARTESIAN_POINT('Ctrl Pts',(37.9717814332294,2.65907152159249,-10.460449767082));
#67566=CARTESIAN_POINT('Ctrl Pts',(38.0908455560787,7.33855284048615,-7.91437381565864));
#67567=CARTESIAN_POINT('Ctrl Pts',(38.2099096789278,10.2301940344878,-3.44017451640469));
#67568=CARTESIAN_POINT('Ctrl Pts',(38.328973801777,10.6295248536994,1.87213035635251));
#67569=CARTESIAN_POINT('Ctrl Pts',(38.4480379246262,8.43925913323114,6.72834124942876));
#67570=CARTESIAN_POINT('Ctrl Pts',(38.5671020474754,4.19299593877704,9.94537358493831));
#67571=CARTESIAN_POINT('Ctrl Pts',(38.6861661703246,-1.07477742884057,10.739484352847));
#67572=CARTESIAN_POINT('Ctrl Pts',(38.8052302931738,-6.08071031450269,8.91720992001931));
#67573=CARTESIAN_POINT('Ctrl Pts',(38.924294416023,-9.60524242205285,4.92249821738793));
#67574=CARTESIAN_POINT('Ctrl Pts',(39.0433585388722,-10.7897167300976,-0.271447178731887));
#67575=CARTESIAN_POINT('Ctrl Pts',(39.1624226617214,-9.34556807587885,-5.39926180377519));
#67576=CARTESIAN_POINT('Ctrl Pts',(39.2814867845705,-5.62462426065916,-9.2116921688142));
#67577=CARTESIAN_POINT('Ctrl Pts',(39.4005509074198,-0.533392711710504,
-10.779942620519));
#67578=CARTESIAN_POINT('Ctrl Pts',(39.5196150302689,4.68778556012255,-9.72195130768049));
#67579=CARTESIAN_POINT('Ctrl Pts',(39.6386791531182,8.76691153588649,-6.29546922861956));
#67580=CARTESIAN_POINT('Ctrl Pts',(39.7577432759673,10.7102163823515,-1.33526616442953));
#67581=CARTESIAN_POINT('Ctrl Pts',(39.8768073988166,10.0442663783095,3.95023842420271));
#67582=CARTESIAN_POINT('Ctrl Pts',(39.9958715216657,6.93130224949493,8.2733741492109));
#67583=CARTESIAN_POINT('Ctrl Pts',(40.1149356445149,2.12971359904549,10.5809257946881));
#67584=CARTESIAN_POINT('Ctrl Pts',(40.2339997673641,-3.19072222863013,10.3107207481211));
#67585=CARTESIAN_POINT('Ctrl Pts',(40.3530638902133,-7.73382479314201,7.52858716873846));
#67586=CARTESIAN_POINT('Ctrl Pts',(40.4721280130625,-10.3927899006936,2.91231673465592));
#67587=CARTESIAN_POINT('Ctrl Pts',(40.5911921359116,-10.5198325443847,-2.41346098595686));
#67588=CARTESIAN_POINT('Ctrl Pts',(40.7102562587609,-8.08400221455837,-7.15126414522724));
#67589=CARTESIAN_POINT('Ctrl Pts',(40.82932038161,-3.67872316309958,-10.1468550091328));
#67590=CARTESIAN_POINT('Ctrl Pts',(40.9483845044593,1.62277739935709,-10.6704388017726));
#67591=CARTESIAN_POINT('Ctrl Pts',(41.0674486273084,6.52893208358652,-8.59445847348277));
#67592=CARTESIAN_POINT('Ctrl Pts',(41.1865127501576,9.84448888406489,-4.42467055139305));
#67593=CARTESIAN_POINT('Ctrl Pts',(41.3055768730069,10.7617019133518,0.823068815814848));
#67594=CARTESIAN_POINT('Ctrl Pts',(41.424640995856,9.05711710161736,5.87028968067695));
#67595=CARTESIAN_POINT('Ctrl Pts',(41.5437051187052,5.14601028387998,9.48737311454202));
#67596=CARTESIAN_POINT('Ctrl Pts',(41.6627692415544,-0.0187826495503634,
10.7931143343773));
#67597=CARTESIAN_POINT('Ctrl Pts',(41.7818333644036,-5.1790001883043,9.46940502488953));
#67598=CARTESIAN_POINT('Ctrl Pts',(41.9008974872528,-9.07749331133013,5.83873070423811));
#67599=CARTESIAN_POINT('Ctrl Pts',(42.019961610102,-10.7645022764989,0.785608024301024));
#67600=CARTESIAN_POINT('Ctrl Pts',(42.1390257329511,-9.82902756568768,-4.45890803155238));
#67601=CARTESIAN_POINT('Ctrl Pts',(42.2580898558004,-6.49898267765482,-8.61712928683789));
#67602=CARTESIAN_POINT('Ctrl Pts',(42.3771539786495,-1.58562306597511,-10.6760243123689));
#67603=CARTESIAN_POINT('Ctrl Pts',(42.4962181014987,3.71400529704884,-10.133985766706));
#67604=CARTESIAN_POINT('Ctrl Pts',(42.6152822243479,8.1088658084942,-7.12309218598227));
#67605=CARTESIAN_POINT('Ctrl Pts',(42.7343463471971,10.5281252274973,-2.37681720430857));
#67606=CARTESIAN_POINT('Ctrl Pts',(42.8534104700464,10.3826749940061,2.94844237261853));
#67607=CARTESIAN_POINT('Ctrl Pts',(42.9724745928955,7.70741127480427,7.55551505879895));
#67608=CARTESIAN_POINT('Ctrl Pts',(43.0915387157447,3.15513697811894,10.3216529484319));
#67609=CARTESIAN_POINT('Ctrl Pts',(43.2106028385939,-2.16719331179086,10.5736883120838));
#67610=CARTESIAN_POINT('Ctrl Pts',(43.2899789204934,-5.36128729434186,9.02356846987115));
#67611=CARTESIAN_POINT('Ctrl Pts',(43.3296669614431,-6.67687804941313,7.91357169861802));
#67612=CARTESIAN_POINT('Ctrl Pts',(0.155159788455616,-9.87377947543221,
1.97057634221972));
#67613=CARTESIAN_POINT('Ctrl Pts',(0.194847829405346,-10.2013776974132,
0.329111086049827));
#67614=CARTESIAN_POINT('Ctrl Pts',(0.274223911304807,-10.021840249213,-3.11868739370281));
#67615=CARTESIAN_POINT('Ctrl Pts',(0.393288034153999,-7.30843550280246,
-7.53276225684153));
#67616=CARTESIAN_POINT('Ctrl Pts',(0.512352157003191,-2.81559820488554,
-10.1107273584017));
#67617=CARTESIAN_POINT('Ctrl Pts',(0.631416279852383,2.36371079283422,-10.2259645636769));
#67618=CARTESIAN_POINT('Ctrl Pts',(0.750480402701574,6.96689532650368,-7.84967628098838));
#67619=CARTESIAN_POINT('Ctrl Pts',(0.869544525550766,9.87292364246029,-3.56115337744866));
#67620=CARTESIAN_POINT('Ctrl Pts',(0.988608648399958,10.373608620426,1.59501402068791));
#67621=CARTESIAN_POINT('Ctrl Pts',(1.10767277124915,8.34708153225567,6.36256533997802));
#67622=CARTESIAN_POINT('Ctrl Pts',(1.22673689409834,4.28699419088582,9.58006712539813));
#67623=CARTESIAN_POINT('Ctrl Pts',(1.34580101694754,-0.817493434454986,
10.463635277209));
#67624=CARTESIAN_POINT('Ctrl Pts',(1.46486513979672,-5.72282606115532,8.79802612159381));
#67625=CARTESIAN_POINT('Ctrl Pts',(1.58392926264592,-9.23394405199729,4.98901316541469));
#67626=CARTESIAN_POINT('Ctrl Pts',(1.70299338549511,-10.4954624503197,-0.0354367893760476));
#67627=CARTESIAN_POINT('Ctrl Pts',(1.8220575083443,-9.20004427129698,-5.05125418271118));
#67628=CARTESIAN_POINT('Ctrl Pts',(1.94112163119349,-5.6632842472853,-8.83646963134304));
#67629=CARTESIAN_POINT('Ctrl Pts',(2.06018575404269,-0.74681783530992,-10.4689181755661));
#67630=CARTESIAN_POINT('Ctrl Pts',(2.17924987689187,4.35159046461578,-9.55089756705936));
#67631=CARTESIAN_POINT('Ctrl Pts',(2.29831399974107,8.38985137183536,-6.30605886170975));
#67632=CARTESIAN_POINT('Ctrl Pts',(2.41737812259025,10.3841516444387,-1.52491926888339));
#67633=CARTESIAN_POINT('Ctrl Pts',(2.53644224543945,9.84863394411602,3.62772569058057));
#67634=CARTESIAN_POINT('Ctrl Pts',(2.65550636828864,6.91376266876593,7.89657330678198));
#67635=CARTESIAN_POINT('Ctrl Pts',(2.77457049113784,2.29453992050261,10.2416341848227));
#67636=CARTESIAN_POINT('Ctrl Pts',(2.89363461398702,-2.88368548691312,10.0915976062867));
#67637=CARTESIAN_POINT('Ctrl Pts',(3.01269873683622,-7.35937883651767,7.48301592715619));
#67638=CARTESIAN_POINT('Ctrl Pts',(3.13176285968541,-10.0421583704944,3.05139959567209));
#67639=CARTESIAN_POINT('Ctrl Pts',(3.2508269825346,-10.2784373385558,-2.12360780413088));
#67640=CARTESIAN_POINT('Ctrl Pts',(3.36989110538379,-8.01065275437778,-6.78125553845112));
#67641=CARTESIAN_POINT('Ctrl Pts',(3.48895522823299,-3.79128906016513,-9.78683357839978));
#67642=CARTESIAN_POINT('Ctrl Pts',(3.60801935108218,1.35171977960818,-10.4081140398368));
#67643=CARTESIAN_POINT('Ctrl Pts',(3.72708347393137,6.16541861617209,-8.49373872428129));
#67644=CARTESIAN_POINT('Ctrl Pts',(3.84614759678056,9.47707978558044,-4.51009345431341));
#67645=CARTESIAN_POINT('Ctrl Pts',(3.96521171962975,10.4799065191379,0.572314231060847));
#67646=CARTESIAN_POINT('Ctrl Pts',(4.08427584247894,8.92958717780655,5.51529301695582));
#67647=CARTESIAN_POINT('Ctrl Pts',(4.20333996532814,5.20381518222463,9.11461967271146));
#67648=CARTESIAN_POINT('Ctrl Pts',(4.32240408817732,0.210274215357055,10.4934155060823));
#67649=CARTESIAN_POINT('Ctrl Pts',(4.44146821102652,-4.83449438284527,9.31577416488656));
#67650=CARTESIAN_POINT('Ctrl Pts',(4.56053233387571,-8.70146904413809,5.86859614412498));
#67651=CARTESIAN_POINT('Ctrl Pts',(4.6795964567249,-10.4485658710995,0.991693231914828));
#67652=CARTESIAN_POINT('Ctrl Pts',(4.7986605795741,-9.65015192530062,-4.12680894245765));
#67653=CARTESIAN_POINT('Ctrl Pts',(4.91772470242328,-6.50073919290531,-8.23992561706452));
#67654=CARTESIAN_POINT('Ctrl Pts',(5.03678882527248,-1.76759699461112,-10.3456070432611));
#67655=CARTESIAN_POINT('Ctrl Pts',(5.15585294812166,3.39617245408182,-9.93086083333501));
#67656=CARTESIAN_POINT('Ctrl Pts',(5.27491707097087,7.73255624289876,-7.09672869562723));
#67657=CARTESIAN_POINT('Ctrl Pts',(5.39398119382005,10.1851116230995,-2.53367035226248));
#67658=CARTESIAN_POINT('Ctrl Pts',(5.51304531666925,10.1563397399983,2.64664831714824));
#67659=CARTESIAN_POINT('Ctrl Pts',(5.63210943951844,7.65325008554719,7.18218263183298));
#67660=CARTESIAN_POINT('Ctrl Pts',(5.75117356236763,3.28565282500688,9.96797219811811));
#67661=CARTESIAN_POINT('Ctrl Pts',(5.87023768521683,-1.8824049738298,10.3253346552754));
#67662=CARTESIAN_POINT('Ctrl Pts',(5.989301808066,-6.59186566003927,8.16720829591889));
#67663=CARTESIAN_POINT('Ctrl Pts',(6.10836593091521,-9.69539637870831,4.01936229875602));
#67664=CARTESIAN_POINT('Ctrl Pts',(6.22743005376439,-10.4369057221332,-1.10769272645255));
#67665=CARTESIAN_POINT('Ctrl Pts',(6.34649417661359,-8.63574497305666,-5.96488834675535));
#67666=CARTESIAN_POINT('Ctrl Pts',(6.46555829946278,-4.73071828381995,-9.36890008208345));
#67667=CARTESIAN_POINT('Ctrl Pts',(6.58462242231197,0.326820099645189,-10.4904324434886));
#67668=CARTESIAN_POINT('Ctrl Pts',(6.70368654516116,5.30473759593165,-9.05625437293148));
#67669=CARTESIAN_POINT('Ctrl Pts',(6.82275066801036,8.99029910157828,-5.41576460835333));
#67670=CARTESIAN_POINT('Ctrl Pts',(6.94181479085954,10.4856171330745,-0.45587012131181));
#67671=CARTESIAN_POINT('Ctrl Pts',(7.06087891370874,9.42639785288965,4.61508480398452));
#67672=CARTESIAN_POINT('Ctrl Pts',(7.17994303655793,6.07069142041281,8.56169900820262));
#67673=CARTESIAN_POINT('Ctrl Pts',(7.29900715940712,1.23602504267618,10.4224865710064));
#67674=CARTESIAN_POINT('Ctrl Pts',(7.41807128225631,-3.89976544150229,9.74411687790103));
#67675=CARTESIAN_POINT('Ctrl Pts',(7.5371354051055,-8.0854834406099,6.69185637626472));
#67676=CARTESIAN_POINT('Ctrl Pts',(7.65619952795469,-10.3013918548464,2.00930587065153));
#67677=CARTESIAN_POINT('Ctrl Pts',(7.7752636508039,-10.0076444690016,-3.16275772246214));
#67678=CARTESIAN_POINT('Ctrl Pts',(7.89432777365307,-7.27580489710256,-7.56430084860656));
#67679=CARTESIAN_POINT('Ctrl Pts',(8.01339189650228,-2.77141204137876,-10.1230064469915));
#67680=CARTESIAN_POINT('Ctrl Pts',(8.13245601935145,2.40816047958505,-10.2155150302614));
#67681=CARTESIAN_POINT('Ctrl Pts',(8.25152014220066,7.00104976392646,-7.81928938152035));
#67682=CARTESIAN_POINT('Ctrl Pts',(8.37058426504984,9.88832242924462,-3.51810513831368));
#67683=CARTESIAN_POINT('Ctrl Pts',(8.48964838789904,10.3665724996254,1.640170368877));
#67684=CARTESIAN_POINT('Ctrl Pts',(8.60871251074823,8.31928726688984,6.39886268018749));
#67685=CARTESIAN_POINT('Ctrl Pts',(8.72777663359742,4.2452324639752,9.59864498539987));
#67686=CARTESIAN_POINT('Ctrl Pts',(8.84684075644661,-0.863058530129139,
10.4599767782965));
#67687=CARTESIAN_POINT('Ctrl Pts',(8.96590487929581,-5.76108863167953,8.77301783919674));
#67688=CARTESIAN_POINT('Ctrl Pts',(9.084969002145,-9.25558514252632,4.94875013497122));
#67689=CARTESIAN_POINT('Ctrl Pts',(9.20403312499418,-10.4952084029044,-0.0811468331815238));
#67690=CARTESIAN_POINT('Ctrl Pts',(9.32309724784339,-9.17795769784646,-5.09127456787318));
#67691=CARTESIAN_POINT('Ctrl Pts',(9.44216137069257,-5.62474557186012,-8.86105081131867));
#67692=CARTESIAN_POINT('Ctrl Pts',(9.56122549354177,-0.701216157947351,
-10.4720714344758));
#67693=CARTESIAN_POINT('Ctrl Pts',(9.68028961639095,4.39314562723144,-9.53185478943469));
#67694=CARTESIAN_POINT('Ctrl Pts',(9.79935373924015,8.41723617534466,-6.26945925877189));
#67695=CARTESIAN_POINT('Ctrl Pts',(9.91841786208933,10.3906945481397,-1.47967936938784));
#67696=CARTESIAN_POINT('Ctrl Pts',(10.0374819849385,9.83274093243286,3.67058442003326));
#67697=CARTESIAN_POINT('Ctrl Pts',(10.1565461077877,6.87930565177331,7.92660948819928));
#67698=CARTESIAN_POINT('Ctrl Pts',(10.2756102306369,2.24991341570653,10.2515303175065));
#67699=CARTESIAN_POINT('Ctrl Pts',(10.3946743534861,-2.92760943542397,10.0789427631348));
#67700=CARTESIAN_POINT('Ctrl Pts',(10.5137384763353,-7.39189934643209,7.450893119697));
#67701=CARTESIAN_POINT('Ctrl Pts',(10.6328025991845,-10.0553526977025,3.00763467757269));
#67702=CARTESIAN_POINT('Ctrl Pts',(10.7518667220337,-10.2690910419876,-2.16835269278329));
#67703=CARTESIAN_POINT('Ctrl Pts',(10.8709308448829,-7.98104280653367,-6.81607951458966));
#67704=CARTESIAN_POINT('Ctrl Pts',(10.9899949677321,-3.74862912490046,-9.80325272105535));
#67705=CARTESIAN_POINT('Ctrl Pts',(11.1090590905813,1.39703676169904,-10.4021282685512));
#67706=CARTESIAN_POINT('Ctrl Pts',(11.2281232134305,6.20235238676807,-8.46680631048589));
#67707=CARTESIAN_POINT('Ctrl Pts',(11.3471873362796,9.49663242937081,-4.4687757529724));
#67708=CARTESIAN_POINT('Ctrl Pts',(11.4662514591288,10.4773145627358,0.617951278351491));
#67709=CARTESIAN_POINT('Ctrl Pts',(11.585315581978,8.90548208136188,5.55413117665345));
#67710=CARTESIAN_POINT('Ctrl Pts',(11.7043797048272,5.1640695012078,9.13719707654523));
#67711=CARTESIAN_POINT('Ctrl Pts',(11.8234438276764,0.164570911090679,10.4942317796089));
#67712=CARTESIAN_POINT('Ctrl Pts',(11.9425079505256,-4.87502093509933,9.29463044511586));
#67713=CARTESIAN_POINT('Ctrl Pts',(12.0615720733748,-8.72694564487861,5.83064352711308));
#67714=CARTESIAN_POINT('Ctrl Pts',(12.180636196224,-10.4527858348887,0.946177847384331));
#67715=CARTESIAN_POINT('Ctrl Pts',(12.2997003190732,-9.63208717197718,-4.16879850081101));
#67716=CARTESIAN_POINT('Ctrl Pts',(12.4187644419224,-6.4647907115389,-8.26815972783132));
#67717=CARTESIAN_POINT('Ctrl Pts',(12.5378285647716,-1.72252266142237,-10.3532072281887));
#67718=CARTESIAN_POINT('Ctrl Pts',(12.6568926876207,3.43939149564005,-9.91597551270928));
#67719=CARTESIAN_POINT('Ctrl Pts',(12.7759568104699,7.76339084105272,-7.06298427564369));
#67720=CARTESIAN_POINT('Ctrl Pts',(12.8950209333191,10.1960497611052,-2.48928774913569));
#67721=CARTESIAN_POINT('Ctrl Pts',(13.0140850561683,10.1447166360597,2.69085648130572));
#67722=CARTESIAN_POINT('Ctrl Pts',(13.1331491790175,7.62189739490336,7.21544623225042));
#67723=CARTESIAN_POINT('Ctrl Pts',(13.2522133018667,3.242208783639,9.98218745727736));
#67724=CARTESIAN_POINT('Ctrl Pts',(13.3712774247159,-1.92735639902351,10.3170384093535));
#67725=CARTESIAN_POINT('Ctrl Pts',(13.4903415475651,-6.62737326881817,8.13842170108466));
#67726=CARTESIAN_POINT('Ctrl Pts',(13.6094056704143,-9.71280970154605,3.97709843107813));
#67727=CARTESIAN_POINT('Ctrl Pts',(13.7284697932635,-10.4319824733975,-1.15313741750913));
#67728=CARTESIAN_POINT('Ctrl Pts',(13.8475339161127,-8.60968456928456,-6.00244249004976));
#67729=CARTESIAN_POINT('Ctrl Pts',(13.9665980389618,-4.68986963828456,-9.38941462524836));
#67730=CARTESIAN_POINT('Ctrl Pts',(14.0856621618111,0.372505318117175,-10.4889095723486));
#67731=CARTESIAN_POINT('Ctrl Pts',(14.2047262846602,5.34412941819326,-9.03306509389438));
#67732=CARTESIAN_POINT('Ctrl Pts',(14.3237904075095,9.0138007744326,-5.37655836272329));
#67733=CARTESIAN_POINT('Ctrl Pts',(14.4428545303586,10.4875031089042,-0.410198451553393));
#67734=CARTESIAN_POINT('Ctrl Pts',(14.5619186532078,9.40620866463942,4.65609522950223));
#67735=CARTESIAN_POINT('Ctrl Pts',(14.680982776057,6.03334561832389,8.58805710733127));
#67736=CARTESIAN_POINT('Ctrl Pts',(14.8000468989062,1.19062092241009,10.4277709050425));
#67737=CARTESIAN_POINT('Ctrl Pts',(14.9191110217554,-3.94216639278166,9.72704006162999));
#67738=CARTESIAN_POINT('Ctrl Pts',(15.0381751446046,-8.1145513767218,6.65657871458557));
#67739=CARTESIAN_POINT('Ctrl Pts',(15.1572392674538,-10.3100451585213,1.96442181269258));
#67740=CARTESIAN_POINT('Ctrl Pts',(15.276303390303,-9.99377499659597,-3.20631338866685));
#67741=CARTESIAN_POINT('Ctrl Pts',(15.3953675131521,-7.24279157083963,-7.5959169617832));
#67742=CARTESIAN_POINT('Ctrl Pts',(15.5144316360014,-2.72729766624086,-10.134980595376));
#67743=CARTESIAN_POINT('Ctrl Pts',(15.6334957588506,2.45262862798792,-10.2049300361201));
#67744=CARTESIAN_POINT('Ctrl Pts',(15.7525598816997,7.03503822268641,-7.78872399268793));
#67745=CARTESIAN_POINT('Ctrl Pts',(15.8716240045489,9.90355082869269,-3.47500578595657));
#67746=CARTESIAN_POINT('Ctrl Pts',(15.9906881273981,10.3593308516804,1.68530369202511));
#67747=CARTESIAN_POINT('Ctrl Pts',(16.1097522502473,8.29133980341716,6.43503445936399));
#67748=CARTESIAN_POINT('Ctrl Pts',(16.2288163730965,4.20338782935896,9.61704294390578));
#67749=CARTESIAN_POINT('Ctrl Pts',(16.3478804959457,-0.908606021232575,
10.4561187506221));
#67750=CARTESIAN_POINT('Ctrl Pts',(16.4669446187949,-5.79924256367529,8.74784372954778));
#67751=CARTESIAN_POINT('Ctrl Pts',(16.5860087416441,-9.27705034073521,4.90839293500387));
#67752=CARTESIAN_POINT('Ctrl Pts',(16.7050728644933,-10.4947554517345,-0.126855182075213));
#67753=CARTESIAN_POINT('Ctrl Pts',(16.8241369873425,-9.15569694661239,-5.13119846144389));
#67754=CARTESIAN_POINT('Ctrl Pts',(16.9432011101916,-5.58610025115397,-8.88546387157073));
#67755=CARTESIAN_POINT('Ctrl Pts',(17.0622652330409,-0.655601156031094,
-10.4750260788765));
#67756=CARTESIAN_POINT('Ctrl Pts',(17.18132935589,4.43461744757741,-9.51263119870489));
#67757=CARTESIAN_POINT('Ctrl Pts',(17.3003934787392,8.4444613255881,-6.23274074140566));
#67758=CARTESIAN_POINT('Ctrl Pts',(17.4194576015884,10.3970403559991,-1.43441140007221));
#67759=CARTESIAN_POINT('Ctrl Pts',(17.5385217244376,9.81666141327586,3.71337352363487));
#67760=CARTESIAN_POINT('Ctrl Pts',(17.6575858472868,6.84471814600233,7.9564953170801));
#67761=CARTESIAN_POINT('Ctrl Pts',(17.776649970136,2.20524423460953,10.2612319969219));
#67762=CARTESIAN_POINT('Ctrl Pts',(17.8957140929852,-2.97147785275479,10.0660967410173));
#67763=CARTESIAN_POINT('Ctrl Pts',(18.0147782158344,-7.42427964536093,7.41862898225881));
#67764=CARTESIAN_POINT('Ctrl Pts',(18.1338423386836,-10.0683562932537,2.96381271018086));
#67765=CARTESIAN_POINT('Ctrl Pts',(18.2529064615328,-10.2595499594392,-2.21305645176568));
#67766=CARTESIAN_POINT('Ctrl Pts',(18.3719705843819,-7.95128147286543,-6.85077420210285));
#67767=CARTESIAN_POINT('Ctrl Pts',(18.4910347072312,-3.70589808496221,-9.81948591387579));
#67768=CARTESIAN_POINT('Ctrl Pts',(18.6100988300803,1.44232724454336,-10.3959451878403));
#67769=CARTESIAN_POINT('Ctrl Pts',(18.7291629529295,6.23916851004201,-8.43971329680288));
#67770=CARTESIAN_POINT('Ctrl Pts',(18.8482270757787,9.51600493934509,-4.427373287096));
#67771=CARTESIAN_POINT('Ctrl Pts',(18.9672911986279,10.4745238707661,0.663576604231755));
#67772=CARTESIAN_POINT('Ctrl Pts',(19.0863553214771,8.88120806414699,5.59286398460229));
#67773=CARTESIAN_POINT('Ctrl Pts',(19.2054194443263,5.12422586720129,9.15960116439776));
#67774=CARTESIAN_POINT('Ctrl Pts',(19.3244835671755,0.118864485213787,10.4948489966786));
#67775=CARTESIAN_POINT('Ctrl Pts',(19.4435476900247,-4.91545501708828,9.27331042313978));
#67776=CARTESIAN_POINT('Ctrl Pts',(19.5626118128739,-8.75225671136026,5.79258031341651));
#67777=CARTESIAN_POINT('Ctrl Pts',(19.6816759357231,-10.456807528375,0.900644515583848));
#67778=CARTESIAN_POINT('Ctrl Pts',(19.8007400585722,-9.61383971550915,-4.21070898465213));
#67779=CARTESIAN_POINT('Ctrl Pts',(19.9198041814215,-6.42871960487108,-8.29623700667221));
#67780=CARTESIAN_POINT('Ctrl Pts',(20.0388683042706,-1.677415655117,-10.360611031638));
#67781=CARTESIAN_POINT('Ctrl Pts',(20.1579324271198,3.48254529820804,-9.90090210409437));
#67782=CARTESIAN_POINT('Ctrl Pts',(20.276996549969,7.79407818182693,-7.02910588371671));
#67783=CARTESIAN_POINT('Ctrl Pts',(20.3960606728182,10.2067944986236,-2.44485792875554));
#67784=CARTESIAN_POINT('Ctrl Pts',(20.5151247956674,10.1329011053296,2.73501360481841));
#67785=CARTESIAN_POINT('Ctrl Pts',(20.6341889185166,7.5904001307525,7.24857296879903));
#67786=CARTESIAN_POINT('Ctrl Pts',(20.7532530413658,3.19870324347748,9.99621337252753));
#67787=CARTESIAN_POINT('Ctrl Pts',(20.872317164215,-1.97227126577789,10.3085464680098));
#67788=CARTESIAN_POINT('Ctrl Pts',(20.9913812870642,-6.66275516840085,8.10948073521845));
#67789=CARTESIAN_POINT('Ctrl Pts',(21.1104454099134,-9.73003879007993,3.93475912508902));
#67790=CARTESIAN_POINT('Ctrl Pts',(21.2295095327626,-10.4268613489607,-1.19856023564992));
#67791=CARTESIAN_POINT('Ctrl Pts',(21.3485736556117,-8.58346085548246,-6.03988277794626));
#67792=CARTESIAN_POINT('Ctrl Pts',(21.467637778461,-4.64893203446674,-9.40975106832484));
#67793=CARTESIAN_POINT('Ctrl Pts',(21.5867019013101,0.41818347084202,-10.4871877457041));
#67794=CARTESIAN_POINT('Ctrl Pts',(21.7057660241593,5.38341987205639,-9.00970447407017));
#67795=CARTESIAN_POINT('Ctrl Pts',(21.8248301470085,9.03713147190878,-5.33725013357698));
#67796=CARTESIAN_POINT('Ctrl Pts',(21.9438942698577,10.4891901559074,-0.364519001077752));
#67797=CARTESIAN_POINT('Ctrl Pts',(22.0629583927069,9.38584105774835,4.69701733737661));
#67798=CARTESIAN_POINT('Ctrl Pts',(22.1820225155561,5.99588537466088,8.6142523066636));
#67799=CARTESIAN_POINT('Ctrl Pts',(22.3010866384053,1.14519421823428,10.4328574432633));
#67800=CARTESIAN_POINT('Ctrl Pts',(22.4201507612545,-3.98449256834685,9.70977874113103));
#67801=CARTESIAN_POINT('Ctrl Pts',(22.5392148841037,-8.14346539457826,6.6211747897362));
#67802=CARTESIAN_POINT('Ctrl Pts',(22.6582790069529,-10.3185028994238,1.91950049323095));
#67803=CARTESIAN_POINT('Ctrl Pts',(22.777343129802,-9.97971596048673,-3.24980823694837));
#67804=CARTESIAN_POINT('Ctrl Pts',(22.8964072526512,-7.20964086201644,-7.62738899425446));
#67805=CARTESIAN_POINT('Ctrl Pts',(23.0154713755005,-2.68313155923512,-10.1467625016439));
#67806=CARTESIAN_POINT('Ctrl Pts',(23.1345354983496,2.49705025449416,-10.1941514730488));
#67807=CARTESIAN_POINT('Ctrl Pts',(23.2535996211988,7.06889323958863,-7.75801086595204));
#67808=CARTESIAN_POINT('Ctrl Pts',(23.372663744048,9.91859137582519,-3.43184051907101));
#67809=CARTESIAN_POINT('Ctrl Pts',(23.4917278668972,10.3518927061033,1.73040504803268));
#67810=CARTESIAN_POINT('Ctrl Pts',(23.6107919897464,8.26323506833476,6.47108417766095));
#67811=CARTESIAN_POINT('Ctrl Pts',(23.7298561125956,4.16146346413405,9.63525848462867));
#67812=CARTESIAN_POINT('Ctrl Pts',(23.8489202354448,-0.954136277735047,
10.4520623894254));
#67813=CARTESIAN_POINT('Ctrl Pts',(23.967984358294,-5.83728649460537,8.72250368924138));
#67814=CARTESIAN_POINT('Ctrl Pts',(24.0870484811432,-9.29833957020137,4.86794263176538));
#67815=CARTESIAN_POINT('Ctrl Pts',(24.2061126039923,-10.4941034341745,-0.172561124757199));
#67816=CARTESIAN_POINT('Ctrl Pts',(24.3251767268415,-9.13326252848837,-5.17102502552844));
#67817=CARTESIAN_POINT('Ctrl Pts',(24.4442408496907,-5.54734897230373,-8.90970839076184));
#67818=CARTESIAN_POINT('Ctrl Pts',(24.5633049725399,-0.609973718555534,
-10.4777820311172));
#67819=CARTESIAN_POINT('Ctrl Pts',(24.6823690953891,4.47600515130988,-9.49322717069275));
#67820=CARTESIAN_POINT('Ctrl Pts',(24.8014332182383,8.47152629978549,-6.19590400030329));
#67821=CARTESIAN_POINT('Ctrl Pts',(24.9204973410875,10.4031889509458,-1.38911622258575));
#67822=CARTESIAN_POINT('Ctrl Pts',(25.0395614639367,9.80039568993721,3.7560921913062));
#67823=CARTESIAN_POINT('Ctrl Pts',(25.1586255867859,6.81000080839887,7.98623022574092));
#67824=CARTESIAN_POINT('Ctrl Pts',(25.2776897096351,2.16053322404739,10.2707390394615));
#67825=CARTESIAN_POINT('Ctrl Pts',(25.3967538324842,-3.01528990656447,10.0530597833845));
#67826=CARTESIAN_POINT('Ctrl Pts',(25.5158179553335,-7.45651911923148,7.38622412694516));
#67827=CARTESIAN_POINT('Ctrl Pts',(25.6348820781826,-10.0811689104299,2.91993452466181));
#67828=CARTESIAN_POINT('Ctrl Pts',(25.7539462010319,-10.2498142719204,-2.25771823309913));
#67829=CARTESIAN_POINT('Ctrl Pts',(25.873010323881,-7.92136931787451,-6.88533894291106));
#67830=CARTESIAN_POINT('Ctrl Pts',(25.9920744467302,-3.66309675088932,-9.83553284893887));
#67831=CARTESIAN_POINT('Ctrl Pts',(26.1111385695794,1.48759036906762,-10.3895649149899));
#67832=CARTESIAN_POINT('Ctrl Pts',(26.2302026924286,6.27586628765668,-8.41246019713529));
#67833=CARTESIAN_POINT('Ctrl Pts',(26.3492668152778,9.53519694804324,-4.38588684201477));
#67834=CARTESIAN_POINT('Ctrl Pts',(26.468330938127,10.4715344961624,0.709189343272753));
#67835=CARTESIAN_POINT('Ctrl Pts',(26.5873950609762,8.85676558659625,5.63149070611111));
#67836=CARTESIAN_POINT('Ctrl Pts',(26.7064591838254,5.08428503596618,9.18183151130437));
#67837=CARTESIAN_POINT('Ctrl Pts',(26.8255233066746,0.0731558046942684,
10.4952671455838));
#67838=CARTESIAN_POINT('Ctrl Pts',(26.9445874295238,-4.95579586185122,9.25181450336041));
#67839=CARTESIAN_POINT('Ctrl Pts',(27.063651552373,-8.77740176347816,5.75440722502514));
#67840=CARTESIAN_POINT('Ctrl Pts',(27.1827156752221,-10.4606308752741,0.855094100197905));
#67841=CARTESIAN_POINT('Ctrl Pts',(27.3017797980713,-9.5954099020176,-4.25253959901537));
#67842=CARTESIAN_POINT('Ctrl Pts',(27.4208439209205,-6.39252655710521,-8.32415692101224));
#67843=CARTESIAN_POINT('Ctrl Pts',(27.5399080437697,-1.63227683129287,-10.3678183131726));
#67844=CARTESIAN_POINT('Ctrl Pts',(27.6589721666189,3.5256330432367,-9.88564089340539));
#67845=CARTESIAN_POINT('Ctrl Pts',(27.7780362894681,7.82461768313833,-6.99509416245773));
#67846=CARTESIAN_POINT('Ctrl Pts',(27.8971004123173,10.2173456318464,-2.40038173387489));
#67847=CARTESIAN_POINT('Ctrl Pts',(28.0161645351665,10.120893371927,2.77911885010604));
#67848=CARTESIAN_POINT('Ctrl Pts',(28.1352286580157,7.55875889054041,7.28156221312484));
#67849=CARTESIAN_POINT('Ctrl Pts',(28.2542927808649,3.1551370297433,10.0100496778225));
#67850=CARTESIAN_POINT('Ctrl Pts',(28.3733569037141,-2.01714872213973,10.2998589923213));
#67851=CARTESIAN_POINT('Ctrl Pts',(28.4924210265632,-6.69801068765711,8.08038594727766));
#67852=CARTESIAN_POINT('Ctrl Pts',(28.6114851494124,-9.74708331750548,3.8923451838882));
#67853=CARTESIAN_POINT('Ctrl Pts',(28.7305492722616,-10.4215424459612,-1.24396031928669));
#67854=CARTESIAN_POINT('Ctrl Pts',(28.8496133951108,-8.55707432906648,-6.07720850027072));
#67855=CARTESIAN_POINT('Ctrl Pts',(28.96867751796,-4.60790624887834,-9.42990902556751));
#67856=CARTESIAN_POINT('Ctrl Pts',(29.0877416408092,0.463853691388278,-10.4852669962151));
#67857=CARTESIAN_POINT('Ctrl Pts',(29.2068057636584,5.42260821225282,-8.98617295656719));
#67858=CARTESIAN_POINT('Ctrl Pts',(29.3258698865076,9.060290751466,-5.29784066651983));
#67859=CARTESIAN_POINT('Ctrl Pts',(29.4449340093568,10.490678242084,-0.318832636340938));
#67860=CARTESIAN_POINT('Ctrl Pts',(29.563998132206,9.36529541855293,4.73785035138961));
#67861=CARTESIAN_POINT('Ctrl Pts',(29.6830622550552,5.95831139997658,8.64028410932423));
#67862=CARTESIAN_POINT('Ctrl Pts',(29.8021263779044,1.09974579181068,10.4377460891864));
#67863=CARTESIAN_POINT('Ctrl Pts',(29.9211905007536,-4.02674316534753,9.69233324382));
#67864=CARTESIAN_POINT('Ctrl Pts',(30.0402546236027,-8.17222494573302,6.58564527326446));
#67865=CARTESIAN_POINT('Ctrl Pts',(30.1593187464519,-10.3267649171259,1.87454276434232));
#67866=CARTESIAN_POINT('Ctrl Pts',(30.2783828693011,-9.96546762734824,-3.29324144228838));
#67867=CARTESIAN_POINT('Ctrl Pts',(30.3974469921503,-7.17635339944174,-7.65871634905305));
#67868=CARTESIAN_POINT('Ctrl Pts',(30.5165111149995,-2.63891455811226,-10.158351942314));
#67869=CARTESIAN_POINT('Ctrl Pts',(30.6355752378487,2.54142451650656,-10.1831795454971));
#67870=CARTESIAN_POINT('Ctrl Pts',(30.7546393606979,7.10261417246512,-7.72715058388468));
#67871=CARTESIAN_POINT('Ctrl Pts',(30.8737034835471,9.9334437853503,-3.38861015642353));
#67872=CARTESIAN_POINT('Ctrl Pts',(30.9927676063963,10.3442582039821,1.77547358140902));
#67873=CARTESIAN_POINT('Ctrl Pts',(31.1118317292455,8.23497359473827,6.50701115128098));
#67874=CARTESIAN_POINT('Ctrl Pts',(31.2308958520947,4.11946016352903,9.65329126205301));
#67875=CARTESIAN_POINT('Ctrl Pts',(31.3499599749439,-0.99964843601095,10.4478077716482));
#67876=CARTESIAN_POINT('Ctrl Pts',(31.4690240977931,-5.87521970284595,8.69699819893175));
#67877=CARTESIAN_POINT('Ctrl Pts',(31.5880882206422,-9.31945242710681,4.82739999252429));
#67878=CARTESIAN_POINT('Ctrl Pts',(31.7071523434915,-10.493252362592,-0.218263794268897));
#67879=CARTESIAN_POINT('Ctrl Pts',(31.8262164663406,-9.1106548690145,-5.21075350468951));
#67880=CARTESIAN_POINT('Ctrl Pts',(31.9452805891898,-5.50849247035029,-8.93378390901784));
#67881=CARTESIAN_POINT('Ctrl Pts',(32.064344712039,-0.564334710989629,-10.4803392389227));
#67882=CARTESIAN_POINT('Ctrl Pts',(32.1834088348883,4.51730795337978,-9.47364307345718));
#67883=CARTESIAN_POINT('Ctrl Pts',(32.3024729577373,8.49843058456348,-6.1589497341906));
#67884=CARTESIAN_POINT('Ctrl Pts',(32.4215370805866,10.409140216352,-1.34379469609559));
#67885=CARTESIAN_POINT('Ctrl Pts',(32.5406012034357,9.7839440709481,3.79873961275201));
#67886=CARTESIAN_POINT('Ctrl Pts',(32.659665326285,6.7751542974874,8.01581365016488));
#67887=CARTESIAN_POINT('Ctrl Pts',(32.7787294491341,2.1157812321061,10.2800512647943));
#67888=CARTESIAN_POINT('Ctrl Pts',(32.8977935719833,-3.05904476581843,10.0398321375235));
#67889=CARTESIAN_POINT('Ctrl Pts',(33.0168576948326,-7.48861715651959,7.35367916841708));
#67890=CARTESIAN_POINT('Ctrl Pts',(33.1359218176817,-10.0937903061991,2.87600095330493));
#67891=CARTESIAN_POINT('Ctrl Pts',(33.254985940531,-10.2398841640994,-2.3023371896311));
#67892=CARTESIAN_POINT('Ctrl Pts',(33.3740500633801,-7.89130690893979,-6.9197730813843));
#67893=CARTESIAN_POINT('Ctrl Pts',(33.4931141862293,-3.62022593454477,-9.85139322186365));
#67894=CARTESIAN_POINT('Ctrl Pts',(33.6121783090785,1.53282527671301,-10.3829875710222));
#67895=CARTESIAN_POINT('Ctrl Pts',(33.7312424319277,6.31244502352206,-8.38504752842475));
#67896=CARTESIAN_POINT('Ctrl Pts',(33.8503065547769,9.55420809142776,-4.34431720465111));
#67897=CARTESIAN_POINT('Ctrl Pts',(33.9693706776261,10.4683464956279,0.754788630283966));
#67898=CARTESIAN_POINT('Ctrl Pts',(34.0884348004753,8.83215511233873,5.67001060850159));
#67899=CARTESIAN_POINT('Ctrl Pts',(34.2074989233245,5.044247765107,9.20388769559607));
#67900=CARTESIAN_POINT('Ctrl Pts',(34.3265630461737,0.0274457365422501,
10.495486218393));
#67901=CARTESIAN_POINT('Ctrl Pts',(34.4456271690228,-4.99604270419572,9.23014309351612));
#67902=CARTESIAN_POINT('Ctrl Pts',(34.5646912918721,-8.80238032427643,5.71612498601302));
#67903=CARTESIAN_POINT('Ctrl Pts',(34.6837554147212,-10.4642558030642,0.809527465234853));
#67904=CARTESIAN_POINT('Ctrl Pts',(34.8028195375704,-9.57679808108244,-4.29428955045041));
#67905=CARTESIAN_POINT('Ctrl Pts',(34.9218836604196,-6.35621225475712,-8.35191894126176));
#67906=CARTESIAN_POINT('Ctrl Pts',(35.0409477832688,-1.58710704615101,-10.3748289360832));
#67907=CARTESIAN_POINT('Ctrl Pts',(35.160011906118,3.56865391342995,-9.87019217011967));
#67908=CARTESIAN_POINT('Ctrl Pts',(35.2790760289672,7.85500876570816,-6.96094975700724));
#67909=CARTESIAN_POINT('Ctrl Pts',(35.3981401518164,10.227702960638,-2.35586000812625));
#67910=CARTESIAN_POINT('Ctrl Pts',(35.5172042746655,10.1086936636169,2.82317138057241));
#67911=CARTESIAN_POINT('Ctrl Pts',(35.6362683975148,7.52697427444376,7.3144133394821));
#67912=CARTESIAN_POINT('Ctrl Pts',(35.755332520364,3.11151096880807,10.0236961107128));
#67913=CARTESIAN_POINT('Ctrl Pts',(35.8743966432131,-2.06198791686537,10.2909761470733));
#67914=CARTESIAN_POINT('Ctrl Pts',(35.9934607660623,-6.73313915785387,8.05113788913754));
#67915=CARTESIAN_POINT('Ctrl Pts',(36.1125248889115,-9.76394296051906,3.84985741199099));
#67916=CARTESIAN_POINT('Ctrl Pts',(36.2315890117607,-10.416025865289,-1.28933680726268));
#67917=CARTESIAN_POINT('Ctrl Pts',(36.3506531346099,-8.53052549054089,-6.11441894902236));
#67918=CARTESIAN_POINT('Ctrl Pts',(36.4697172574591,-4.56679305970356,-9.44988811461674));
#67919=CARTESIAN_POINT('Ctrl Pts',(36.5887813803082,0.509515113475162,-10.4831473603146));
#67920=CARTESIAN_POINT('Ctrl Pts',(36.7078455031575,5.46169369545109,-8.96247098773554));
#67921=CARTESIAN_POINT('Ctrl Pts',(36.8269096260067,9.08327817381496,-5.25833070907757));
#67922=CARTESIAN_POINT('Ctrl Pts',(36.9459737488559,10.4919673392078,-0.273140223929764));
#67923=CARTESIAN_POINT('Ctrl Pts',(37.0650378717051,9.34457213676633,4.77859349701376));
#67924=CARTESIAN_POINT('Ctrl Pts',(37.1841019945542,5.92062440698051,8.66615202153747));
#67925=CARTESIAN_POINT('Ctrl Pts',(37.3031661174034,1.05427650521303,10.4424367500831));
#67926=CARTESIAN_POINT('Ctrl Pts',(37.4222302402527,-4.06891738236679,9.67470390060619));
#67927=CARTESIAN_POINT('Ctrl Pts',(37.5412943631018,-8.20082948466987,6.54999083910055));
#67928=CARTESIAN_POINT('Ctrl Pts',(37.660358485951,-10.3348310549124,1.82954947879261));
#67929=CARTESIAN_POINT('Ctrl Pts',(37.7794226088002,-9.95103026744526,-3.33661218083857));
#67930=CARTESIAN_POINT('Ctrl Pts',(37.8984867316494,-7.14292981451776,-7.68989843195632));
#67931=CARTESIAN_POINT('Ctrl Pts',(38.0175508544986,-2.59464750158812,-10.1697486975556));
#67932=CARTESIAN_POINT('Ctrl Pts',(38.1366149773478,2.58575057232614,-10.1720144615826));
#67933=CARTESIAN_POINT('Ctrl Pts',(38.255679100197,7.13620038169131,-7.69614373184913));
#67934=CARTESIAN_POINT('Ctrl Pts',(38.3747432230462,9.948107775545,-3.34531551801509));
#67935=CARTESIAN_POINT('Ctrl Pts',(38.4938073458954,10.3364274901293,1.82050843728659));
#67936=CARTESIAN_POINT('Ctrl Pts',(38.6128714687446,8.20655591869616,6.54281469875498));
#67937=CARTESIAN_POINT('Ctrl Pts',(38.7319355915937,4.07737872427021,9.6711409341297));
#67938=CARTESIAN_POINT('Ctrl Pts',(38.8509997144429,-1.04514163277688,10.4433549779928));
#67939=CARTESIAN_POINT('Ctrl Pts',(38.9700638372921,-5.91304146887271,8.67132774241194));
#67940=CARTESIAN_POINT('Ctrl Pts',(39.0891279601413,-9.34038851097928,4.78676578630067));
#67941=CARTESIAN_POINT('Ctrl Pts',(39.2081920829905,-10.4922022531302,-0.263962323714354));
#67942=CARTESIAN_POINT('Ctrl Pts',(39.3272562058397,-9.0878743970168,-5.25038314535039));
#67943=CARTESIAN_POINT('Ctrl Pts',(39.4463203286889,-5.46953148233069,-8.9576899696698));
#67944=CARTESIAN_POINT('Ctrl Pts',(39.5653844515381,-0.518684999023309,
-10.4826976537873));
#67945=CARTESIAN_POINT('Ctrl Pts',(39.6844485743872,4.55852507034851,-9.45387927847339));
#67946=CARTESIAN_POINT('Ctrl Pts',(39.8035126972365,8.52517366959541,-6.12187864402225));
#67947=CARTESIAN_POINT('Ctrl Pts',(39.9225768200856,10.4148940393362,-1.29844768026914));
#67948=CARTESIAN_POINT('Ctrl Pts',(40.0416409429349,9.76730686835976,3.84131497903059));
#67949=CARTESIAN_POINT('Ctrl Pts',(40.160705065784,6.74017927425415,8.04524502920423));
#67950=CARTESIAN_POINT('Ctrl Pts',(40.2797691886333,2.07098910762834,10.2891684962916));
#67951=CARTESIAN_POINT('Ctrl Pts',(40.3988333114824,-3.10274160052417,10.0264140543247));
#67952=CARTESIAN_POINT('Ctrl Pts',(40.5178974343316,-7.52057314846527,7.32099472402093));
#67953=CARTESIAN_POINT('Ctrl Pts',(40.6369615571808,-10.1062202409998,2.83201282939607));
#67954=CARTESIAN_POINT('Ctrl Pts',(40.75602568003,-10.2297598246351,-2.34691247491805));
#67955=CARTESIAN_POINT('Ctrl Pts',(40.8750898028791,-7.86109481570529,-6.95407596456924));
#67956=CARTESIAN_POINT('Ctrl Pts',(40.9941539257284,-3.57728645024092,-9.86706673142152));
#67957=CARTESIAN_POINT('Ctrl Pts',(41.1132180485776,1.57803111163873,-10.376213281443));
#67958=CARTESIAN_POINT('Ctrl Pts',(41.2322821714268,6.34890401958871,-8.35747580919987));
#67959=CARTESIAN_POINT('Ctrl Pts',(41.351346294276,9.57303801703849,-4.30266516628609));
#67960=CARTESIAN_POINT('Ctrl Pts',(41.4704104171251,10.4649599138979,0.80037360570219));
#67961=CARTESIAN_POINT('Ctrl Pts',(41.5894745399744,8.80737713858352,5.70842295074491));
#67962=CARTESIAN_POINT('Ctrl Pts',(41.7085386628235,5.00411475535267,9.22576931894892));
#67963=CARTESIAN_POINT('Ctrl Pts',(41.8276027856728,-0.0182647388121033,
10.4955061722386));
#67964=CARTESIAN_POINT('Ctrl Pts',(41.9466669085219,-5.03619499973622,9.20829667944856));
#67965=CARTESIAN_POINT('Ctrl Pts',(42.0657310313711,-8.82719149690324,5.67773417809401));
#67966=CARTESIAN_POINT('Ctrl Pts',(42.1847951542203,-10.4676830601359,0.763945753984031));
#67967=CARTESIAN_POINT('Ctrl Pts',(42.3038592770695,-9.55800302737459,-4.33595858588686));
#67968=CARTESIAN_POINT('Ctrl Pts',(42.4229233999187,-6.31978043532264,-8.37952150001038));
#67969=CARTESIAN_POINT('Ctrl Pts',(42.5419875227679,-1.54190126780919,-10.3816447777769));
#67970=CARTESIAN_POINT('Ctrl Pts',(42.6610516456171,3.61159571846151,-9.85455234408739));
#67971=CARTESIAN_POINT('Ctrl Pts',(42.7801157684663,7.88527282360298,-6.92668081586803));
#67972=CARTESIAN_POINT('Ctrl Pts',(42.8991798913155,10.2378238462044,-2.31127910492416));
#67973=CARTESIAN_POINT('Ctrl Pts',(43.0182440141647,10.0963842416504,2.86714234294199));
#67974=CARTESIAN_POINT('Ctrl Pts',(43.1373081370138,7.49488795361275,7.34718010736619));
#67975=CARTESIAN_POINT('Ctrl Pts',(43.256372259863,3.06813757384479,10.0370448113317));
#67976=CARTESIAN_POINT('Ctrl Pts',(43.3754363827122,-2.10743535884606,10.2821305792463));
#67977=CARTESIAN_POINT('Ctrl Pts',(43.4548124646117,-5.21345574091479,8.7747535731645));
#67978=CARTESIAN_POINT('Ctrl Pts',(43.4945005055614,-6.49277053942583,7.69536373229664));
#67979=CARTESIAN_POINT('Origin',(8.,0.,0.));
#67980=CARTESIAN_POINT('',(9.5,0.,0.));
#67981=CARTESIAN_POINT('',(8.,-2.5,-3.06161699786838E-16));
#67982=CARTESIAN_POINT('Origin',(43.,11.3514471211877,-1.97095110413219));
#67983=CARTESIAN_POINT('Origin',(43.,10.5909347898596,-4.53564772407893));
#67984=CARTESIAN_POINT('Origin',(43.,9.25946242264882,-6.85582640121192));
#67985=CARTESIAN_POINT('Origin',(43.,7.42881003951057,-8.80640570249106));
#67986=CARTESIAN_POINT('Origin',(43.,5.19766858426649,-10.2822293928957));
#67987=CARTESIAN_POINT('Origin',(43.,2.68631947027824,-11.2037354352735));
#67988=CARTESIAN_POINT('Origin',(43.,0.0301501783194109,-11.5212452003569));
#67989=CARTESIAN_POINT('Origin',(43.,-2.6276445175567,-11.2176416545259));
#67990=CARTESIAN_POINT('Origin',(43.,-5.1437822173509,-10.309292143521));
#67991=CARTESIAN_POINT('Origin',(43.,-7.3826172863893,-8.84516602459817));
#67992=CARTESIAN_POINT('Origin',(43.,-9.22345354659921,-6.90419471580332));
#67993=CARTESIAN_POINT('Origin',(43.,-10.56705103871,-4.59101648279533));
#67994=CARTESIAN_POINT('Origin',(43.,-11.3409760741447,-2.03033536285951));
#67995=CARTESIAN_POINT('Origin',(43.,-11.50350615392,0.639801662020789));
#67996=CARTESIAN_POINT('Origin',(43.,-11.0458792393659,3.27544681369506));
#67997=CARTESIAN_POINT('Origin',(43.,-9.99276611589833,5.73451177982522));
#67998=CARTESIAN_POINT('Origin',(43.,-8.40094038459157,7.88442773158195));
#67999=CARTESIAN_POINT('Origin',(43.,-6.3562177826491,9.60929214352105));
#68000=CARTESIAN_POINT('Origin',(43.,-3.96882983479838,10.8161171287304));
#68001=CARTESIAN_POINT('Origin',(43.,-1.36748124326036,11.4398424398823));
#68002=CARTESIAN_POINT('Origin',(43.,1.30758861606115,11.4468428840072));
#68003=CARTESIAN_POINT('Origin',(43.,3.91216603463411,10.8367410653506));
#68004=CARTESIAN_POINT('Origin',(43.,6.30583756965351,9.64242773087495));
#68005=CARTESIAN_POINT('Origin',(43.,8.35955976908767,7.92828862157849));
#68006=CARTESIAN_POINT('Origin',(43.,9.96261593757892,5.7867334205317));
#68007=CARTESIAN_POINT('Origin',(43.,11.0285849021483,3.33321392294394));
#68008=CARTESIAN_POINT('Origin',(43.,11.5,0.7));
#68009=CARTESIAN_POINT('Origin',(133.079689783217,7.42462120245875,-12.8598211496117));
#68010=CARTESIAN_POINT('Origin',(133.079689783217,7.42462120245875,-12.8598211496117));
#68011=CARTESIAN_POINT('Origin',(155.,2.16262821021007E-15,-3.7457819379656E-15));
#68012=CARTESIAN_POINT('Origin',(158.5,0.,0.));
#68013=CARTESIAN_POINT('Origin',(133.079689783217,7.42462120245876,12.8598211496117));
#68014=CARTESIAN_POINT('Origin',(133.079689783217,14.8492424049175,-1.04365961982954E-15));
#68015=CARTESIAN_POINT('Origin',(21.9,0.,0.));
#90338=UNCERTAINTY_MEASURE_WITH_UNIT(LENGTH_MEASURE(0.01),#90375,
'DISTANCE_ACCURACY_VALUE',
'Maximum model space distance between geometric entities at asserted c
onnectivities');
#90355=UNCERTAINTY_MEASURE_WITH_UNIT(LENGTH_MEASURE(0.01),#90375,
'DISTANCE_ACCURACY_VALUE',
'Maximum model space distance between geometric entities at asserted c
onnectivities');
#90357=(
GEOMETRIC_REPRESENTATION_CONTEXT(3)
GLOBAL_UNCERTAINTY_ASSIGNED_CONTEXT((#90338))
GLOBAL_UNIT_ASSIGNED_CONTEXT((#90375,#90377,#90378))
REPRESENTATION_CONTEXT('','3D')
);
#90374=(
GEOMETRIC_REPRESENTATION_CONTEXT(3)
GLOBAL_UNCERTAINTY_ASSIGNED_CONTEXT((#90355))
GLOBAL_UNIT_ASSIGNED_CONTEXT((#90375,#90377,#90378))
REPRESENTATION_CONTEXT('','3D')
);
#90375=(
LENGTH_UNIT()
NAMED_UNIT(*)
SI_UNIT(.MILLI.,.METRE.)
);
#90377=(
NAMED_UNIT(*)
PLANE_ANGLE_UNIT()
SI_UNIT($,.RADIAN.)
);
#90378=(
NAMED_UNIT(*)
SI_UNIT($,.STERADIAN.)
SOLID_ANGLE_UNIT()
);
#90380=SHAPE_DEFINITION_REPRESENTATION(#90398,#90441);
#90398=PRODUCT_DEFINITION_SHAPE('',$,#90460);
#90441=SHAPE_REPRESENTATION('',(#40551),#90357);
#90458=PRODUCT_DEFINITION_CONTEXT('part definition',#90514,'design');
#90460=PRODUCT_DEFINITION('2026-10-11-12-53-07-348',
'01_Outer_CV_Bell_Housing_with_Stub',#90478,#90458);
#90478=PRODUCT_DEFINITION_FORMATION('',$,#90517);
#90514=APPLICATION_CONTEXT(
'Core Data for Automotive Mechanical Design Process');
#90515=PRODUCT_CONTEXT('part definition',#90514,'mechanical');
#90517=PRODUCT('2026-10-11-12-53-07-348',
'01_Outer_CV_Bell_Housing_with_Stub',$,(#90515));
#90660=COLOUR_RGB('Dark Blue',0.08,0.2,0.34);
#90661=FILL_AREA_STYLE_COLOUR('',#90660);
#90662=FILL_AREA_STYLE('',(#90661));
#90663=SURFACE_STYLE_FILL_AREA(#90662);
#90664=SURFACE_SIDE_STYLE('',(#90663));
#90665=SURFACE_STYLE_USAGE(.BOTH.,#90664);
#90666=PRESENTATION_STYLE_ASSIGNMENT((#90665));
ENDSEC;
END-ISO-10303-21;
